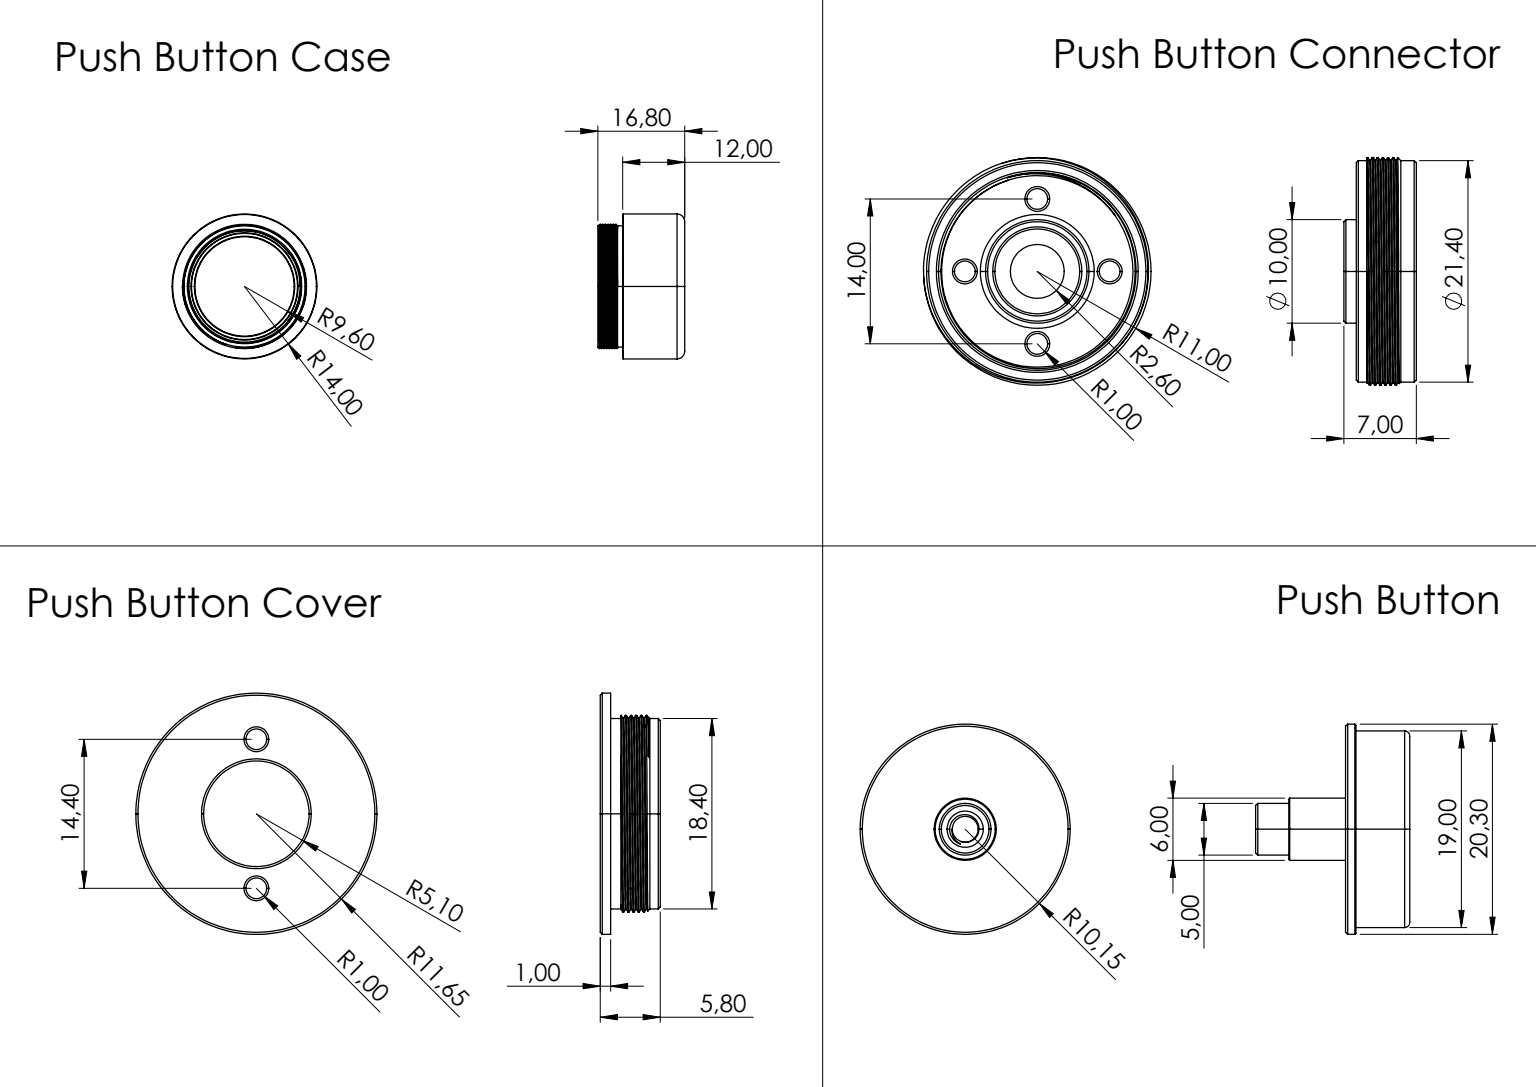
ISO-10303-21;
HEADER;
FILE_DESCRIPTION (('STEP AP214'),
    '1' );
FILE_NAME ('Push Button Case.step',
    '2026-10-07T19:06:49',
    ( '' ),
    ( '' ),
    'SwSTEP 2.0',
    'SolidWorks 2020',
    '' );
FILE_SCHEMA (( 'AUTOMOTIVE_DESIGN' ));
ENDSEC;

DATA;
#16=CARTESIAN_POINT ( 'NONE',  ( 3.109033293168000256, -77.33638120859698972, -11.95479571607999958 ) ) ;
#23=CARTESIAN_POINT ( 'NONE',  ( -2.309466437478999712, -77.64150279751002870, 10.97654204954999990 ) ) ;
#32=AXIS2_PLACEMENT_3D ( 'NONE', #6356, #50954, #38231 ) ;
#33=ADVANCED_FACE ( 'NONE', ( #3684 ), #39982, .F. ) ;
#37=AXIS2_PLACEMENT_3D ( 'NONE', #47276, #15952, #33942 ) ;
#39=CARTESIAN_POINT ( 'NONE',  ( -6.620362748380999918, -76.28137637478999977, -10.34376132320999986 ) ) ;
#46=CARTESIAN_POINT ( 'NONE',  ( 2.813789756862229652, -77.85416666666665719, 10.47020627418440064 ) ) ;
#50=CARTESIAN_POINT ( 'NONE',  ( -10.20076187689604374, -79.12621043184928737, -3.463739626987611064 ) ) ;
#55=CARTESIAN_POINT ( 'NONE',  ( -11.91766194687999914, -78.07234609596400787, 0.6362673702790999641 ) ) ;
#59=CARTESIAN_POINT ( 'NONE',  ( 7.698699457163000304, -79.83930274324279708, 7.739857405570000459 ) ) ;
#68=CARTESIAN_POINT ( 'NONE',  ( 1.570796326794856590, -77.76458333333333428, 12.00000000000000711 ) ) ;
#72=CARTESIAN_POINT ( 'NONE',  ( 6.724228645090999379, -79.38539396382098801, -8.890407735272999545 ) ) ;
#80=ADVANCED_FACE ( 'NONE', ( #13408 ), #31504, .F. ) ;
#87=DIRECTION ( 'NONE',  ( 0.000000000000000000, 1.000000000000000000, 0.000000000000000000 ) ) ;
#96=ORIENTED_EDGE ( 'NONE', *, *, #34117, .T. ) ;
#98=CARTESIAN_POINT ( 'NONE',  ( 6.225574660483999878, -77.96842036916400787, 9.107357164861998200 ) ) ;
#102=CARTESIAN_POINT ( 'NONE',  ( 10.54265532893000135, -78.47604828264000787, 3.830212845596999927 ) ) ;
#103=CARTESIAN_POINT ( 'NONE',  ( 10.87736683009447525, -81.00000000000001421, 1.725104219249947057 ) ) ;
#104=EDGE_LOOP ( 'NONE', ( #8306, #56264, #8122, #44410 ) ) ;
#119=CARTESIAN_POINT ( 'NONE',  ( -10.96659098533000076, -79.41245439073298940, -5.858662427812999951 ) ) ;
#121=CARTESIAN_POINT ( 'NONE',  ( 2.970805461283999804, -76.56305898269899046, 11.10324980701000008 ) ) ;
#122=CARTESIAN_POINT ( 'NONE',  ( -5.476929600924019148, -78.01766025678556105, 9.250714535254271453 ) ) ;
#123=CARTESIAN_POINT ( 'NONE',  ( -4.085659785884999451, -78.53658950733898791, 11.26159174134999930 ) ) ;
#129=CARTESIAN_POINT ( 'NONE',  ( 4.095273378172390899, -80.94411864974023274, 9.939233580224922093 ) ) ;
#132=CARTESIAN_POINT ( 'NONE',  ( 8.145565103785999739, -77.70092985212998826, 7.609492079688000565 ) ) ;
#133=CARTESIAN_POINT ( 'NONE',  ( 11.68767212001977995, -78.07083333333333997, 3.140974612311385972 ) ) ;
#134=CARTESIAN_POINT ( 'NONE',  ( -1.803444444386999912, -80.27907522661350015, 10.99384993464000004 ) ) ;
#140=CARTESIAN_POINT ( 'NONE',  ( 0.2654799511899000319, -78.39298939775198960, -11.21373274707999990 ) ) ;
#150=CARTESIAN_POINT ( 'NONE',  ( 0.1384068119873999858, -77.08287542851299179, 11.14609546546000018 ) ) ;
#159=CARTESIAN_POINT ( 'NONE',  ( 10.58961540942159729, -78.57316667069575544, -3.698874623828772634 ) ) ;
#164=CARTESIAN_POINT ( 'NONE',  ( -0.4120475804594999625, -79.51319421340399174, -11.13933648663000042 ) ) ;
#183=CARTESIAN_POINT ( 'NONE',  ( 4.145485675599949182, -78.25643109645689321, -9.984513293680489454 ) ) ;
#185=VERTEX_POINT ( 'NONE', #55030 ) ;
#196=CARTESIAN_POINT ( 'NONE',  ( -7.859650249856000137, -76.58738468523199572, -7.529696512734999736 ) ) ;
#197=CARTESIAN_POINT ( 'NONE',  ( 12.00000000000000000, -78.14999999999999147, 0.000000000000000000 ) ) ;
#200=CARTESIAN_POINT ( 'NONE',  ( -11.26045488449999965, -80.83153675553073469, 0.3336940576009999604 ) ) ;
#207=CARTESIAN_POINT ( 'NONE',  ( 8.440675369999999234, -80.13928997744719140, 7.053722371789000967 ) ) ;
#219=ORIENTED_EDGE ( 'NONE', *, *, #4233, .T. ) ;
#230=CARTESIAN_POINT ( 'NONE',  ( 0.2080084001491119827, -77.22664242507777033, -10.74806830262927981 ) ) ;
#238=CARTESIAN_POINT ( 'NONE',  ( -0.7898276719169999849, -78.74313915747200099, -11.90847071177000061 ) ) ;
#242=CARTESIAN_POINT ( 'NONE',  ( 9.597438627498371844, -76.59723940367341299, -7.375897342311914073 ) ) ;
#263=CARTESIAN_POINT ( 'NONE',  ( -1.879551087701830880, -76.29218749999812133, 11.88134584529343485 ) ) ;
#275=CARTESIAN_POINT ( 'NONE',  ( 2.269106295766999856E-14, -92.56607767729998670, -10.93038838648999977 ) ) ;
#277=CARTESIAN_POINT ( 'NONE',  ( 5.013494814495999208, -77.86362032395699373, 9.697434492446999954 ) ) ;
#278=CARTESIAN_POINT ( 'NONE',  ( 12.18149635271999820, -78.11332874153899297, -1.551427017228999894 ) ) ;
#286=CARTESIAN_POINT ( 'NONE',  ( -4.648821459404000045, -81.05100055871760389, 9.896537447400001852 ) ) ;
#289=CARTESIAN_POINT ( 'NONE',  ( 7.508079800428999917, -77.01725177193199556, -8.333477563431999968 ) ) ;
#305=ORIENTED_EDGE ( 'NONE', *, *, #4247, .T. ) ;
#307=ORIENTED_EDGE ( 'NONE', *, *, #4039, .F. ) ;
#314=CARTESIAN_POINT ( 'NONE',  ( 1.293235748077000036, -76.48998211639099054, 12.16612483867000094 ) ) ;
#315=CARTESIAN_POINT ( 'NONE',  ( -10.47027344149396377, -78.61824586144523153, -2.436629557234976762 ) ) ;
#321=CARTESIAN_POINT ( 'NONE',  ( -1.570796326794885012, -78.91458333333333997, -12.00000000000000178 ) ) ;
#334=DIRECTION ( 'NONE',  ( 0.000000000000000000, 1.000000000000000000, 1.686839199259000058E-13 ) ) ;
#335=ADVANCED_FACE ( 'NONE', ( #15362 ), #37204, .T. ) ;
#341=ORIENTED_EDGE ( 'NONE', *, *, #14163, .T. ) ;
#351=CARTESIAN_POINT ( 'NONE',  ( -1.612912635236000147, -78.84554001676799828, 10.91330597072999886 ) ) ;
#353=VERTEX_POINT ( 'NONE', #51103 ) ;
#360=CARTESIAN_POINT ( 'NONE',  ( -3.140974612311405512, -77.79583333333334849, 11.68767212001977640 ) ) ;
#364=CARTESIAN_POINT ( 'NONE',  ( -9.018305195942000196, -79.72548445825199792, 6.745675351750000104 ) ) ;
#374=CARTESIAN_POINT ( 'NONE',  ( -5.413904038987206846, -78.41666666666665719, 9.393203674808249914 ) ) ;
#381=CARTESIAN_POINT ( 'NONE',  ( -3.140974612311405512, -79.69583333333332575, 11.68767212001977640 ) ) ;
#382=EDGE_LOOP ( 'NONE', ( #44129, #54601, #18071, #20029, #55022, #27124, #7591, #40469, #14418, #38243, #20068 ) ) ;
#383=CARTESIAN_POINT ( 'NONE',  ( 8.628867348358941314, -76.05332450398152844, 6.837351357443815836 ) ) ;
#386=AXIS2_PLACEMENT_3D ( 'NONE', #45632, #45042, #41184 ) ;
#387=CARTESIAN_POINT ( 'NONE',  ( 11.00720109383000000, -77.39645716612599813, 0.7370606905150999255 ) ) ;
#391=CARTESIAN_POINT ( 'NONE',  ( 1.099819419251000019, -79.63329055598900652, 11.16281809564999961 ) ) ;
#411=CARTESIAN_POINT ( 'NONE',  ( -12.01465389393999850, -78.95880199243299558, -2.711845028153999859 ) ) ;
#412=CARTESIAN_POINT ( 'NONE',  ( -10.26547038271000112, -76.61176894222799660, 3.946724975948999958 ) ) ;
#413=CARTESIAN_POINT ( 'NONE',  ( -6.822290318485905836, -78.02980255133013543, 8.307683877974495701 ) ) ;
#414=CARTESIAN_POINT ( 'NONE',  ( 8.770451247185000909, -78.94352923869598726, 8.160602927202999624 ) ) ;
#419=CARTESIAN_POINT ( 'NONE',  ( 6.307978547608708020, -80.92535043715515997, 8.704505370279399301 ) ) ;
#421=DIRECTION ( 'NONE',  ( -0.7071067811864976127, 0.7071067811865975328, -1.591673720108993631E-09 ) ) ;
#422=CARTESIAN_POINT ( 'NONE',  ( -10.52129323452999898, -77.86434791014099233, 3.681981700656000278 ) ) ;
#424=CARTESIAN_POINT ( 'NONE',  ( -11.00676540241999923, -80.45419303504098707, 0.6467430135644000044 ) ) ;
#431=CARTESIAN_POINT ( 'NONE',  ( 9.070694317316998934, -77.99836472845399271, 6.598531290616000078 ) ) ;
#436=CARTESIAN_POINT ( 'NONE',  ( -10.65295200446612967, -78.51231955895573833, -1.664190318615639042 ) ) ;
#439=CARTESIAN_POINT ( 'NONE',  ( -4.801183948719927486, -76.05000000000001137, 10.79468190462868016 ) ) ;
#441=CARTESIAN_POINT ( 'NONE',  ( -3.610459473067000324, -77.11011177151499396, 10.54605058607999979 ) ) ;
#447=CARTESIAN_POINT ( 'NONE',  ( -7.579570500035162972, -80.16319179611589618, -7.622759937838323729 ) ) ;
#451=DIRECTION ( 'NONE',  ( 0.000000000000000000, 1.000000000000000000, 0.000000000000000000 ) ) ;
#452=CARTESIAN_POINT ( 'NONE',  ( 0.9518616847512999524, -79.02294003937198852, -11.10623968335000100 ) ) ;
#472=CARTESIAN_POINT ( 'NONE',  ( 10.75000000000000000, -78.25000000000000000, 1.005550720961999908E-14 ) ) ;
#483=CARTESIAN_POINT ( 'NONE',  ( 9.755626371838998168, -80.97443200427989041, -5.633583086437000453 ) ) ;
#489=CARTESIAN_POINT ( 'NONE',  ( 7.551392188974999975, -80.21711109272469287, 8.117862728809001283 ) ) ;
#493=CARTESIAN_POINT ( 'NONE',  ( -10.75000000000000000, -80.00000000000000000, 0.000000000000000000 ) ) ;
#502=CARTESIAN_POINT ( 'NONE',  ( -6.340838181001343443, -79.52523374718921900, 8.680779125499762827 ) ) ;
#516=CARTESIAN_POINT ( 'NONE',  ( 0.01050698433460529012, -77.22515890467916222, -10.74994752102681339 ) ) ;
#520=ORIENTED_EDGE ( 'NONE', *, *, #57168, .F. ) ;
#524=CARTESIAN_POINT ( 'NONE',  ( 6.436424241555000592, -80.32391735373440156, 8.610165096135999008 ) ) ;
#526=CARTESIAN_POINT ( 'NONE',  ( 11.27339212957999948, -77.96985744374799765, 4.255161755617000274 ) ) ;
#533=FACE_OUTER_BOUND ( 'NONE', #5641, .T. ) ;
#534=CIRCLE ( 'NONE', #25023, 12.09999999999999964 ) ;
#543=CARTESIAN_POINT ( 'NONE',  ( -11.08400893143999966, -76.20894737471998326, -1.489506537590000068 ) ) ;
#546=CARTESIAN_POINT ( 'NONE',  ( -11.92766985523999956, -77.65742819841213418, -1.116582401450000095 ) ) ;
#548=CARTESIAN_POINT ( 'NONE',  ( -6.660059710594288696, -76.92432036743132073, -9.025807911732075084 ) ) ;
#562=CARTESIAN_POINT ( 'NONE',  ( -0.2428088493965334382, -78.22329368912637904, -10.77973457647781785 ) ) ;
#563=EDGE_CURVE ( 'NONE', #20195, #7399, #29212, .T. ) ;
#569=CARTESIAN_POINT ( 'NONE',  ( 1.764045786578000152, -77.01006991430598703, -11.99279291753999921 ) ) ;
#578=CARTESIAN_POINT ( 'NONE',  ( -7.249076177254000442, -80.50531345225510904, 8.347662706485998285 ) ) ;
#579=CARTESIAN_POINT ( 'NONE',  ( -9.599999999999999645, -90.39999999999999147, 0.000000000000000000 ) ) ;
#581=CYLINDRICAL_SURFACE ( 'NONE', #57781, 12.00000000000000000 ) ;
#610=CARTESIAN_POINT ( 'NONE',  ( -10.75000000000000000, -76.50000000000000000, 0.000000000000000000 ) ) ;
#616=VERTEX_POINT ( 'NONE', #44246 ) ;
#624=CARTESIAN_POINT ( 'NONE',  ( 2.548493721447000038, -77.06004840258400179, 12.01365081398999912 ) ) ;
#635=CARTESIAN_POINT ( 'NONE',  ( 11.20799393363000007, -77.77703814603999888, 4.230477091134000389 ) ) ;
#637=CARTESIAN_POINT ( 'NONE',  ( 4.928445265185000146, -78.16739492409399759, -10.99573548889999941 ) ) ;
#640=CARTESIAN_POINT ( 'NONE',  ( -10.57985553746999940, -78.98172173177698596, -3.125442558719000008 ) ) ;
#642=ORIENTED_EDGE ( 'NONE', *, *, #17291, .F. ) ;
#646=CARTESIAN_POINT ( 'NONE',  ( -14.00000000000000000, -80.89999999999999147, 0.000000000000000000 ) ) ;
#647=CARTESIAN_POINT ( 'NONE',  ( -7.374560639699019760, -77.82708333333329165, 9.596002108778129980 ) ) ;
#652=CARTESIAN_POINT ( 'NONE',  ( 10.16136252780999882, -79.56206640024099386, 4.855993836148999598 ) ) ;
#654=CARTESIAN_POINT ( 'NONE',  ( 9.393203674808260573, -79.79166666666665719, 5.413904038987188194 ) ) ;
#671=CARTESIAN_POINT ( 'NONE',  ( 7.605248831740031967, -78.78754124960966010, -7.597529869121465218 ) ) ;
#672=CARTESIAN_POINT ( 'NONE',  ( -12.00000000000000000, -79.79999999999999716, 6.639246269807000381E-13 ) ) ;
#679=CARTESIAN_POINT ( 'NONE',  ( -6.549634241348975650, -76.96947804690607597, 10.29244451497932467 ) ) ;
#680=CARTESIAN_POINT ( 'NONE',  ( 6.917883603915965907, -78.72389193389439299, -9.780740130690492862 ) ) ;
#681=CARTESIAN_POINT ( 'NONE',  ( 10.93160348586000019, -79.03409100994899461, 2.513594203403000105 ) ) ;
#682=CARTESIAN_POINT ( 'NONE',  ( 10.14177821597014173, -81.00000000000002842, 4.213176577505078235 ) ) ;
#692=CARTESIAN_POINT ( 'NONE',  ( -10.75000000000000000, -81.00000000000000000, 2.851355842494999902E-13 ) ) ;
#694=DIRECTION ( 'NONE',  ( 0.000000000000000000, -1.000000000000000000, 0.000000000000000000 ) ) ;
#700=CARTESIAN_POINT ( 'NONE',  ( -12.29903597714999997, -79.44542282429898705, -0.6631160193374000533 ) ) ;
#701=CARTESIAN_POINT ( 'NONE',  ( -3.222839321634999976, -76.53899580226399735, 10.90918487679000037 ) ) ;
#702=CARTESIAN_POINT ( 'NONE',  ( 1.078297123321654505, -77.96723831660007420, 10.71709050783147710 ) ) ;
#703=CARTESIAN_POINT ( 'NONE',  ( -8.885616033064000163, -78.07539114513500067, 8.035041515002001589 ) ) ;
#706=AXIS2_PLACEMENT_3D ( 'NONE', #56290, #17001, #47739 ) ;
#709=CARTESIAN_POINT ( 'NONE',  ( 8.032001238464035353, -80.90813382219710093, 7.145123807818250405 ) ) ;
#712=CARTESIAN_POINT ( 'NONE',  ( -11.10013370946000144, -76.88383956207499637, 1.020686637641000205 ) ) ;
#713=CARTESIAN_POINT ( 'NONE',  ( -0.6669403506045999963, -76.27067270026404344, -12.26286337364000012 ) ) ;
#718=CARTESIAN_POINT ( 'NONE',  ( 1.633411169670999863, -77.83494667044399762, -11.09730050697999992 ) ) ;
#740=CARTESIAN_POINT ( 'NONE',  ( -0.2300833467695000134, -78.44680123892500490, -11.11357981391999949 ) ) ;
#744=EDGE_CURVE ( 'NONE', #35616, #18221, #56482, .T. ) ;
#754=CARTESIAN_POINT ( 'NONE',  ( 10.75000000000000355, -78.23958333333330017, -1.407171709420407035 ) ) ;
#756=EDGE_CURVE ( 'NONE', #5144, #34885, #31774, .T. ) ;
#758=ORIENTED_EDGE ( 'NONE', *, *, #11996, .T. ) ;
#772=CARTESIAN_POINT ( 'NONE',  ( -9.578166812159000898, -80.15420130091290218, 5.930253639820000089 ) ) ;
#775=CARTESIAN_POINT ( 'NONE',  ( 9.494399870356199145, -76.17369791634894227, -7.297544775540704798 ) ) ;
#786=CARTESIAN_POINT ( 'NONE',  ( -9.038474301085981821, -79.55454762255861567, 5.819977710880431587 ) ) ;
#801=CARTESIAN_POINT ( 'NONE',  ( -6.221842943951165772, -77.17604202210270614, -8.766351684138484757 ) ) ;
#811=CARTESIAN_POINT ( 'NONE',  ( 7.527227981725999939, -78.51244375222299254, 9.409389490551998136 ) ) ;
#816=CARTESIAN_POINT ( 'NONE',  ( -11.68619273497913014, -76.42035715448702149, -3.140303762288782163 ) ) ;
#823=CARTESIAN_POINT ( 'NONE',  ( 0.000000000000000000, -76.00000000000000000, 0.000000000000000000 ) ) ;
#828=CONICAL_SURFACE ( 'NONE', #33783, 10.96250000000000036, 0.7853981633972997312 ) ;
#829=CARTESIAN_POINT ( 'NONE',  ( -4.800187936532999800, -76.10861960676400884, 10.10109298474000106 ) ) ;
#830=CARTESIAN_POINT ( 'NONE',  ( 0.000000000000000000, -92.79999999999999716, 0.000000000000000000 ) ) ;
#846=CARTESIAN_POINT ( 'NONE',  ( 2.264809212410999647E-14, -92.79999999999999716, 0.000000000000000000 ) ) ;
#852=CARTESIAN_POINT ( 'NONE',  ( 11.48873525783000105, -77.65213037933499152, 4.336443399433000501 ) ) ;
#860=CARTESIAN_POINT ( 'NONE',  ( -6.095058532100999571, -81.19811224954469253, 9.210169058603000281 ) ) ;
#865=CARTESIAN_POINT ( 'NONE',  ( 11.75000000000000000, -79.80000000000002558, -1.240340237986687466 ) ) ;
#877=CARTESIAN_POINT ( 'NONE',  ( 11.26957934775000147, -79.10909624325299205, 4.877733875464000057 ) ) ;
#885=ORIENTED_EDGE ( 'NONE', *, *, #57938, .F. ) ;
#886=CARTESIAN_POINT ( 'NONE',  ( 5.438910196678000020, -76.28506842486599737, -10.95925680354000065 ) ) ;
#909=FACE_OUTER_BOUND ( 'NONE', #1382, .T. ) ;
#914=CARTESIAN_POINT ( 'NONE',  ( -2.848564863371000122, -78.85456761274453186, -10.84913769894000168 ) ) ;
#918=DIRECTION ( 'NONE',  ( 1.558073931336000057E-11, -1.000000000000000000, 1.336740861260999965E-10 ) ) ;
#919=CIRCLE ( 'NONE', #14073, 10.25000000000000000 ) ;
#924=CARTESIAN_POINT ( 'NONE',  ( -4.771559678803999560, -78.60146397087400771, -11.06471824780000013 ) ) ;
#927=CARTESIAN_POINT ( 'NONE',  ( 10.41480047653000085, -78.68212195875699422, -3.637813056042999982 ) ) ;
#939=CARTESIAN_POINT ( 'NONE',  ( -3.994755123096000560, -79.11303053380299843, 10.40656197200999955 ) ) ;
#941=CARTESIAN_POINT ( 'NONE',  ( -3.037998163973060883, -79.44541822414515764, 11.43917581953734697 ) ) ;
#957=CARTESIAN_POINT ( 'NONE',  ( 7.478737840490471633, -78.78621029007136656, -7.724116019082565288 ) ) ;
#958=CIRCLE ( 'NONE', #32, 10.25000000000000000 ) ;
#965=CARTESIAN_POINT ( 'NONE',  ( -9.690759288037638086, -78.09991767914834782, -7.043378150385348313 ) ) ;
#966=CARTESIAN_POINT ( 'NONE',  ( 2.407803015296000382, -80.19133328329790800, 10.73324203768999929 ) ) ;
#967=CARTESIAN_POINT ( 'NONE',  ( 4.500641208133613347, -81.00000000000001421, 9.880214559888472081 ) ) ;
#968=ORIENTED_EDGE ( 'NONE', *, *, #8365, .F. ) ;
#973=CARTESIAN_POINT ( 'NONE',  ( 9.576266942756152645, -76.04999999999998295, 5.533717098124343536 ) ) ;
#977=CARTESIAN_POINT ( 'NONE',  ( 1.570796326794910547, -78.53541666666664867, -11.99999999999999822 ) ) ;
#987=CARTESIAN_POINT ( 'NONE',  ( -8.615867236575999399, -76.71811381506900318, 7.785367480540000606 ) ) ;
#989=CARTESIAN_POINT ( 'NONE',  ( -11.86109855473999986, -78.57731821575799813, -1.682380905046999997 ) ) ;
#993=CARTESIAN_POINT ( 'NONE',  ( 1.544981608555010544, -80.96391980284444401, 10.63828215852447023 ) ) ;
#996=CARTESIAN_POINT ( 'NONE',  ( 10.69210609810000001, -78.16394768316000352, 3.151740433137000252 ) ) ;
#998=CARTESIAN_POINT ( 'NONE',  ( 8.209261416751999718, -80.19853216860269640, 7.218337095169999884 ) ) ;
#1003=CARTESIAN_POINT ( 'NONE',  ( -6.984027423104000043, -77.12680175239600544, 8.777327129872999123 ) ) ;
#1014=EDGE_CURVE ( 'NONE', #4724, #21904, #41618, .T. ) ;
#1017=CARTESIAN_POINT ( 'NONE',  ( 8.229676506584999274, -77.58638398095499156, 7.688067972860000765 ) ) ;
#1020=CARTESIAN_POINT ( 'NONE',  ( -9.596002108778161954, -79.35208333333332575, -7.374560639698982456 ) ) ;
#1023=CARTESIAN_POINT ( 'NONE',  ( -5.970525758963701080, -80.17821961223123139, -8.939477884329102508 ) ) ;
#1028=CARTESIAN_POINT ( 'NONE',  ( -10.27879708628000088, -78.85952198136099867, 4.312879667924000238 ) ) ;
#1042=VERTEX_POINT ( 'NONE', #55012 ) ;
#1056=CARTESIAN_POINT ( 'NONE',  ( 11.02326530841000007, -81.02459481428599020, 1.187788371667000131 ) ) ;
#1058=CYLINDRICAL_SURFACE ( 'NONE', #386, 12.00000000000000000 ) ;
#1059=CARTESIAN_POINT ( 'NONE',  ( 3.098607378237295595, -76.14114583267888747, -11.53327867144136043 ) ) ;
#1070=FACE_BOUND ( 'NONE', #30736, .T. ) ;
#1074=CARTESIAN_POINT ( 'NONE',  ( 7.189755216797094839, -79.41669502080303289, 7.992951545765084376 ) ) ;
#1086=CARTESIAN_POINT ( 'NONE',  ( 12.00000000000000000, -76.64999999999999147, 0.000000000000000000 ) ) ;
#1089=CARTESIAN_POINT ( 'NONE',  ( -10.75033332359620708, -77.11068282368783855, -1.411355356088692670 ) ) ;
#1095=CARTESIAN_POINT ( 'NONE',  ( 6.536979956083999177, -79.30461158636299501, -10.09826910480999906 ) ) ;
#1097=DIRECTION ( 'NONE',  ( 0.000000000000000000, -1.000000000000000000, 0.000000000000000000 ) ) ;
#1099=CARTESIAN_POINT ( 'NONE',  ( 11.66178877871000097, -78.39045805696299851, 2.537357863477000208 ) ) ;
#1110=CARTESIAN_POINT ( 'NONE',  ( -10.75000000000000000, -80.50000000000000000, -1.711887504597999906E-14 ) ) ;
#1114=CARTESIAN_POINT ( 'NONE',  ( 9.776276929627000456, -75.90796407085099418, -5.431214116490000521 ) ) ;
#1145=CARTESIAN_POINT ( 'NONE',  ( -10.20620196243999978, -80.81341270350478112, -5.091275341613999750 ) ) ;
#1150=CARTESIAN_POINT ( 'NONE',  ( 10.79417609527999922, -77.62976718524500086, -3.050225076229999832 ) ) ;
#1155=CARTESIAN_POINT ( 'NONE',  ( 1.147008568205678536, -76.09166666666237688, 10.95833333328629067 ) ) ;
#1156=ORIENTED_EDGE ( 'NONE', *, *, #53762, .F. ) ;
#1159=CARTESIAN_POINT ( 'NONE',  ( 0.000000000000000000, -87.64999999984398471, 0.000000000000000000 ) ) ;
#1164=CARTESIAN_POINT ( 'NONE',  ( 2.263099670254000273, -78.11897245443199722, 11.95244370277000101 ) ) ;
#1173=VERTEX_POINT ( 'NONE', #7578 ) ;
#1175=CARTESIAN_POINT ( 'NONE',  ( 8.586577278446998918, -79.87637572403669139, 6.741381070085999738 ) ) ;
#1182=CARTESIAN_POINT ( 'NONE',  ( -10.31421052434999908, -76.72175206120299151, 3.823226550887000030 ) ) ;
#1188=CARTESIAN_POINT ( 'NONE',  ( -10.75000000000000000, -77.51041666666665719, -1.407171709420429018 ) ) ;
#1193=CARTESIAN_POINT ( 'NONE',  ( 10.16964605767000052, -76.26874748315199781, -6.884832982024000181 ) ) ;
#1197=CARTESIAN_POINT ( 'NONE',  ( -6.324515969367999979, -78.82733126974268600, -9.263833350438000380 ) ) ;
#1206=CARTESIAN_POINT ( 'NONE',  ( 10.75624577990000041, -78.22165355494099970, -5.431293436759999871 ) ) ;
#1219=CARTESIAN_POINT ( 'NONE',  ( 6.758989304250999197, -77.04505930305400341, -10.14916591256000089 ) ) ;
#1226=CARTESIAN_POINT ( 'NONE',  ( -11.77076513002849012, -79.55082450634814961, -0.1443961957164959509 ) ) ;
#1235=CARTESIAN_POINT ( 'NONE',  ( 9.393203674808260573, -79.29166666666665719, 5.413904038987188194 ) ) ;
#1241=CARTESIAN_POINT ( 'NONE',  ( 6.122270975308672369, -78.77338805014832701, -8.836258741097333669 ) ) ;
#1247=EDGE_CURVE ( 'NONE', #50686, #10829, #57163, .T. ) ;
#1250=CARTESIAN_POINT ( 'NONE',  ( 8.049776716670494991, -77.23386658315779130, -8.806146062382781636 ) ) ;
#1252=CARTESIAN_POINT ( 'NONE',  ( -7.301194973305000779, -79.19750906795999867, 8.515319286630999684 ) ) ;
#1269=ORIENTED_EDGE ( 'NONE', *, *, #11855, .T. ) ;
#1270=CARTESIAN_POINT ( 'NONE',  ( -3.140974612311352221, -79.50416666666664867, -11.68767212001979061 ) ) ;
#1272=CARTESIAN_POINT ( 'NONE',  ( 3.165837231865861856, -77.95154321140272202, 10.30965284180923724 ) ) ;
#1276=CARTESIAN_POINT ( 'NONE',  ( 10.45256899451774757, -80.86916725350319268, 2.510129016786621925 ) ) ;
#1279=CARTESIAN_POINT ( 'NONE',  ( -3.573177736666999671, -77.36011177151499396, 10.43715168250999881 ) ) ;
#1280=CARTESIAN_POINT ( 'NONE',  ( 2.548493721447000038, -77.00836198975264324, 12.01365081398999912 ) ) ;
#1281=CARTESIAN_POINT ( 'NONE',  ( -6.382578252665999763, -80.53473609305189029, -8.990542599477999275 ) ) ;
#1282=ORIENTED_EDGE ( 'NONE', *, *, #26492, .F. ) ;
#1285=CARTESIAN_POINT ( 'NONE',  ( -7.712695008784000272, -77.26298346740499312, -8.144473358846001432 ) ) ;
#1300=CARTESIAN_POINT ( 'NONE',  ( -7.374560639698971798, -79.37291666666664014, -9.596002108778163731 ) ) ;
#1303=CARTESIAN_POINT ( 'NONE',  ( -7.600460745173878152, -80.16297109611984695, -7.601925197388003319 ) ) ;
#1307=ORIENTED_EDGE ( 'NONE', *, *, #22440, .T. ) ;
#1311=CARTESIAN_POINT ( 'NONE',  ( -5.305451056584999492, -80.04393910884809316, -9.672327717035999584 ) ) ;
#1334=CARTESIAN_POINT ( 'NONE',  ( -12.00000000000000000, -76.89999999999999147, 0.000000000000000000 ) ) ;
#1342=CARTESIAN_POINT ( 'NONE',  ( 8.440675369999999234, -80.07150142417098948, 7.053722371789000967 ) ) ;
#1343=LINE ( 'NONE', #46804, #52543 ) ;
#1344=CARTESIAN_POINT ( 'NONE',  ( 5.413936244485441307, -76.76681587759365755, -9.393431973814015734 ) ) ;
#1356=CARTESIAN_POINT ( 'NONE',  ( 10.07201971379686967, -79.37863564844947462, 3.781752685250035828 ) ) ;
#1369=CARTESIAN_POINT ( 'NONE',  ( -6.271765859646529329, -77.17558322877896160, -8.730771744879000096 ) ) ;
#1371=ADVANCED_FACE ( 'NONE', ( #22609 ), #37635, .F. ) ;
#1374=CARTESIAN_POINT ( 'NONE',  ( 2.377756013412999803, -79.34251650879200213, -11.79209151100000064 ) ) ;
#1379=B_SPLINE_CURVE_WITH_KNOTS ( 'NONE', 3,
 ( #54929, #32472, #36631, #36336, #46687, #49939, #54361, #10071, #37209, #28052, #41359, #5340, #36918, #27471, #654, #51107, #41940, #10659 ),
 .UNSPECIFIED., .F., .F.,
 ( 4, 2, 2, 2, 2, 2, 2, 2, 4 ),
 ( 0.000000000000000000, 0.1250000000000000000, 0.2500000000000000000, 0.3750000000000000000, 0.5000000000000000000, 0.6250000000000000000, 0.7500000000000000000, 0.8750000000000000000, 1.000000000000000000 ),
 .UNSPECIFIED. ) ;
#1380=CARTESIAN_POINT ( 'NONE',  ( 10.65351345285000129, -78.33619942611500164, -5.379419444189999844 ) ) ;
#1382=EDGE_LOOP ( 'NONE', ( #1591, #17664, #4339, #1641 ) ) ;
#1393=CARTESIAN_POINT ( 'NONE',  ( -10.75000000000000000, -80.51041666666664298, -1.407171709420429018 ) ) ;
#1395=CARTESIAN_POINT ( 'NONE',  ( -2.170944906844886724, -79.79999999999999716, -11.61767828058813024 ) ) ;
#1396=DIRECTION ( 'NONE',  ( 0.000000000000000000, 1.000000000000000000, 0.000000000000000000 ) ) ;
#1399=CARTESIAN_POINT ( 'NONE',  ( 11.09875712452000052, -76.02591650810499857, 1.375294608629999971 ) ) ;
#1429=CARTESIAN_POINT ( 'NONE',  ( 10.68616709762000028, -77.08241475543599108, -6.049920594266999352 ) ) ;
#1435=CARTESIAN_POINT ( 'NONE',  ( -9.360432184603999062, -80.25606803504099673, -6.310659218800999781 ) ) ;
#1438=CARTESIAN_POINT ( 'NONE',  ( 5.151324428776999476, -77.73871255725200058, 9.964033682248000900 ) ) ;
#1444=ORIENTED_EDGE ( 'NONE', *, *, #36214, .F. ) ;
#1452=CARTESIAN_POINT ( 'NONE',  ( -0.08650930969203998733, -78.63442944748399555, 12.16449944406000050 ) ) ;
#1457=ORIENTED_EDGE ( 'NONE', *, *, #20680, .F. ) ;
#1467=CARTESIAN_POINT ( 'NONE',  ( 4.763443004301499251, -80.76150222777162924, -9.661361922714023720 ) ) ;
#1481=CARTESIAN_POINT ( 'NONE',  ( -3.699256142337000064, -76.96545403433599120, 11.71059914860999918 ) ) ;
#1485=FACE_OUTER_BOUND ( 'NONE', #53120, .T. ) ;
#1488=DIRECTION ( 'NONE',  ( 0.000000000000000000, 0.000000000000000000, -1.000000000000000000 ) ) ;
#1493=CARTESIAN_POINT ( 'NONE',  ( -10.32936100969000037, -78.46581739375498898, 6.204842689816000068 ) ) ;
#1497=CARTESIAN_POINT ( 'NONE',  ( -10.76888293467999880, -79.53970297022300429, -1.790677617362999907 ) ) ;
#1508=EDGE_LOOP ( 'NONE', ( #37769, #21742, #3756, #37883, #53212, #55093 ) ) ;
#1510=CARTESIAN_POINT ( 'NONE',  ( -6.349996674360999904, -78.85392148219399644, -9.301156207373001195 ) ) ;
#1512=CARTESIAN_POINT ( 'NONE',  ( 11.75000000000000000, -79.79999999999999716, -4.009019365174000020E-13 ) ) ;
#1516=CARTESIAN_POINT ( 'NONE',  ( -9.735746418238305111, -79.30854793174478345, 5.571072665431956672 ) ) ;
#1522=CARTESIAN_POINT ( 'NONE',  ( -1.570796326794938524, -77.18541666666666856, 11.99999999999999645 ) ) ;
#1523=VERTEX_POINT ( 'NONE', #42081 ) ;
#1525=FACE_OUTER_BOUND ( 'NONE', #27120, .T. ) ;
#1526=CARTESIAN_POINT ( 'NONE',  ( 7.078252940824787842, -78.78224352234950345, -8.090973445952867493 ) ) ;
#1529=CARTESIAN_POINT ( 'NONE',  ( 5.177752511601999785, -76.58669514303510084, 9.912858493839999952 ) ) ;
#1535=CARTESIAN_POINT ( 'NONE',  ( 3.925131995945446928, -78.39834014880939606, 11.31871592374366031 ) ) ;
#1536=CARTESIAN_POINT ( 'NONE',  ( -9.735611069857000643, -79.22474541096200085, 5.570995215215999607 ) ) ;
#1543=FACE_OUTER_BOUND ( 'NONE', #16314, .T. ) ;
#1546=CARTESIAN_POINT ( 'NONE',  ( -6.043427764450784778, -78.48333333333333428, -10.48543666025109822 ) ) ;
#1553=ORIENTED_EDGE ( 'NONE', *, *, #47173, .F. ) ;
#1556=CARTESIAN_POINT ( 'NONE',  ( 10.44750279757892208, -77.86896311195575038, 2.532177459664171515 ) ) ;
#1557=CARTESIAN_POINT ( 'NONE',  ( -4.743879332790999825, -78.65870616202899157, -11.00053059214000051 ) ) ;
#1561=CARTESIAN_POINT ( 'NONE',  ( 10.56032766684168145, -80.86570825649420158, 2.052053817749484033 ) ) ;
#1564=CARTESIAN_POINT ( 'NONE',  ( 5.176319218327999572, -78.12272937556599572, -9.742045664616000522 ) ) ;
#1566=CARTESIAN_POINT ( 'NONE',  ( 7.215203368301000175, -80.84409233149752083, 8.184401438574999688 ) ) ;
#1570=CARTESIAN_POINT ( 'NONE',  ( 9.329667775425885878, -80.39183487745914647, 5.387493164505086085 ) ) ;
#1571=CARTESIAN_POINT ( 'NONE',  ( -7.712695008784000272, -77.33077202068200506, -8.144473358846001432 ) ) ;
#1580=DIRECTION ( 'NONE',  ( -1.000000000000000000, 0.000000000000000000, 0.000000000000000000 ) ) ;
#1591=ORIENTED_EDGE ( 'NONE', *, *, #32952, .F. ) ;
#1596=CARTESIAN_POINT ( 'NONE',  ( -1.751509483276000090, -80.07117545184989638, -10.89192126806999994 ) ) ;
#1602=ORIENTED_EDGE ( 'NONE', *, *, #43595, .T. ) ;
#1606=SHAPE_DEFINITION_REPRESENTATION ( #29966, #7879 ) ;
#1610=CARTESIAN_POINT ( 'NONE',  ( 10.34999999999999964, -82.00000000000000000, 0.000000000000000000 ) ) ;
#1612=ORIENTED_EDGE ( 'NONE', *, *, #744, .T. ) ;
#1624=CARTESIAN_POINT ( 'NONE',  ( -12.00000000000000000, -77.29999999999999716, 0.000000000000000000 ) ) ;
#1632=CARTESIAN_POINT ( 'NONE',  ( -10.75000000000000000, -76.59999999999999432, 0.000000000000000000 ) ) ;
#1641=ORIENTED_EDGE ( 'NONE', *, *, #1869, .F. ) ;
#1643=B_SPLINE_CURVE_WITH_KNOTS ( 'NONE', 3,
 ( #34375, #34084, #11680, #11964, #12528, #39107, #29655, #47707, #7236, #25241, #29940, #52690, #3108, #7529, #25527, #30236, #48279, #7815, #43844, #3391, #39399, #57408, #16965, #31391, #10665, #22555, #58278, #40566, #33064, #37502, #5921, #51111, #13982, #1516, #26967, #40265, #50817, #28345, #49431, #4257, #28642, #26670, #31093, #39968, #46395, #22254, #19508, #46692, #15069, #9273, #17841, #4553, #44702, #55521, #10360, #49130, #23926, #54446, #35829, #41945, #159, #57982, #13687, #18135, #21956 ),
 .UNSPECIFIED., .F., .F.,
 ( 4, 1, 1, 1, 1, 1, 1, 1, 1, 1, 1, 1, 1, 1, 1, 1, 1, 1, 1, 1, 1, 1, 1, 1, 1, 1, 1, 1, 1, 1, 1, 1, 1, 1, 1, 1, 1, 1, 1, 1, 1, 1, 1, 1, 1, 1, 1, 1, 1, 1, 1, 1, 1, 1, 1, 1, 1, 1, 1, 1, 1, 1, 4 ),
 ( 0.000000000000000000, 0.01249977918653635833, 0.02874978664248438107, 0.04499979409843239686, 0.06124980155438042306, 0.07749980901032844927, 0.09374981646627647547, 0.1099998239222245017, 0.1262498313781725279, 0.1424998388341205402, 0.1587498462900685803, 0.1749998537460165648, 0.1912498612019646049, 0.2074998686579126173, 0.2237498761138606573, 0.2399998835698086697, 0.2562498910257566265, 0.2724998984817046943, 0.2887499059376527066, 0.3049999133936007190, 0.3212499208495487313, 0.3374999283054967991, 0.3537499357614448114, 0.3699999432173928238, 0.3862499506733408361, 0.4024999581292889039, 0.4187499655852369163, 0.4349999730411849286, 0.4512499804971329409, 0.4674999879530810087, 0.4837499954090290211, 0.5000000028649770334, 0.5162500103209249902, 0.5325000177768730580, 0.5487500252328210149, 0.5650000326887690827, 0.5812500401447171505, 0.5975000476006652184, 0.6137500550566131752, 0.6300000625125612430, 0.6462500699685091998, 0.6625000774244572677, 0.6787500848804052245, 0.6950000923363532923, 0.7112500997923013601, 0.7275001072482493170, 0.7437501147041973848, 0.7600001221601453416, 0.7762501296160934094, 0.7925001370720413663, 0.8087501445279894341, 0.8250001519839373909, 0.8412501594398855698, 0.8575001668958335266, 0.8737501743517815944, 0.8900001818077295512, 0.9062501892636776191, 0.9225001967196255759, 0.9387502041755736437, 0.9550002116315216005, 0.9712502190874696684, 0.9875002265434177362, 1.000000000000000000 ),
 .UNSPECIFIED. ) ;
#1649=CARTESIAN_POINT ( 'NONE',  ( 10.75346375278748745, -79.35200905115739545, 0.2566943562741798579 ) ) ;
#1661=CARTESIAN_POINT ( 'NONE',  ( 10.75000000000000000, -80.34999999999999432, 0.000000000000000000 ) ) ;
#1667=CARTESIAN_POINT ( 'NONE',  ( 7.520016693046000178, -79.81263331077090584, -9.389162645085001202 ) ) ;
#1672=CARTESIAN_POINT ( 'NONE',  ( 2.687462146607000335, -77.76648380221600121, -11.62811462177000088 ) ) ;
#1674=ORIENTED_EDGE ( 'NONE', *, *, #38865, .T. ) ;
#1687=CARTESIAN_POINT ( 'NONE',  ( -10.61294613146216115, -80.08761099959438923, 1.709916667674025392 ) ) ;
#1690=CARTESIAN_POINT ( 'NONE',  ( 9.886069181790999139, -76.40960291063299792, -5.228720670581999741 ) ) ;
#1691=CARTESIAN_POINT ( 'NONE',  ( 9.470019493006097022, -76.39166030756085490, 5.309339906474421333 ) ) ;
#1701=CARTESIAN_POINT ( 'NONE',  ( -9.947467367995102450, -78.06912791544839081, 4.075482521126458479 ) ) ;
#1702=ADVANCED_FACE ( 'NONE', ( #52967 ), #24938, .F. ) ;
#1721=EDGE_LOOP ( 'NONE', ( #52266, #3590, #38822, #18146 ) ) ;
#1724=CARTESIAN_POINT ( 'NONE',  ( -3.103714625783000169, -80.67352195949028726, 10.97518102889000069 ) ) ;
#1727=CARTESIAN_POINT ( 'NONE',  ( -4.531904799951000484, -77.49358547023599897, -10.26060180864999971 ) ) ;
#1732=CARTESIAN_POINT ( 'NONE',  ( 11.00000000000000178, -81.00000000000002842, -0.5732958683357214369 ) ) ;
#1735=CARTESIAN_POINT ( 'NONE',  ( 9.755626371838998168, -80.90664345100368848, -5.633583086437000453 ) ) ;
#1737=ADVANCED_FACE ( 'NONE', ( #2804 ), #31377, .F. ) ;
#1743=CARTESIAN_POINT ( 'NONE',  ( 8.400721904471998513, -78.44452423951798892, -8.798318138657000631 ) ) ;
#1768=CARTESIAN_POINT ( 'NONE',  ( -6.606377239730330864, -77.57291666666665719, -8.596418555780440229 ) ) ;
#1772=CARTESIAN_POINT ( 'NONE',  ( -7.650089724727000551, -76.70538068117299701, -9.607224057717001386 ) ) ;
#1776=CARTESIAN_POINT ( 'NONE',  ( 4.653115705712000505, -78.90904029874850778, -10.20620521156999949 ) ) ;
#1784=CARTESIAN_POINT ( 'NONE',  ( 3.268459929338999981, -78.65572260172200458, -11.59797143510999895 ) ) ;
#1786=AXIS2_PLACEMENT_3D ( 'NONE', #26851, #36596, #14156 ) ;
#1799=CARTESIAN_POINT ( 'NONE',  ( 0.000000000000000000, -75.15999999999999659, 0.000000000000000000 ) ) ;
#1801=CARTESIAN_POINT ( 'NONE',  ( -5.290207344092000774, -78.69050342418300659, 9.942216594703999988 ) ) ;
#1802=CARTESIAN_POINT ( 'NONE',  ( 8.155100784587984819, -76.15986216400646924, 7.653265680561434969 ) ) ;
#1819=CARTESIAN_POINT ( 'NONE',  ( 6.894123566350000232, -77.49915716295998891, -10.09017945751000056 ) ) ;
#1820=CARTESIAN_POINT ( 'NONE',  ( 9.939632792372378844, -78.81897174444549137, -4.094538100961752747 ) ) ;
#1830=CARTESIAN_POINT ( 'NONE',  ( -3.085217259120516697, -78.15417630999539256, -11.57589848832679280 ) ) ;
#1831=CARTESIAN_POINT ( 'NONE',  ( -11.06493808903000087, -79.34700665024199395, -1.839906431680000010 ) ) ;
#1832=ORIENTED_EDGE ( 'NONE', *, *, #17700, .T. ) ;
#1838=CARTESIAN_POINT ( 'NONE',  ( -10.93323770240847814, -78.36784654652733195, -2.507174414007888430 ) ) ;
#1839=EDGE_CURVE ( 'NONE', #54390, #24385, #25400, .T. ) ;
#1853=CARTESIAN_POINT ( 'NONE',  ( -2.102085772900874616, -77.99079252367346271, 10.54238248243097686 ) ) ;
#1854=CARTESIAN_POINT ( 'NONE',  ( 10.99419336675999936, -78.84861136999599296, 4.758540471090999979 ) ) ;
#1856=CARTESIAN_POINT ( 'NONE',  ( -2.814036715996205196, -78.99599336343645462, 10.47066865085466958 ) ) ;
#1861=CARTESIAN_POINT ( 'NONE',  ( -6.868829560331000117, -77.38734811451699613, 8.632549730677999023 ) ) ;
#1862=CARTESIAN_POINT ( 'NONE',  ( 12.24159337356999977, -76.39362091517861586, -0.9828625608234000666 ) ) ;
#1863=CARTESIAN_POINT ( 'NONE',  ( -9.596002108778161954, -78.35208333333332575, -7.374560639698982456 ) ) ;
#1868=CARTESIAN_POINT ( 'NONE',  ( 10.75087127669428000, -80.36060727671831216, 1.407091297144698938 ) ) ;
#1869=EDGE_CURVE ( 'NONE', #14050, #10331, #7738, .T. ) ;
#1870=CARTESIAN_POINT ( 'NONE',  ( 10.75916580684000046, -78.03891693872900248, 3.171507801093999657 ) ) ;
#1882=CARTESIAN_POINT ( 'NONE',  ( 6.459716167540999976, -77.45020226594600388, -9.225293035625000471 ) ) ;
#1892=ORIENTED_EDGE ( 'NONE', *, *, #36548, .T. ) ;
#1894=CARTESIAN_POINT ( 'NONE',  ( 10.46019799182000121, -80.23459350986080096, 3.505129431450999977 ) ) ;
#1912=FACE_OUTER_BOUND ( 'NONE', #13839, .T. ) ;
#1915=CARTESIAN_POINT ( 'NONE',  ( 11.05000000000000071, -81.00000000000000000, 0.000000000000000000 ) ) ;
#1928=CARTESIAN_POINT ( 'NONE',  ( 6.043427764450763462, -77.23333333333330586, 10.48543666025111065 ) ) ;
#1941=EDGE_CURVE ( 'NONE', #51047, #53789, #919, .T. ) ;
#1945=CARTESIAN_POINT ( 'NONE',  ( -1.399903487910991728, -79.48551242492223423, 10.65869450429586962 ) ) ;
#1949=EDGE_CURVE ( 'NONE', #5424, #31838, #47110, .T. ) ;
#1954=EDGE_CURVE ( 'NONE', #4693, #53569, #56526, .T. ) ;
#1959=CARTESIAN_POINT ( 'NONE',  ( 10.70855674592274909, -80.34275261640850374, -1.007396462679471805 ) ) ;
#1960=CARTESIAN_POINT ( 'NONE',  ( -6.227654752595058518, -77.17598872457767811, -8.762225621070838244 ) ) ;
#1962=ORIENTED_EDGE ( 'NONE', *, *, #31274, .F. ) ;
#1964=CARTESIAN_POINT ( 'NONE',  ( 7.313768098873999257, -78.95596922647499127, 9.313141831727000053 ) ) ;
#1965=CARTESIAN_POINT ( 'NONE',  ( -5.051502324002999760E-14, -80.79999999999999716, 0.000000000000000000 ) ) ;
#1969=CARTESIAN_POINT ( 'NONE',  ( -0.08487245167305000615, -78.49897531865799749, 11.93433278878999992 ) ) ;
#1972=VECTOR ( 'NONE', #18173, 1000.000000000000000 ) ;
#1984=CARTESIAN_POINT ( 'NONE',  ( 11.34981816413709055, -79.79999999999996874, 3.212464588891036588 ) ) ;
#1985=ADVANCED_FACE ( 'NONE', ( #13379 ), #26655, .T. ) ;
#1989=CARTESIAN_POINT ( 'NONE',  ( 1.546553306619000256, -76.53772274449399049, -11.07619323537999989 ) ) ;
#1990=CARTESIAN_POINT ( 'NONE',  ( 10.83694732149156081, -76.34642857556234219, -0.6522557621669171635 ) ) ;
#2000=CARTESIAN_POINT ( 'NONE',  ( 4.607226558409000639, -78.92046296702099539, 11.17099812874999998 ) ) ;
#2001=CARTESIAN_POINT ( 'NONE',  ( -8.509317581196993885, -78.04784009799371347, 6.570080670988565075 ) ) ;
#2018=CARTESIAN_POINT ( 'NONE',  ( -8.360726197242001945, -80.08342291261719481, 7.410943183935000178 ) ) ;
#2021=CARTESIAN_POINT ( 'NONE',  ( 3.895497176768000003, -77.24845838321999736, 10.51870773133999926 ) ) ;
#2035=CARTESIAN_POINT ( 'NONE',  ( 6.129172116842999785, -78.09184313900898644, 10.50789130831999962 ) ) ;
#2037=CARTESIAN_POINT ( 'NONE',  ( 3.042547531669000271, -78.64783470746900207, -10.31045122763999977 ) ) ;
#2038=ORIENTED_EDGE ( 'NONE', *, *, #42332, .T. ) ;
#2043=CARTESIAN_POINT ( 'NONE',  ( -6.043427764450832740, -79.71666666666668277, 10.48543666025107512 ) ) ;
#2047=CARTESIAN_POINT ( 'NONE',  ( -7.210617325615999995, -79.14099446298800444, -8.196484842528999337 ) ) ;
#2064=CARTESIAN_POINT ( 'NONE',  ( -12.17466003208999936, -76.62341520456298838, 1.612538369963999907 ) ) ;
#2067=CARTESIAN_POINT ( 'NONE',  ( 3.507155896972999898, -79.09969469976067558, 10.65448112794999957 ) ) ;
#2070=ORIENTED_EDGE ( 'NONE', *, *, #1949, .T. ) ;
#2075=DIRECTION ( 'NONE',  ( 0.000000000000000000, 1.000000000000000000, 0.000000000000000000 ) ) ;
#2077=CARTESIAN_POINT ( 'NONE',  ( 7.966054476048999078, -77.32638614595698812, 9.040893068079999040 ) ) ;
#2081=CARTESIAN_POINT ( 'NONE',  ( -1.596083865962000026, -78.91326708118100441, 10.79943897993000057 ) ) ;
#2094=CARTESIAN_POINT ( 'NONE',  ( 9.414214675708999280, -79.48035737123599631, -6.181142822975999707 ) ) ;
#2095=CARTESIAN_POINT ( 'NONE',  ( -9.831872778489293196, -76.31035381594146827, 5.330330710487904078 ) ) ;
#2096=CARTESIAN_POINT ( 'NONE',  ( 5.000677505783216681, -78.88963964525443373, 10.65720018581769502 ) ) ;
#2104=CARTESIAN_POINT ( 'NONE',  ( 0.000000000000000000, -91.29999999999999716, 0.000000000000000000 ) ) ;
#2105=DIRECTION ( 'NONE',  ( 1.000000000000000000, 0.000000000000000000, 0.000000000000000000 ) ) ;
#2111=CARTESIAN_POINT ( 'NONE',  ( -4.169758043522275415, -78.69350354638132217, -9.910626147760272175 ) ) ;
#2120=CARTESIAN_POINT ( 'NONE',  ( -10.75729140709000120, -78.85675247620899597, -3.177859684493999914 ) ) ;
#2126=CARTESIAN_POINT ( 'NONE',  ( -6.984124517864168880, -77.27839282645433627, 8.777449155807051540 ) ) ;
#2129=CARTESIAN_POINT ( 'NONE',  ( -6.606377239730371720, -80.92708333333332860, 8.596418555780411808 ) ) ;
#2133=CARTESIAN_POINT ( 'NONE',  ( 10.52307592342000042, -79.44025170634557753, 5.828552047478999576 ) ) ;
#2141=CARTESIAN_POINT ( 'NONE',  ( -9.964549960864999889, -77.58706346750800265, 6.650098383618000319 ) ) ;
#2149=CARTESIAN_POINT ( 'NONE',  ( 2.807878695492000087, -78.31338377657900196, 10.66853090226000056 ) ) ;
#2156=CARTESIAN_POINT ( 'NONE',  ( -9.393714757630084122, -80.55838208141010170, 5.413950316515291128 ) ) ;
#2157=CARTESIAN_POINT ( 'NONE',  ( 9.144378690012999300, -77.46695373569099274, -6.496033325431000094 ) ) ;
#2162=CARTESIAN_POINT ( 'NONE',  ( -11.95099068536000075, -76.09110318827499952, -2.203773976563000225 ) ) ;
#2199=DIRECTION ( 'NONE',  ( 0.000000000000000000, -1.000000000000000000, 0.000000000000000000 ) ) ;
#2213=CARTESIAN_POINT ( 'NONE',  ( -10.48543666025111776, -77.35833333333330586, 6.043427764450754580 ) ) ;
#2217=CARTESIAN_POINT ( 'NONE',  ( -3.140974612311405512, -78.29583333333334849, 11.68767212001977640 ) ) ;
#2221=CARTESIAN_POINT ( 'NONE',  ( 10.65295200446612967, -80.26231955895572412, 1.664190318615631270 ) ) ;
#2230=CARTESIAN_POINT ( 'NONE',  ( -0.8350018197176957147, -79.48137498126830280, 10.71907040161639735 ) ) ;
#2236=CARTESIAN_POINT ( 'NONE',  ( 9.706674989537999565, -76.85173030608999056, -5.242346328414999590 ) ) ;
#2243=CARTESIAN_POINT ( 'NONE',  ( 7.892561263457914755, -80.29061954989504102, -7.298914836821083441 ) ) ;
#2244=EDGE_CURVE ( 'NONE', #1173, #5899, #7451, .T. ) ;
#2247=CARTESIAN_POINT ( 'NONE',  ( -11.22206352833000054, -79.59542660325699615, -4.332716936452000844 ) ) ;
#2250=CARTESIAN_POINT ( 'NONE',  ( 10.42985624311000059, -77.41380270170699873, 5.801172517007000096 ) ) ;
#2253=CARTESIAN_POINT ( 'NONE',  ( 9.393203674808260573, -78.79166666666665719, 5.413904038987188194 ) ) ;
#2263=ORIENTED_EDGE ( 'NONE', *, *, #43832, .T. ) ;
#2266=CARTESIAN_POINT ( 'NONE',  ( -3.627345285118236173, -79.79999999999999716, -11.28297148844626641 ) ) ;
#2272=CARTESIAN_POINT ( 'NONE',  ( -10.99972769911000015, -76.38723109256000043, 2.019869862886000345 ) ) ;
#2273=CARTESIAN_POINT ( 'NONE',  ( 9.145904359845623333, -76.30685081006325277, -5.699187237481845969 ) ) ;
#2275=CARTESIAN_POINT ( 'NONE',  ( -1.950974211964999983, -76.50209444038399909, -10.94135830880000171 ) ) ;
#2283=CARTESIAN_POINT ( 'NONE',  ( 2.757516338679999901, -79.71991147651499432, -11.76501219937000009 ) ) ;
#2284=CARTESIAN_POINT ( 'NONE',  ( -8.197392310145165339, -78.04411871163161152, 6.956661028266359459 ) ) ;
#2294=LINE ( 'NONE', #15566, #45221 ) ;
#2301=CARTESIAN_POINT ( 'NONE',  ( 10.71017182930000011, -80.49865852947209532, -3.921716777206999627 ) ) ;
#2304=CARTESIAN_POINT ( 'NONE',  ( -10.93308570624999909, -78.41962113229800480, -2.507139558745000052 ) ) ;
#2321=CARTESIAN_POINT ( 'NONE',  ( 12.16237383090999913, -78.01045519273699824, 0.2432969017631999853 ) ) ;
#2326=CARTESIAN_POINT ( 'NONE',  ( -1.570796326794938524, -79.68541666666668277, 11.99999999999999645 ) ) ;
#2331=CARTESIAN_POINT ( 'NONE',  ( 10.30613478042999986, -78.29666782993099616, -3.599856929194000354 ) ) ;
#2333=CARTESIAN_POINT ( 'NONE',  ( 9.393794433358884532, -80.80838448933172913, -5.414110195013384974 ) ) ;
#2339=VECTOR ( 'NONE', #17547, 1000.000000000000000 ) ;
#2349=CARTESIAN_POINT ( 'NONE',  ( 7.144724566336000393, -76.39169569806699656, 9.988770583665001368 ) ) ;
#2352=CARTESIAN_POINT ( 'NONE',  ( 11.68767212001979594, -78.02916666666668277, -3.140974612311341563 ) ) ;
#2359=CARTESIAN_POINT ( 'NONE',  ( -9.022824479474000015, -77.88263333629100771, 8.159115699504999597 ) ) ;
#2364=CARTESIAN_POINT ( 'NONE',  ( -0.2230286467304000153, -78.64998243216399487, -10.77282081049999896 ) ) ;
#2365=CARTESIAN_POINT ( 'NONE',  ( -10.07999562765293255, -79.57180944839785752, 3.736692566665637205 ) ) ;
#2366=ORIENTED_EDGE ( 'NONE', *, *, #17037, .F. ) ;
#2378=CARTESIAN_POINT ( 'NONE',  ( 8.680500415593000341, -78.58155805217599266, 7.175156920760000112 ) ) ;
#2389=CARTESIAN_POINT ( 'NONE',  ( 6.605943070247981552, -78.42293208188651477, 8.595924706473319077 ) ) ;
#2393=CARTESIAN_POINT ( 'NONE',  ( -12.36265669798000033, -76.74838446013099258, 1.637438600144999867 ) ) ;
#2394=CARTESIAN_POINT ( 'NONE',  ( 0.5871605803710688853, -78.72939686299562823, -10.73511180301259671 ) ) ;
#2399=CARTESIAN_POINT ( 'NONE',  ( -3.463687794021950150, -79.69898096214407701, -10.20052495849528995 ) ) ;
#2401=CARTESIAN_POINT ( 'NONE',  ( 6.060638544127889382, -77.21786737044560311, -10.11814076704347443 ) ) ;
#2402=CARTESIAN_POINT ( 'NONE',  ( 9.453938376997999882, -79.12911590622699975, 6.036651369377000087 ) ) ;
#2410=CARTESIAN_POINT ( 'NONE',  ( 10.34084413924634305, -78.06824677350734021, -4.346096116244792640 ) ) ;
#2424=CARTESIAN_POINT ( 'NONE',  ( -5.413876276891260275, -79.18349062226657509, -9.393307288579276104 ) ) ;
#2425=CARTESIAN_POINT ( 'NONE',  ( 0.9627474882855999727, -78.12971924654898714, -11.94107121277999894 ) ) ;
#2427=CARTESIAN_POINT ( 'NONE',  ( 9.329450859912574501, -78.89181274521322962, 5.387597712135250738 ) ) ;
#2429=CARTESIAN_POINT ( 'NONE',  ( 9.526733066210548273, -80.88851237995341137, 4.980266374315006850 ) ) ;
#2433=CARTESIAN_POINT ( 'NONE',  ( -10.41264997627000000, -77.93207497455300370, 3.643961423121000021 ) ) ;
#2434=CARTESIAN_POINT ( 'NONE',  ( 10.75000000000000000, -79.25000000000000000, 0.000000000000000000 ) ) ;
#2435=CARTESIAN_POINT ( 'NONE',  ( 0.5212087151649998917, -80.89778770350477544, 10.89825343941999947 ) ) ;
#2442=CARTESIAN_POINT ( 'NONE',  ( 9.869466656387999137, -76.97669956165799476, -5.330266269891000164 ) ) ;
#2446=FACE_OUTER_BOUND ( 'NONE', #20407, .T. ) ;
#2452=EDGE_CURVE ( 'NONE', #31055, #49519, #17758, .T. ) ;
#2459=CARTESIAN_POINT ( 'NONE',  ( 0.000000000000000000, -87.20000000000000284, 0.000000000000000000 ) ) ;
#2472=CARTESIAN_POINT ( 'NONE',  ( -8.973625165401864834, -81.00000000000001421, -6.089121955489211757 ) ) ;
#2473=CARTESIAN_POINT ( 'NONE',  ( -5.597547907814000467, -77.65556621773498591, -9.372450235129999641 ) ) ;
#2480=LINE ( 'NONE', #38190, #24417 ) ;
#2481=EDGE_CURVE ( 'NONE', #44663, #23438, #1379, .T. ) ;
#2486=CARTESIAN_POINT ( 'NONE',  ( 1.407171709420440342, -76.63541666666665719, -10.74999999999999822 ) ) ;
#2487=CARTESIAN_POINT ( 'NONE',  ( -12.00000000000000888, -76.88958333333333428, 1.570796326794847264 ) ) ;
#2492=CARTESIAN_POINT ( 'NONE',  ( -1.570796326794937636, -77.28541666666664867, 11.99999999999999467 ) ) ;
#2498=( NAMED_UNIT ( * ) SI_UNIT ( $, .STERADIAN. ) SOLID_ANGLE_UNIT ( ) );
#2501=AXIS2_PLACEMENT_3D ( 'NONE', #15199, #10199, #28179 ) ;
#2510=CARTESIAN_POINT ( 'NONE',  ( -9.329492144256546382, -77.05848916406876015, 5.387603188400559517 ) ) ;
#2518=EDGE_CURVE ( 'NONE', #9803, #34745, #14001, .T. ) ;
#2520=CARTESIAN_POINT ( 'NONE',  ( -2.172168385828000314, -77.81825668956298614, -10.93326506925000174 ) ) ;
#2526=CARTESIAN_POINT ( 'NONE',  ( 9.446529892197220946, -80.31034450011661363, -5.155174753762183926 ) ) ;
#2529=CARTESIAN_POINT ( 'NONE',  ( -3.970056213021999625, -78.96787035545898448, 11.35542513096999961 ) ) ;
#2540=VECTOR ( 'NONE', #37179, 1000.000000000000114 ) ;
#2543=VERTEX_POINT ( 'NONE', #6502 ) ;
#2551=CARTESIAN_POINT ( 'NONE',  ( -11.00477662459603501, -79.80000000000001137, -4.649775713267806587 ) ) ;
#2553=CARTESIAN_POINT ( 'NONE',  ( -10.13847005927290468, -80.07308699731846957, 3.575929410332394642 ) ) ;
#2556=CARTESIAN_POINT ( 'NONE',  ( 11.06808393496999976, -76.66313245443998881, 1.603559079323000125 ) ) ;
#2559=CARTESIAN_POINT ( 'NONE',  ( -7.811514047910000258, -76.82815968624299785, 7.905692513472000194 ) ) ;
#2565=CARTESIAN_POINT ( 'NONE',  ( 9.045277090019000710, -79.20032221108399995, -8.187312926306001160 ) ) ;
#2567=CARTESIAN_POINT ( 'NONE',  ( -10.56344111567097954, -78.08522265697479270, 1.994203520344934644 ) ) ;
#2575=B_SPLINE_CURVE_WITH_KNOTS ( 'NONE', 3,
 ( #11940, #20789, #52668, #39377, #12504, #34924, #47969, #2221, #7213, #25504 ),
 .UNSPECIFIED., .F., .F.,
 ( 4, 2, 2, 2, 4 ),
 ( 0.000000000000000000, 0.2500000000000000000, 0.5000000000000000000, 0.7500000000000000000, 1.000000000000000000 ),
 .UNSPECIFIED. ) ;
#2584=CONICAL_SURFACE ( 'NONE', #12912, 9.649999999909001147, 0.7853981633972997312 ) ;
#2586=DIRECTION ( 'NONE',  ( 0.000000000000000000, 1.000000000000000000, 0.000000000000000000 ) ) ;
#2596=CARTESIAN_POINT ( 'NONE',  ( 4.230954068466677320, -79.94294377347027591, 9.882283910680856209 ) ) ;
#2608=CARTESIAN_POINT ( 'NONE',  ( 4.442094508599000235, -77.41361025341399227, -11.32474889210000057 ) ) ;
#2616=CARTESIAN_POINT ( 'NONE',  ( -6.040190233171999878, -79.49506692201099156, 9.093484917090998820 ) ) ;
#2625=CARTESIAN_POINT ( 'NONE',  ( 9.831723082683108572, -80.55996316945166313, -5.387191927894570576 ) ) ;
#2627=CARTESIAN_POINT ( 'NONE',  ( 11.88382656225999945, -78.38991971485397414, -1.513515996960000276 ) ) ;
#2637=CARTESIAN_POINT ( 'NONE',  ( 11.61133755414000035, -76.77471726614500369, 3.999933378912999604 ) ) ;
#2639=EDGE_CURVE ( 'NONE', #51790, #14050, #28489, .T. ) ;
#2640=CARTESIAN_POINT ( 'NONE',  ( -11.68767212001979061, -77.82083333333333997, -3.140974612311365988 ) ) ;
#2641=ORIENTED_EDGE ( 'NONE', *, *, #31744, .F. ) ;
#2648=CARTESIAN_POINT ( 'NONE',  ( -11.23155942826000064, -77.90976265171399007, 4.672751159098000429 ) ) ;
#2653=CARTESIAN_POINT ( 'NONE',  ( -9.823574345946489927, -79.56680724124903747, 4.374665960120871944 ) ) ;
#2656=CARTESIAN_POINT ( 'NONE',  ( -11.40016033654000083, -79.16505199243299273, 3.876673637571999897 ) ) ;
#2663=CARTESIAN_POINT ( 'NONE',  ( -11.68767212001978706, -77.92083333333333428, -3.140974612311364655 ) ) ;
#2667=CARTESIAN_POINT ( 'NONE',  ( 3.970614904013836988, -79.39750627768901836, 11.12517343397338898 ) ) ;
#2669=B_SPLINE_SURFACE_WITH_KNOTS ( 'NONE', 3, 3, ( 
 ( #15754, #38763, #7476, #24326, #42342, #19902, #25473, #3053, #15469, #21048, #33749, #39050, #57065, #51498, #16625, #34610, #11055, #29037, #47076, #6604, #24616, #42629, #4498, #54093, #44067, #35772, #48787, #8332, #53800, #31628, #17482, #34894, #16914, #21902, #8046, #8921, #4200, #22496, #3337, #57351, #57925, #7763, #31038, #40507, #26911, #43786, #40209, #3616, #30753, #31330, #44646, #49374, #48501, #17782, #13334, #53497, #35469, #49074, #3898, #102, #52923, #26331, #39344, #12757, #25766, #39911, #39625 ),
 ( #44942, #13631, #21331, #18077, #13040, #26043, #36072, #12474, #30475, #8624, #21621, #57633, #22198, #17189, #26610, #35178, #53209, #44345, #58219, #391, #55248, #37522, #28076, #45535, #45829, #37231, #55540, #15091, #19529, #54953, #41671, #49670, #9215, #27493, #1536, #1252, #28367, #54671, #9506, #19239, #14794, #681, #50251, #4786, #27201, #22788, #45239, #46125, #14505, #40797, #32789, #5649, #5080, #10382, #18664, #46413, #9801, #18368, #5943, #36361, #54388, #27784, #23658, #13925, #14212, #31920, #41383 ),
 ( #966, #5365, #23947, #41963, #49965, #23075, #41090, #36652, #32209, #23372, #18949, #36942, #32496, #50543, #10096, #38399, #16264, #2972, #28664, #7394, #33960, #42265, #34243, #51712, #24828, #33385, #56419, #11262, #29243, #7111, #24249, #20119, #1831, #19827, #47290, #52278, #6818, #2695, #43414, #42843, #2402, #51421, #56987, #20971, #46713, #33086, #20403, #51997, #15968, #38109, #2120, #33675, #38976, #6233, #20689, #15678, #11552, #29530, #47586, #43137, #25112, #6527, #38687, #51130, #37819, #11833, #56707 ),
 ( #29813, #24539, #47865, #28957, #10978, #10684, #25397, #55840, #15391, #46999, #42552, #56129, #48430, #4123, #3266, #39837, #12403, #22123, #21257, #49298, #3832, #26262, #21831, #8550, #12966, #8850, #35104, #57852, #4422, #40133, #39263, #58146, #44568, #17409, #34822, #35391, #22422, #44275, #53422, #30965, #53138, #26541, #53727, #44868, #26840, #49002, #34531, #39553, #17713, #52850, #16549, #35698, #13266, #31257, #17119, #43995, #40434, #52564, #12116, #7972, #25969, #30101, #48152, #57558, #7683, #30394, #25684 ) ),
 .UNSPECIFIED., .F., .F., .F.,
 ( 4, 4 ),
 ( 4, 1, 1, 1, 1, 1, 1, 1, 1, 1, 1, 1, 1, 1, 1, 1, 1, 1, 1, 1, 1, 1, 1, 1, 1, 1, 1, 1, 1, 1, 1, 1, 1, 1, 1, 1, 1, 1, 1, 1, 1, 1, 1, 1, 1, 1, 1, 1, 1, 1, 1, 1, 1, 1, 1, 1, 1, 1, 1, 1, 1, 1, 1, 1, 4 ),
 ( -0.5168282991434000051, 1.516828299142999992 ),
 ( -0.02000000000000000042, -0.003749999999999999861, 0.01250000000000000069, 0.02875000000000000125, 0.04499999999999999833, 0.06124999999999999889, 0.07749999999999999944, 0.09375000000000000000, 0.1100000000000000006, 0.1262500000000000011, 0.1424999999999999878, 0.1587500000000000022, 0.1749999999999999889, 0.1912500000000000033, 0.2074999999999999900, 0.2237500000000000044, 0.2399999999999999911, 0.2562499999999999778, 0.2725000000000000200, 0.2887500000000000067, 0.3049999999999999933, 0.3212499999999999800, 0.3375000000000000222, 0.3537500000000000089, 0.3699999999999999956, 0.3862499999999999822, 0.4025000000000000244, 0.4187500000000000111, 0.4349999999999999978, 0.4512499999999999845, 0.4675000000000000266, 0.4837500000000000133, 0.5000000000000000000, 0.5162499999999999867, 0.5324999999999999734, 0.5487499999999999600, 0.5649999999999999467, 0.5812500000000000444, 0.5975000000000000311, 0.6137500000000000178, 0.6300000000000000044, 0.6462499999999999911, 0.6624999999999999778, 0.6787499999999999645, 0.6949999999999999512, 0.7112500000000000488, 0.7275000000000000355, 0.7437500000000000222, 0.7600000000000000089, 0.7762499999999999956, 0.7924999999999999822, 0.8087499999999999689, 0.8249999999999999556, 0.8412500000000000533, 0.8575000000000000400, 0.8737500000000000266, 0.8900000000000000133, 0.9062500000000000000, 0.9224999999999999867, 0.9387499999999999734, 0.9549999999999999600, 0.9712499999999999467, 0.9875000000000000444, 1.003749999999999920, 1.020000000000000018 ),
 .UNSPECIFIED. ) ;
#2674=DIRECTION ( 'NONE',  ( 0.000000000000000000, -1.000000000000000000, 0.000000000000000000 ) ) ;
#2677=CARTESIAN_POINT ( 'NONE',  ( 9.375326036246072192, -76.27905215015013596, 5.420036776477389573 ) ) ;
#2678=CARTESIAN_POINT ( 'NONE',  ( -6.606163316386915341, -78.52711955731416538, 8.596028648480132262 ) ) ;
#2682=CARTESIAN_POINT ( 'NONE',  ( -6.722591978632999066, -76.33855707708200100, -10.50348591810000087 ) ) ;
#2683=CARTESIAN_POINT ( 'NONE',  ( -4.872804940501344717, -78.68772107945071070, -9.582789324058202496 ) ) ;
#2695=CARTESIAN_POINT ( 'NONE',  ( -0.2721098858049000313, -79.21082493523199730, 11.21356619464000026 ) ) ;
#2697=ORIENTED_EDGE ( 'NONE', *, *, #42819, .F. ) ;
#2702=CARTESIAN_POINT ( 'NONE',  ( 10.79432616025544611, -77.57799259947435644, -3.050267481686816939 ) ) ;
#2708=EDGE_CURVE ( 'NONE', #53789, #24195, #958, .T. ) ;
#2716=CARTESIAN_POINT ( 'NONE',  ( 11.97742283006000186, -77.81769738389299107, 0.2395971301470000148 ) ) ;
#2719=CIRCLE ( 'NONE', #8341, 10.25000000000000000 ) ;
#2724=CARTESIAN_POINT ( 'NONE',  ( 10.06402303786000196, -78.24492912598299199, -4.229752508564000202 ) ) ;
#2725=CARTESIAN_POINT ( 'NONE',  ( 8.596418555780450887, -79.19791666666667140, -6.606377239730321982 ) ) ;
#2726=CARTESIAN_POINT ( 'NONE',  ( -10.51811773240999948, -81.00517844751929886, 2.900480251473000148 ) ) ;
#2728=ORIENTED_EDGE ( 'NONE', *, *, #37415, .F. ) ;
#2731=CARTESIAN_POINT ( 'NONE',  ( -5.751434148371999733, -77.84826253771599625, -9.630115047516998317 ) ) ;
#2735=CARTESIAN_POINT ( 'NONE',  ( -11.14126686682999967, -76.54389604793398405, 4.853629488117999990 ) ) ;
#2756=CARTESIAN_POINT ( 'NONE',  ( -2.812084287824942574, -81.00000000000000000, -10.57161323837342159 ) ) ;
#2757=CARTESIAN_POINT ( 'NONE',  ( -7.506332976489000330, -77.13807570069999997, -7.926558599818001483 ) ) ;
#2761=B_SPLINE_CURVE_WITH_KNOTS ( 'NONE', 3,
 ( #32593, #11357, #47092, #6623, #46219, #24634, #10477, #15773, #1344, #33765, #5745, #51803, #23753, #55345, #24045, #46512, #14888, #32886, #50930, #28463, #6036, #1632 ),
 .UNSPECIFIED., .F., .F.,
 ( 4, 2, 2, 2, 2, 2, 2, 2, 2, 2, 4 ),
 ( 0.000000000000000000, 0.06249999999999995837, 0.1249999999999999167, 0.2500000000000000000, 0.3750000000000000000, 0.5000000000000001110, 0.6250000000000001110, 0.7500000000000001110, 0.8125000000000001110, 0.8750000000000001110, 1.000000000000000000 ),
 .UNSPECIFIED. ) ;
#2765=CARTESIAN_POINT ( 'NONE',  ( 5.643184558664585460, -76.28046875019616380, -9.211581335339863230 ) ) ;
#2804=FACE_OUTER_BOUND ( 'NONE', #5564, .T. ) ;
#2808=CARTESIAN_POINT ( 'NONE',  ( -6.550114462690999950, -76.71554859108100288, -8.876808543633000426 ) ) ;
#2814=CARTESIAN_POINT ( 'NONE',  ( 7.627621379903384735, -80.28777230127180076, -7.575081149988561080 ) ) ;
#2817=CARTESIAN_POINT ( 'NONE',  ( 6.536979956083999177, -79.16903447980999431, -10.09826910480999906 ) ) ;
#2819=CARTESIAN_POINT ( 'NONE',  ( 10.97564558566000059, -79.09139468996799849, 2.523721168482999655 ) ) ;
#2822=VERTEX_POINT ( 'NONE', #57977 ) ;
#2836=CARTESIAN_POINT ( 'NONE',  ( 6.200214177871735899, -79.80000000000001137, 10.15137242043624966 ) ) ;
#2837=CARTESIAN_POINT ( 'NONE',  ( -5.074860051582180454, -80.01429829952145667, 9.477187767418271847 ) ) ;
#2840=CARTESIAN_POINT ( 'NONE',  ( -1.432420283025999996, -76.28690332460300283, 11.09153081809999897 ) ) ;
#2841=CARTESIAN_POINT ( 'NONE',  ( -8.707837037439713157, -76.54997136955654469, 6.490898182015857110 ) ) ;
#2844=CARTESIAN_POINT ( 'NONE',  ( 10.16646861257000012, -76.10830213011298895, 4.767248372777999954 ) ) ;
#2851=CARTESIAN_POINT ( 'NONE',  ( -5.997359202501453268, -78.02227085838593723, 8.921436172744598991 ) ) ;
#2859=CARTESIAN_POINT ( 'NONE',  ( 6.365665562422999635, -79.13050366622999832, 10.17242851768000023 ) ) ;
#2869=CARTESIAN_POINT ( 'NONE',  ( -6.711381441964999972, -80.17578567971679604, 9.048015653393999713 ) ) ;
#2873=DIRECTION ( 'NONE',  ( 0.000000000000000000, -1.000000000000000000, 0.000000000000000000 ) ) ;
#2878=EDGE_CURVE ( 'NONE', #28730, #12876, #9840, .T. ) ;
#2879=VERTEX_POINT ( 'NONE', #42317 ) ;
#2880=DIRECTION ( 'NONE',  ( 4.860620543616000107E-11, -1.000000000000000000, 3.762834028070999803E-10 ) ) ;
#2889=ORIENTED_EDGE ( 'NONE', *, *, #50634, .F. ) ;
#2895=VECTOR ( 'NONE', #57044, 1000.000000000000000 ) ;
#2904=CARTESIAN_POINT ( 'NONE',  ( -11.19161167724979222, -80.34518168142261629, 0.6576043368013242407 ) ) ;
#2905=CARTESIAN_POINT ( 'NONE',  ( -6.777984382448001277, -78.22714382231113461, -9.878005474088999094 ) ) ;
#2906=FACE_OUTER_BOUND ( 'NONE', #17702, .T. ) ;
#2915=CARTESIAN_POINT ( 'NONE',  ( 4.297951556683999641, -76.65176905123000495, -11.50435740523999861 ) ) ;
#2922=CARTESIAN_POINT ( 'NONE',  ( 8.012523733906446566, -78.71708638852500428, 8.990154430766319038 ) ) ;
#2924=CARTESIAN_POINT ( 'NONE',  ( 6.129172116842999785, -77.77411607459599452, 10.50789130831999962 ) ) ;
#2932=CARTESIAN_POINT ( 'NONE',  ( -6.394435847298999498, -79.27158651582300308, -10.20310948103000115 ) ) ;
#2943=CARTESIAN_POINT ( 'NONE',  ( -5.279640230871068596, -76.43576352588647183, -9.859185912017370157 ) ) ;
#2944=CARTESIAN_POINT ( 'NONE',  ( 8.047230821198958495, -79.23460565973853420, -8.591241732543773324 ) ) ;
#2957=CARTESIAN_POINT ( 'NONE',  ( 0.000000000000000000, -79.79999999999999716, 0.000000000000000000 ) ) ;
#2961=CARTESIAN_POINT ( 'NONE',  ( 5.596253190686999446, -76.48824961810498735, -11.27629867687000065 ) ) ;
#2962=CARTESIAN_POINT ( 'NONE',  ( 4.129401235074444010, -78.75639348479435853, -9.925231067652177330 ) ) ;
#2972=CARTESIAN_POINT ( 'NONE',  ( -6.206245474241999460, -79.75555179526899963, 9.343480492029000217 ) ) ;
#2994=EDGE_CURVE ( 'NONE', #3745, #31953, #5640, .T. ) ;
#2995=DIRECTION ( 'NONE',  ( 0.000000000000000000, -1.000000000000000000, 0.000000000000000000 ) ) ;
#3000=CARTESIAN_POINT ( 'NONE',  ( -11.70000000000000107, -80.79999999999999716, 0.000000000000000000 ) ) ;
#3002=CARTESIAN_POINT ( 'NONE',  ( -5.687706977064000746, -77.98047327643499216, 10.54353137130999940 ) ) ;
#3009=CARTESIAN_POINT ( 'NONE',  ( -6.481772035086000194, -77.10100271990599197, -8.784189910979000260 ) ) ;
#3015=CARTESIAN_POINT ( 'NONE',  ( -7.421735313277000756, -79.75327784566698597, 9.772525563196001741 ) ) ;
#3016=CARTESIAN_POINT ( 'NONE',  ( 12.00000000000000000, -77.04999999999999716, 0.000000000000000000 ) ) ;
#3020=CARTESIAN_POINT ( 'NONE',  ( 11.82336703301000114, -76.80802521606899802, -2.809544199102999684 ) ) ;
#3023=ORIENTED_EDGE ( 'NONE', *, *, #17197, .T. ) ;
#3024=CARTESIAN_POINT ( 'NONE',  ( 7.679819846117000637, -78.82741272537499810, -7.919728626202000576 ) ) ;
#3026=EDGE_CURVE ( 'NONE', #8229, #8361, #4019, .T. ) ;
#3031=CARTESIAN_POINT ( 'NONE',  ( 12.00000000000000888, -79.53958333333332575, -1.570796326794872577 ) ) ;
#3037=CYLINDRICAL_SURFACE ( 'NONE', #46262, 10.75000000000000000 ) ;
#3042=ORIENTED_EDGE ( 'NONE', *, *, #46991, .F. ) ;
#3048=CARTESIAN_POINT ( 'NONE',  ( 3.399186938124000079, -81.00000000000000000, -10.46162167925000119 ) ) ;
#3049=CARTESIAN_POINT ( 'NONE',  ( -3.535896000267000350, -76.97465764268899591, 10.32825277893000226 ) ) ;
#3052=AXIS2_PLACEMENT_3D ( 'NONE', #44830, #36259, #26502 ) ;
#3053=CARTESIAN_POINT ( 'NONE',  ( 8.554126827399000987, -79.89233811873450009, -7.255689219360999864 ) ) ;
#3056=B_SPLINE_CURVE_WITH_KNOTS ( 'NONE', 3,
 ( #4437, #26856, #4142, #26556, #35410, #8864, #36816, #27948, #50417, #40149, #16857, #21847, #58161, #35122, #57294, #17727, #54834, #35715 ),
 .UNSPECIFIED., .F., .F.,
 ( 4, 2, 2, 2, 2, 2, 2, 2, 4 ),
 ( 0.000000000000000000, 0.1250000000000000000, 0.2499999999999999722, 0.3750000000000000000, 0.5000000000000000000, 0.6250000000000000000, 0.7500000000000000000, 0.8750000000000000000, 1.000000000000000000 ),
 .UNSPECIFIED. ) ;
#3072=CARTESIAN_POINT ( 'NONE',  ( 8.770451247185000909, -79.01131779197200444, 8.160602927202999624 ) ) ;
#3078=CARTESIAN_POINT ( 'NONE',  ( 0.000000000000000000, -76.00000000000000000, -11.04999999999995275 ) ) ;
#3079=CARTESIAN_POINT ( 'NONE',  ( -0.8287201338969000242, -77.44254838670400432, -11.23152649900999833 ) ) ;
#3083=CARTESIAN_POINT ( 'NONE',  ( 0.000000000000000000, -87.29999999999999716, 0.000000000000000000 ) ) ;
#3095=ADVANCED_FACE ( 'NONE', ( #16321 ), #45280, .F. ) ;
#3096=AXIS2_PLACEMENT_3D ( 'NONE', #8865, #40453, #9164 ) ;
#3099=CARTESIAN_POINT ( 'NONE',  ( 6.290530912463999869, -78.03614743357699979, 9.202381290206000486 ) ) ;
#3105=CARTESIAN_POINT ( 'NONE',  ( -2.054101735612868129, -80.20991162323984724, -10.55179437476100013 ) ) ;
#3108=CARTESIAN_POINT ( 'NONE',  ( -10.39774148753954641, -79.88051113478326215, -4.208156475417354159 ) ) ;
#3112=CARTESIAN_POINT ( 'NONE',  ( 7.652056849482000267, -79.31845263404798629, 9.281873293285000770 ) ) ;
#3114=CARTESIAN_POINT ( 'NONE',  ( 0.9616906432773000279, -78.95521297495899660, -11.22092312000000014 ) ) ;
#3115=CARTESIAN_POINT ( 'NONE',  ( 9.393509054760620813, -77.39172388621676646, 5.413909507467279170 ) ) ;
#3119=ORIENTED_EDGE ( 'NONE', *, *, #17784, .F. ) ;
#3133=CARTESIAN_POINT ( 'NONE',  ( -8.667213820335565089, -80.04983638533551016, 6.359185785815872016 ) ) ;
#3135=CARTESIAN_POINT ( 'NONE',  ( -9.939389728518001732, -76.79599943707599152, 5.126617716248000001 ) ) ;
#3140=CARTESIAN_POINT ( 'NONE',  ( -4.770269334038999887, -76.30143890447099864, 10.03813491106999933 ) ) ;
#3143=FACE_OUTER_BOUND ( 'NONE', #47788, .T. ) ;
#3147=CARTESIAN_POINT ( 'NONE',  ( -2.206042088423531222, -77.99158609026490296, 10.52113899700466781 ) ) ;
#3152=VECTOR ( 'NONE', #49791, 1000.000000000000000 ) ;
#3163=CARTESIAN_POINT ( 'NONE',  ( -11.09105850093000001, -80.23598105172408168, 1.974238845993000258 ) ) ;
#3170=CARTESIAN_POINT ( 'NONE',  ( -0.4597697825790413861, -79.97871958790278768, 10.74439705486481067 ) ) ;
#3179=AXIS2_PLACEMENT_3D ( 'NONE', #19689, #45696, #37390 ) ;
#3183=CARTESIAN_POINT ( 'NONE',  ( -0.7974440169908999509, -78.81086622188499291, -12.02330465019000094 ) ) ;
#3185=ORIENTED_EDGE ( 'NONE', *, *, #8365, .T. ) ;
#3199=FACE_BOUND ( 'NONE', #5719, .T. ) ;
#3200=CARTESIAN_POINT ( 'NONE',  ( 4.212091869424105184, -80.69420159946982096, 10.38955714771617522 ) ) ;
#3201=CARTESIAN_POINT ( 'NONE',  ( -11.86109855474000163, -78.66121286909155685, -1.682380905047000219 ) ) ;
#3209=CARTESIAN_POINT ( 'NONE',  ( -3.699256142337000064, -76.89766548106000243, 11.71059914860999918 ) ) ;
#3212=DIRECTION ( 'NONE',  ( -1.000000000000000000, 0.000000000000000000, 0.000000000000000000 ) ) ;
#3220=CARTESIAN_POINT ( 'NONE',  ( 9.940990682305997694, -78.64225416815600056, -7.011364793726000855 ) ) ;
#3225=CARTESIAN_POINT ( 'NONE',  ( -6.312747718300130373, -79.52497251010836976, 8.701216629874789277 ) ) ;
#3228=CARTESIAN_POINT ( 'NONE',  ( -11.00710520982000062, -79.72435824023099826, -4.882200574570999763 ) ) ;
#3232=DIRECTION ( 'NONE',  ( 1.000000000000000000, 0.000000000000000000, 0.000000000000000000 ) ) ;
#3241=EDGE_CURVE ( 'NONE', #12329, #353, #49848, .T. ) ;
#3256=CARTESIAN_POINT ( 'NONE',  ( 9.642431301336001681, -77.02102521606900609, -8.092989473023999736 ) ) ;
#3257=CARTESIAN_POINT ( 'NONE',  ( 2.342876876834760758, -78.74262638912878742, -10.49166047009287261 ) ) ;
#3258=ORIENTED_EDGE ( 'NONE', *, *, #2878, .T. ) ;
#3266=CARTESIAN_POINT ( 'NONE',  ( -11.20683111097000051, -79.90504937755049752, -0.4743912329535999728 ) ) ;
#3283=CARTESIAN_POINT ( 'NONE',  ( -8.734850699938000673, -79.58966986058341320, 8.271005326623001253 ) ) ;
#3290=CARTESIAN_POINT ( 'NONE',  ( 11.53501176087999980, -78.72656418587199312, -3.234124663588000104 ) ) ;
#3294=CARTESIAN_POINT ( 'NONE',  ( -8.968518105033201238, -76.34128233971088662, 8.069401009964305871 ) ) ;
#3303=CARTESIAN_POINT ( 'NONE',  ( -3.799897982867999957, -79.72664421481898955, 11.66812693903999865 ) ) ;
#3304=DIRECTION ( 'NONE',  ( -1.000000000000000000, 0.000000000000000000, 0.000000000000000000 ) ) ;
#3307=DIRECTION ( 'NONE',  ( 1.000000000000000000, 0.000000000000000000, 0.000000000000000000 ) ) ;
#3308=CARTESIAN_POINT ( 'NONE',  ( -10.53979166895999953, -76.55163446013099815, -6.281747244366999716 ) ) ;
#3312=CARTESIAN_POINT ( 'NONE',  ( 5.587778422887999419, -79.87564813785350282, -9.645275144704999803 ) ) ;
#3321=CARTESIAN_POINT ( 'NONE',  ( 8.696932689530999738, -76.29999999999999716, -6.318691462144000681 ) ) ;
#3334=CARTESIAN_POINT ( 'NONE',  ( -4.522750724863999316, -77.98240233375699404, 9.935798501838000618 ) ) ;
#3335=VECTOR ( 'NONE', #54267, 1000.000000000000114 ) ;
#3337=CARTESIAN_POINT ( 'NONE',  ( 3.507155896972999898, -79.04801148567800340, 10.65448112794999957 ) ) ;
#3353=CARTESIAN_POINT ( 'NONE',  ( 11.88382656225999945, -78.44160216807300401, -1.513515996960000054 ) ) ;
#3355=EDGE_CURVE ( 'NONE', #37074, #8174, #57905, .T. ) ;
#3361=CARTESIAN_POINT ( 'NONE',  ( 6.459716167540999976, -77.49702107270799445, -9.225293035625000471 ) ) ;
#3363=CARTESIAN_POINT ( 'NONE',  ( 0.5376952571279000059, -80.69460651026599862, 11.24298004781999971 ) ) ;
#3365=ORIENTED_EDGE ( 'NONE', *, *, #5634, .T. ) ;
#3383=CARTESIAN_POINT ( 'NONE',  ( -3.190971086128000067, -76.74278493408199608, -10.56027646911999973 ) ) ;
#3389=CARTESIAN_POINT ( 'NONE',  ( -5.498018440344079494, -80.18236152930400351, -9.239502841344624073 ) ) ;
#3390=CARTESIAN_POINT ( 'NONE',  ( -5.930212039233577315, -76.09166666665643675, 10.26675032132114040 ) ) ;
#3391=CARTESIAN_POINT ( 'NONE',  ( 4.782544914675210812, -79.68985673377078172, 10.14637241100733434 ) ) ;
#3392=CARTESIAN_POINT ( 'NONE',  ( -8.734850699938000673, -79.43798715743798766, 8.271005326623001253 ) ) ;
#3395=CARTESIAN_POINT ( 'NONE',  ( 5.414072109562871660, -77.43337924860836097, 9.393465288415251635 ) ) ;
#3402=CARTESIAN_POINT ( 'NONE',  ( -10.75000000000000000, -78.50000000000000000, 0.000000000000000000 ) ) ;
#3411=CARTESIAN_POINT ( 'NONE',  ( 0.000000000000000000, -75.15999999999999659, 0.000000000000000000 ) ) ;
#3414=CARTESIAN_POINT ( 'NONE',  ( -4.824611332692330556, -80.01213778624108386, 9.606459940033937883 ) ) ;
#3419=VECTOR ( 'NONE', #39889, 1000.000000000000000 ) ;
#3422=CARTESIAN_POINT ( 'NONE',  ( 9.860379324123998757, -76.74539509872099075, 4.873887145968000212 ) ) ;
#3442=CARTESIAN_POINT ( 'NONE',  ( 8.735587516832000077, -80.07898629742850005, 6.757696599697999851 ) ) ;
#3447=CARTESIAN_POINT ( 'NONE',  ( -2.935164356122387908, -79.99732793198559477, 10.34225144355774617 ) ) ;
#3453=ORIENTED_EDGE ( 'NONE', *, *, #38507, .F. ) ;
#3458=AXIS2_PLACEMENT_3D ( 'NONE', #15490, #47098, #28759 ) ;
#3475=CARTESIAN_POINT ( 'NONE',  ( 0.000000000000000000, -82.00000000000000000, 0.000000000000000000 ) ) ;
#3477=CARTESIAN_POINT ( 'NONE',  ( -9.690626710582000314, -78.20001450688755540, -7.043281791253000357 ) ) ;
#3485=CARTESIAN_POINT ( 'NONE',  ( 6.725657209017000149, -77.17088373642599208, -9.843613558058999402 ) ) ;
#3487=AXIS2_PLACEMENT_3D ( 'NONE', #5752, #19053, #37042 ) ;
#3497=CARTESIAN_POINT ( 'NONE',  ( 0.4919088493939999807, -77.31291771239200727, 12.15485731165999894 ) ) ;
#3503=CARTESIAN_POINT ( 'NONE',  ( -7.608827018420656785, -79.53773796140059460, 7.593810091919143801 ) ) ;
#3506=CARTESIAN_POINT ( 'NONE',  ( -5.548968227290999700, -79.70989843751300441, -10.55673919551000139 ) ) ;
#3516=ORIENTED_EDGE ( 'NONE', *, *, #38191, .F. ) ;
#3517=B_SPLINE_CURVE_WITH_KNOTS ( 'NONE', 3,
 ( #51296, #47461, #43295, #32958, #38565, #6698, #19695, #43009, #2567, #19404, #11146, #42135, #20567, #33835, #56580, #20280, #55413, #52160, #56006, #6109, #24117, #16140, #1701, #42719, #33254, #33549, #51588, #37695, #14961, #34116, #10852, #51873, #28825, #55714, #10552, #11716, #29120, #11427, #29693, #29408, #24416, #46874, #6401, #42432, #2001, #47166, #19996, #24707, #2284, #38274, #8944, #54112, #49986, #9530, #39930, #13946, #13653, #40821, #8646, #21134, #31648, #44962, #57946, #49395, #27515, #31354, #26931, #13356, #40228, #49691, #413, #31942, #54408, #4517, #20848, #26631, #22518, #17500, #2851, #40528, #18391, #4220, #35789, #35488, #22217, #122, #53820, #58240, #9237, #36382, #18099, #36095, #38852, #27223, #43584, #16429, #56871, #45262, #34412, #4810, #52441, #12001, #53518, #22810, #44666, #17803, #29979, #48033, #7564, #25564, #3147, #13059, #31058, #49095, #41987, #1853, #41111, #36676, #37255, #45556, #10404, #23681, #15111, #55861, #5671, #41694, #45853, #10996, #15413, #702, #5102, #1272, #46436, #19263, #50563, #14526, #46146, #33406, #18684, #33108, #28097, #23101, #55267, #18973, #14815, #19547, #54692, #32812, #51151, #10706, #5386, #14234, #51444, #32232, #50274, #50859, #5965, #28389, #10117, #32519, #23968, #9822, #1556, #27806, #37545, #23393, #55562, #36964, #28683, #46735, #41405, #6254, #24269, #42285 ),
 .UNSPECIFIED., .F., .F.,
 ( 4, 2, 2, 2, 1, 1, 1, 2, 2, 2, 2, 1, 1, 1, 1, 1, 2, 2, 2, 2, 2, 1, 1, 1, 1, 2, 2, 2, 1, 2, 2, 1, 1, 1, 1, 1, 1, 2, 2, 2, 2, 2, 1, 1, 1, 2, 2, 2, 2, 1, 1, 1, 2, 2, 2, 2, 1, 1, 1, 2, 2, 2, 1, 1, 1, 1, 1, 2, 2, 2, 2, 2, 1, 1, 1, 1, 2, 2, 2, 2, 2, 2, 2, 2, 2, 2, 2, 2, 1, 1, 1, 2, 2, 2, 1, 1, 2, 2, 1, 1, 2, 2, 2, 2, 1, 2, 2, 1, 2, 4 ),
 ( 0.000000000000000000, 0.03125000000004676121, 0.04687500000007015916, 0.05468750000008183038, 0.05859375000008768680, 0.06054687500009063583, 0.06152343750009210688, 0.06201171875009282852, 0.06250000000009355017, 0.09375000000013758439, 0.1093750000001596362, 0.1171875000001706552, 0.1210937500001761785, 0.1230468750001789263, 0.1240234375001803419, 0.1245117187501810357, 0.1247558593751813966, 0.1250000000001817435, 0.1562500000002016165, 0.1718750000002115252, 0.1796875000002164657, 0.1835937500002188805, 0.1855468750002200740, 0.1865234375002206846, 0.1870117187502209621, 0.1872558593752211009, 0.1875000000002212397, 0.2031250000002264577, 0.2109375000002290113, 0.2148437500002303435, 0.2187500000002316480, 0.2343750000002371714, 0.2421875000002399470, 0.2460937500002412792, 0.2480468750002420286, 0.2490234375002424450, 0.2495117187502426670, 0.2497558593752427503, 0.2500000000002428058, 0.2656250000002447487, 0.2734375000002456924, 0.2773437500002461920, 0.2792968750002464140, 0.2802734375002465250, 0.2807617187502465805, 0.2810058593752466360, 0.2812500000002466360, 0.2968750000002501888, 0.3046875000002519096, 0.3085937500002527978, 0.3105468750002532419, 0.3115234375002534639, 0.3120117187502535749, 0.3125000000002536304, 0.3281250000002541301, 0.3359375000002544076, 0.3398437500002545186, 0.3417968750002544631, 0.3427734375002545186, 0.3432617187502545741, 0.3437500000002546297, 0.3593750000002553513, 0.3671875000002556844, 0.3710937500002557954, 0.3730468750002559064, 0.3740234375002558509, 0.3745117187502558509, 0.3747558593752558509, 0.3750000000002557954, 0.4062500000002492451, 0.4218750000002459699, 0.4296875000002443601, 0.4335937500002434719, 0.4355468750002430278, 0.4365234375002428058, 0.4370117187502426948, 0.4372558593752426392, 0.4375000000002425282, 0.4687500000002331468, 0.4843750000002284284, 0.4921875000002260414, 0.4960937500002248757, 0.5000000000002235989, 0.5625000000002046141, 0.6250000000001857403, 0.6406250000001809664, 0.6425781250001804112, 0.6435546875001800782, 0.6445312500001797451, 0.6484375000001786349, 0.6562500000001763034, 0.6875000000001670886, 0.7500000000001487699, 0.8125000000001304512, 0.8437500000001213474, 0.8476562500001202372, 0.8496093750001195710, 0.8500976562501194600, 0.8505859375001192380, 0.8515625000001189049, 0.8593750000001161293, 0.8750000000001104672, 0.9062500000000992539, 0.9218750000000937028, 0.9238281250000927036, 0.9248046875000915934, 0.9257812500000903722, 0.9296875000000855982, 0.9375000000000761613, 1.000000000000000000 ),
 .UNSPECIFIED. ) ;
#3534=CARTESIAN_POINT ( 'NONE',  ( 12.43062359974000053, -76.50248803030198985, -0.9980395665033999775 ) ) ;
#3537=ORIENTED_EDGE ( 'NONE', *, *, #6365, .T. ) ;
#3543=CARTESIAN_POINT ( 'NONE',  ( 3.895497176767999559, -77.09677593747389324, 10.51870773133999926 ) ) ;
#3559=LINE ( 'NONE', #26552, #51524 ) ;
#3570=CARTESIAN_POINT ( 'NONE',  ( 7.483561698776000526, -78.31962445451600274, 9.354804580292000793 ) ) ;
#3573=CARTESIAN_POINT ( 'NONE',  ( 2.687462146607000335, -77.71966499545499119, -11.62811462177000088 ) ) ;
#3579=ORIENTED_EDGE ( 'NONE', *, *, #2518, .T. ) ;
#3582=CARTESIAN_POINT ( 'NONE',  ( -9.570476163416000048, -79.38040701380199948, -7.680520617063000266 ) ) ;
#3583=EDGE_CURVE ( 'NONE', #49218, #13366, #20951, .T. ) ;
#3587=CARTESIAN_POINT ( 'NONE',  ( -11.96958589357000058, -75.93049390057900894, 1.626211782151000040 ) ) ;
#3590=ORIENTED_EDGE ( 'NONE', *, *, #46709, .T. ) ;
#3591=CARTESIAN_POINT ( 'NONE',  ( -0.2676215762113999808, -79.01806712638799013, 11.02860431212999970 ) ) ;
#3600=CARTESIAN_POINT ( 'NONE',  ( -1.881092013513000039, -78.21382883426899468, 12.13496073407999987 ) ) ;
#3612=CARTESIAN_POINT ( 'NONE',  ( 3.791268666074999683, -76.92018495668600053, 10.23726759892000082 ) ) ;
#3616=CARTESIAN_POINT ( 'NONE',  ( -2.848564863371000122, -78.80288439866200179, -10.84913769893999991 ) ) ;
#3617=ORIENTED_EDGE ( 'NONE', *, *, #38962, .F. ) ;
#3633=ORIENTED_EDGE ( 'NONE', *, *, #2452, .T. ) ;
#3635=CARTESIAN_POINT ( 'NONE',  ( -6.506018757879999725, -79.93025345888189293, 9.866615368227002136 ) ) ;
#3637=CARTESIAN_POINT ( 'NONE',  ( 0.9627474882855999727, -78.33308490637799082, -11.94107121277999894 ) ) ;
#3644=CARTESIAN_POINT ( 'NONE',  ( -10.91036644271999911, -76.84334884066400662, -2.792455208340000272 ) ) ;
#3660=CIRCLE ( 'NONE', #29108, 11.05000000000000071 ) ;
#3665=CARTESIAN_POINT ( 'NONE',  ( -10.09586848912000079, -78.24005621299899360, 4.990731814912999553 ) ) ;
#3671=CARTESIAN_POINT ( 'NONE',  ( -1.794921875279598122, -80.21179327765182165, -10.59966322526386229 ) ) ;
#3672=CARTESIAN_POINT ( 'NONE',  ( 2.813789756862274505, -77.14583333333334281, -10.47020627418438821 ) ) ;
#3674=CARTESIAN_POINT ( 'NONE',  ( -7.858171174022000827, -78.92996543302999157, 9.108036400545000077 ) ) ;
#3676=CARTESIAN_POINT ( 'NONE',  ( 1.104250457816000175, -79.69059423600799619, 11.20779173096999948 ) ) ;
#3684=FACE_OUTER_BOUND ( 'NONE', #58058, .T. ) ;
#3685=CARTESIAN_POINT ( 'NONE',  ( -10.76888293467999880, -79.08652177698400010, -1.790677617362999907 ) ) ;
#3688=VERTEX_POINT ( 'NONE', #35977 ) ;
#3703=CARTESIAN_POINT ( 'NONE',  ( -10.78744351475000052, -76.53722080125399430, -1.449653075750000131 ) ) ;
#3715=VERTEX_POINT ( 'NONE', #3810 ) ;
#3727=CARTESIAN_POINT ( 'NONE',  ( -10.34138800174999950, -80.71754402778218207, 4.468208825537999473 ) ) ;
#3733=CARTESIAN_POINT ( 'NONE',  ( -3.202240918582688334, -79.99931087886648129, 10.26207580309217349 ) ) ;
#3735=ORIENTED_EDGE ( 'NONE', *, *, #12317, .F. ) ;
#3745=VERTEX_POINT ( 'NONE', #48982 ) ;
#3756=ORIENTED_EDGE ( 'NONE', *, *, #55347, .T. ) ;
#3762=CARTESIAN_POINT ( 'NONE',  ( 1.283537837596413045, -80.98401907456398874, -11.03296757967288677 ) ) ;
#3771=CARTESIAN_POINT ( 'NONE',  ( -8.987350104473000201, -76.93864821936499254, 8.369597699504998545 ) ) ;
#3773=CARTESIAN_POINT ( 'NONE',  ( 3.042547531669000271, -78.24783470746899638, -10.31045122763999977 ) ) ;
#3779=AXIS2_PLACEMENT_3D ( 'NONE', #2104, #29513, #47568 ) ;
#3781=CARTESIAN_POINT ( 'NONE',  ( -0.8126767071385999630, -78.49313915747200099, -12.25297252704000073 ) ) ;
#3784=CARTESIAN_POINT ( 'NONE',  ( -1.407171709420418138, -79.11458333333331439, -10.75000000000000000 ) ) ;
#3788=CARTESIAN_POINT ( 'NONE',  ( -5.583693648563480494, -79.51845993124416623, 9.199230099472547550 ) ) ;
#3790=CARTESIAN_POINT ( 'NONE',  ( -6.745911349169845472, -78.82231418035541992, 9.981325353439961745 ) ) ;
#3791=CARTESIAN_POINT ( 'NONE',  ( -11.34557120194999946, -79.21831925412799080, -4.033641907284000183 ) ) ;
#3792=CARTESIAN_POINT ( 'NONE',  ( -3.008550086500999754, -80.47034076625139676, 10.63866553953000071 ) ) ;
#3794=CARTESIAN_POINT ( 'NONE',  ( -2.047671225339077468E-06, -76.25353340279926329, -10.79679441329301959 ) ) ;
#3799=ORIENTED_EDGE ( 'NONE', *, *, #26920, .T. ) ;
#3808=CONICAL_SURFACE ( 'NONE', #12328, 9.649999999909001147, 0.7853981633972997312 ) ;
#3810=CARTESIAN_POINT ( 'NONE',  ( 3.042547531669000271, -78.24783470746899638, -10.31045122763999977 ) ) ;
#3820=CARTESIAN_POINT ( 'NONE',  ( -9.039790932574998550, -77.13146751707299131, 8.418433967051999645 ) ) ;
#3821=CARTESIAN_POINT ( 'NONE',  ( -10.53015523610255144, -78.61621378903457469, -2.164481121597691349 ) ) ;
#3829=CARTESIAN_POINT ( 'NONE',  ( -6.884807209879997281, -78.32241137255587660, -8.855368954042999619 ) ) ;
#3832=CARTESIAN_POINT ( 'NONE',  ( 4.782478426736999744, -79.74163131954000505, 10.14623135401999932 ) ) ;
#3845=LINE ( 'NONE', #27142, #31714 ) ;
#3859=CARTESIAN_POINT ( 'NONE',  ( -11.01904509677000021, -78.04521678053998812, 4.584337204197000304 ) ) ;
#3869=CARTESIAN_POINT ( 'NONE',  ( 11.59999999999999964, -87.70000000000000284, 0.000000000000000000 ) ) ;
#3873=CARTESIAN_POINT ( 'NONE',  ( 12.30622754380999950, -76.18204548927899111, -1.412018855228999836 ) ) ;
#3877=VECTOR ( 'NONE', #5772, 1000.000000000000000 ) ;
#3878=CARTESIAN_POINT ( 'NONE',  ( 4.576365007000999796, -78.80017638237299593, -10.03785921918999868 ) ) ;
#3882=CARTESIAN_POINT ( 'NONE',  ( -10.75000000000000533, -76.49166666666666003, 1.125737367536309597 ) ) ;
#3883=CARTESIAN_POINT ( 'NONE',  ( 9.377644441546999943, -78.13244088799798703, 7.928150093746000771 ) ) ;
#3885=CARTESIAN_POINT ( 'NONE',  ( -10.75000000000000355, -78.48958333333331439, 1.407171709420384609 ) ) ;
#3886=EDGE_CURVE ( 'NONE', #616, #8229, #9683, .T. ) ;
#3890=CARTESIAN_POINT ( 'NONE',  ( 10.60216386470985839, -78.83683079414333861, -1.778172759129439395 ) ) ;
#3895=CARTESIAN_POINT ( 'NONE',  ( -6.481772035086000194, -76.64782152666799675, -8.784189910979000260 ) ) ;
#3898=CARTESIAN_POINT ( 'NONE',  ( 8.645668071321999548, -78.50328462564201004, 7.146365085715999044 ) ) ;
#3917=CARTESIAN_POINT ( 'NONE',  ( 8.190016797772999624, -79.75825050192599974, 9.199421104438000540 ) ) ;
#3919=CARTESIAN_POINT ( 'NONE',  ( 7.483561698776000526, -78.52299011434399745, 9.354804580292000793 ) ) ;
#3927=CARTESIAN_POINT ( 'NONE',  ( 0.5495723139228999576, -76.95229421267099212, -11.24864145460999865 ) ) ;
#3928=DIRECTION ( 'NONE',  ( 1.000000000000000000, 0.000000000000000000, 0.000000000000000000 ) ) ;
#3929=CARTESIAN_POINT ( 'NONE',  ( 4.329053196835999984, -80.47982502223689494, -10.39004403086999950 ) ) ;
#3937=CARTESIAN_POINT ( 'NONE',  ( 10.74983318585575631, -76.85537858145019641, 0.7036223827703862455 ) ) ;
#3942=DIRECTION ( 'NONE',  ( 0.000000000000000000, 1.000000000000000000, 0.000000000000000000 ) ) ;
#3945=CARTESIAN_POINT ( 'NONE',  ( -11.10013370946000144, -76.70156662648800250, 1.020686637641000205 ) ) ;
#3952=CARTESIAN_POINT ( 'NONE',  ( 4.121696569562778301, -80.25639609395949492, -9.928389259389652111 ) ) ;
#3953=CARTESIAN_POINT ( 'NONE',  ( -6.606377239730330864, -77.07291666666667140, -8.596418555780440229 ) ) ;
#3959=CARTESIAN_POINT ( 'NONE',  ( 4.752670204043000446, -79.73108495741900015, 10.08299194199999960 ) ) ;
#3970=CARTESIAN_POINT ( 'NONE',  ( -5.305451056584999492, -79.72621204443500176, -9.672327717035999584 ) ) ;
#3971=CARTESIAN_POINT ( 'NONE',  ( -3.140974612311351777, -76.40416666663691103, -11.68767212001978884 ) ) ;
#3977=ADVANCED_FACE ( 'NONE', ( #13735 ), #58327, .T. ) ;
#3981=CYLINDRICAL_SURFACE ( 'NONE', #54615, 10.75000000000000000 ) ;
#3989=CARTESIAN_POINT ( 'NONE',  ( 5.236819022057999540, -76.36164720732999456, 9.541811095419998168 ) ) ;
#3997=CARTESIAN_POINT ( 'NONE',  ( 11.02326530841000007, -81.16017192083839404, 1.187788371667000131 ) ) ;
#4002=DIRECTION ( 'NONE',  ( -1.776356839400000238E-14, -1.000000000000000000, 8.585724723767000453E-14 ) ) ;
#4013=CARTESIAN_POINT ( 'NONE',  ( -3.140974612311352221, -79.00416666666664867, -11.68767212001979061 ) ) ;
#4018=ORIENTED_EDGE ( 'NONE', *, *, #5557, .F. ) ;
#4019=B_SPLINE_CURVE_WITH_KNOTS ( 'NONE', 3,
 ( #45882, #23712, #5414, #41434, #1020, #1300, #41722, #19001, #55009, #14847, #32841, #51763, #38160, #11314, #56183, #34591, #3031, #29295 ),
 .UNSPECIFIED., .F., .F.,
 ( 4, 2, 2, 2, 2, 2, 2, 2, 4 ),
 ( 0.000000000000000000, 0.1250000000000000000, 0.2500000000000000000, 0.3750000000000000000, 0.5000000000000000000, 0.6250000000000000000, 0.7500000000000000000, 0.8750000000000000000, 1.000000000000000000 ),
 .UNSPECIFIED. ) ;
#4020=CARTESIAN_POINT ( 'NONE',  ( 7.615030601986474856, -77.28781258845663160, -7.587605221805258537 ) ) ;
#4028=ORIENTED_EDGE ( 'NONE', *, *, #48091, .F. ) ;
#4030=CARTESIAN_POINT ( 'NONE',  ( -7.209427067528999977, -77.61717634323900938, 9.655047023863000177 ) ) ;
#4034=CARTESIAN_POINT ( 'NONE',  ( 11.61765826232213250, -76.62845391823577756, -3.111680234998253525 ) ) ;
#4039=EDGE_CURVE ( 'NONE', #40109, #10164, #49176, .T. ) ;
#4041=DIRECTION ( 'NONE',  ( 0.000000000000000000, -1.000000000000000000, 0.000000000000000000 ) ) ;
#4049=CARTESIAN_POINT ( 'NONE',  ( 11.20799393363000185, -77.92872135264997269, 4.230477091134000389 ) ) ;
#4059=DIRECTION ( 'NONE',  ( 0.000000000000000000, 0.000000000000000000, -1.000000000000000000 ) ) ;
#4067=CARTESIAN_POINT ( 'NONE',  ( -8.418448289622000758, -78.08151106797200214, -6.950186643912999784 ) ) ;
#4069=CARTESIAN_POINT ( 'NONE',  ( -1.881092013513000039, -77.76064764102999050, 12.13496073407999987 ) ) ;
#4079=CARTESIAN_POINT ( 'NONE',  ( -11.88541927438999934, -79.62999754497099048, -0.9862366044713999358 ) ) ;
#4080=CARTESIAN_POINT ( 'NONE',  ( -9.997577002847000571, -80.67795857467889675, -4.987204589701000224 ) ) ;
#4083=CARTESIAN_POINT ( 'NONE',  ( 0.5473670387515998659, -76.96277908592900019, -11.20350390113000039 ) ) ;
#4097=DIRECTION ( 'NONE',  ( 0.000000000000000000, -1.000000000000000000, 0.000000000000000000 ) ) ;
#4107=ORIENTED_EDGE ( 'NONE', *, *, #58364, .T. ) ;
#4109=CARTESIAN_POINT ( 'NONE',  ( 8.222285421689999652, -77.37736394690199404, -8.489546592527000612 ) ) ;
#4111=CARTESIAN_POINT ( 'NONE',  ( -10.50169165321555553, -78.61722614632127204, -2.300187871545900098 ) ) ;
#4119=CARTESIAN_POINT ( 'NONE',  ( 9.668944085725000193, -77.04230325147001679, 5.685915129398998680 ) ) ;
#4120=CARTESIAN_POINT ( 'NONE',  ( 0.000000000000000000, -76.29999999999999716, 0.000000000000000000 ) ) ;
#4123=CARTESIAN_POINT ( 'NONE',  ( -10.39759693597000023, -79.93228572055228653, -4.208097972746998927 ) ) ;
#4137=CARTESIAN_POINT ( 'NONE',  ( -11.38972971424999869, -76.73218649614399567, -4.593112662244999811 ) ) ;
#4138=CYLINDRICAL_SURFACE ( 'NONE', #33583, 10.75000000000000000 ) ;
#4142=CARTESIAN_POINT ( 'NONE',  ( 10.47020627418439531, -79.72916666666665719, -2.813789756862242974 ) ) ;
#4143=CARTESIAN_POINT ( 'NONE',  ( -1.780884232981000181, -79.86231230381177681, -11.07459082487999957 ) ) ;
#4152=CARTESIAN_POINT ( 'NONE',  ( -9.654076420390000024, -78.12660472681200474, -7.016716533807999312 ) ) ;
#4166=CARTESIAN_POINT ( 'NONE',  ( -5.751434148371999733, -77.91605109099198501, -9.630115047516998317 ) ) ;
#4169=CARTESIAN_POINT ( 'NONE',  ( -11.24870262279999977, -76.47616898352099213, 4.900433263621000179 ) ) ;
#4174=CARTESIAN_POINT ( 'NONE',  ( 2.026540639977999714, -79.84841179485169960, -10.96119216345999803 ) ) ;
#4182=CARTESIAN_POINT ( 'NONE',  ( -5.393290222407999934, -77.91540636460800329, -11.03214393298000040 ) ) ;
#4196=CARTESIAN_POINT ( 'NONE',  ( 8.145694891731999121, -77.83223865415499176, -7.439717004853999782 ) ) ;
#4200=CARTESIAN_POINT ( 'NONE',  ( -4.019809786096000259, -79.10248417168200774, 10.47183077952999852 ) ) ;
#4217=EDGE_LOOP ( 'NONE', ( #23361, #54592, #1307, #38166, #34155, #25462, #27092, #36877, #27817, #27219, #29425 ) ) ;
#4218=CARTESIAN_POINT ( 'NONE',  ( 1.519276649035000037, -79.23866123649499116, 12.34025290414999887 ) ) ;
#4220=CARTESIAN_POINT ( 'NONE',  ( -5.974663857816401524, -78.02206841552093408, 8.936645035771457302 ) ) ;
#4225=CARTESIAN_POINT ( 'NONE',  ( 6.244078553291731559, -80.92595668623671656, 8.750503958027614715 ) ) ;
#4228=CARTESIAN_POINT ( 'NONE',  ( -6.686799317902000439, -76.89782152666799675, -9.062045808939998892 ) ) ;
#4230=CARTESIAN_POINT ( 'NONE',  ( 2.042758677500000175, -81.03081043471520672, -10.95189639700000050 ) ) ;
#4233=EDGE_CURVE ( 'NONE', #46084, #55147, #40190, .T. ) ;
#4247=EDGE_CURVE ( 'NONE', #49218, #15698, #10038, .T. ) ;
#4249=CARTESIAN_POINT ( 'NONE',  ( -0.8202502003661000796, -77.32800251553000237, -11.11673469052999863 ) ) ;
#4255=CARTESIAN_POINT ( 'NONE',  ( 0.04941934297688648642, -80.22561524380986953, -10.74974344490763656 ) ) ;
#4257=CARTESIAN_POINT ( 'NONE',  ( 9.454069809452303019, -79.14512987373443309, 6.036735293332626817 ) ) ;
#4259=AXIS2_PLACEMENT_3D ( 'NONE', #57813, #39517, #26225 ) ;
#4261=CARTESIAN_POINT ( 'NONE',  ( -1.478754609759999950, -78.43772245792399644, -10.94487265352999827 ) ) ;
#4263=ORIENTED_EDGE ( 'NONE', *, *, #16967, .F. ) ;
#4272=CARTESIAN_POINT ( 'NONE',  ( 4.703593957913000168, -79.48108495741900015, 9.978874598900000947 ) ) ;
#4279=ORIENTED_EDGE ( 'NONE', *, *, #2481, .F. ) ;
#4288=MECHANICAL_DESIGN_GEOMETRIC_PRESENTATION_REPRESENTATION('',(#23168),#56180);
#4289=CARTESIAN_POINT ( 'NONE',  ( 2.042225293701000144, -76.31900208490598914, 10.80792172197000056 ) ) ;
#4296=CARTESIAN_POINT ( 'NONE',  ( -8.418594644163000851, -80.95952068081420805, -7.485750452785000064 ) ) ;
#4304=ADVANCED_FACE ( 'NONE', ( #1070, #19058 ), #37046, .T. ) ;
#4321=CARTESIAN_POINT ( 'NONE',  ( -0.8545357605647209143, -77.21876371591302757, -10.72076371046810017 ) ) ;
#4324=VERTEX_POINT ( 'NONE', #7793 ) ;
#4325=EDGE_LOOP ( 'NONE', ( #27413, #52065, #13250, #55978 ) ) ;
#4330=CARTESIAN_POINT ( 'NONE',  ( 0.4872551020249000220, -77.56291771239200727, 12.03986520427999984 ) ) ;
#4331=EDGE_CURVE ( 'NONE', #38464, #40725, #54158, .T. ) ;
#4333=CIRCLE ( 'NONE', #43117, 12.50000000000000000 ) ;
#4339=ORIENTED_EDGE ( 'NONE', *, *, #16382, .T. ) ;
#4343=CARTESIAN_POINT ( 'NONE',  ( -11.05835115351384879, -79.80000000000001137, -4.525376038907399590 ) ) ;
#4353=CARTESIAN_POINT ( 'NONE',  ( -10.07979664880000037, -76.97175206120299151, 3.736335038366999761 ) ) ;
#4362=CARTESIAN_POINT ( 'NONE',  ( 0.000000000000000000, -92.79999999999999716, 0.000000000000000000 ) ) ;
#4371=CARTESIAN_POINT ( 'NONE',  ( 10.47129194184999967, -78.29940181198600158, 3.086650459461000473 ) ) ;
#4373=CARTESIAN_POINT ( 'NONE',  ( 11.54375705602000046, -77.66559881290099554, -3.837213001227999687 ) ) ;
#4382=CARTESIAN_POINT ( 'NONE',  ( -1.100349016362999865, -80.25828634263528727, -11.11813777798999858 ) ) ;
#4387=CARTESIAN_POINT ( 'NONE',  ( 4.013660496580000903, -78.55580284730699248, -10.47417304634999979 ) ) ;
#4405=FILL_AREA_STYLE ('',( #22407 ) ) ;
#4407=ORIENTED_EDGE ( 'NONE', *, *, #46423, .F. ) ;
#4409=CARTESIAN_POINT ( 'NONE',  ( -1.996166675347000208, -76.07957723391299965, 11.82412830296999928 ) ) ;
#4414=VECTOR ( 'NONE', #23046, 1000.000000000000000 ) ;
#4419=CARTESIAN_POINT ( 'NONE',  ( 0.5473670387515998659, -76.87888519345946747, -11.20350390113000039 ) ) ;
#4422=CARTESIAN_POINT ( 'NONE',  ( -0.4146318973825999787, -79.52374057552499664, -11.20920117498000046 ) ) ;
#4437=CARTESIAN_POINT ( 'NONE',  ( 10.75000000000000000, -79.75000000000000000, 0.000000000000000000 ) ) ;
#4438=CARTESIAN_POINT ( 'NONE',  ( 4.782478426736999744, -79.58994887379353145, 10.14623135401999932 ) ) ;
#4447=CARTESIAN_POINT ( 'NONE',  ( 6.891697027498000061, -78.75057898155800729, -9.743716654505998775 ) ) ;
#4452=CARTESIAN_POINT ( 'NONE',  ( 10.91479203715999979, -80.27508423127190440, -0.2066369003937000015 ) ) ;
#4463=CARTESIAN_POINT ( 'NONE',  ( 8.082813797676999812, -77.12536394690199870, -8.776523399436001682 ) ) ;
#4465=FACE_OUTER_BOUND ( 'NONE', #31696, .T. ) ;
#4468=CARTESIAN_POINT ( 'NONE',  ( 11.07171638148000170, -78.94961247579199437, -1.292941197001999942 ) ) ;
#4472=B_SPLINE_CURVE_WITH_KNOTS ( 'NONE', 3,
 ( #58362, #31174, #816, #45086, #27636, #22641, #45678, #23223, #41227, #54809, #40353, #22930, #14351, #49215, #48923, #8764, #242, #17625, #44483, #4034, #22338, #31471, #22040 ),
 .UNSPECIFIED., .F., .F.,
 ( 4, 2, 2, 1, 2, 2, 2, 2, 2, 2, 2, 4 ),
 ( 0.2857074366539503751, 0.3749940070722066476, 0.4196372922813347284, 0.4642805774904628646, 0.5089238626995910009, 0.5535671479087190816, 0.6428537183269752431, 0.7321402887452314046, 0.8214268591634875660, 0.9107134295817437275, 0.9553567147908719193, 1.000000000000000000 ),
 .UNSPECIFIED. ) ;
#4477=CARTESIAN_POINT ( 'NONE',  ( 8.990136242696999958, -79.13622555867699759, 8.365012251980999736 ) ) ;
#4483=CARTESIAN_POINT ( 'NONE',  ( 10.47020627418438643, -78.27083333333332860, 2.813789756862283387 ) ) ;
#4491=ORIENTED_EDGE ( 'NONE', *, *, #56196, .T. ) ;
#4498=CARTESIAN_POINT ( 'NONE',  ( 10.12058791103999944, -79.48379297370699703, 4.836508133599999759 ) ) ;
#4515=CARTESIAN_POINT ( 'NONE',  ( -1.810985506639999798, -79.76004069920800532, 12.30075622849999917 ) ) ;
#4516=CARTESIAN_POINT ( 'NONE',  ( 7.350255374610999759, -76.45613051119899239, -8.990260894034001637 ) ) ;
#4517=CARTESIAN_POINT ( 'NONE',  ( -6.285277716731378028, -78.02485450714230808, 8.721419318336506521 ) ) ;
#4518=CARTESIAN_POINT ( 'NONE',  ( 2.956870837876000468, -78.98874476440199999, 11.44999256673999888 ) ) ;
#4521=DIRECTION ( 'NONE',  ( -3.552713678800000476E-14, -1.000000000000000000, 1.317464655887999919E-13 ) ) ;
#4524=CARTESIAN_POINT ( 'NONE',  ( 1.648069335750886433, -80.96312284482743848, 10.62269281186031655 ) ) ;
#4527=CARTESIAN_POINT ( 'NONE',  ( 10.94776161156000072, -77.15620299209300015, 2.097883759165000139 ) ) ;
#4529=CARTESIAN_POINT ( 'NONE',  ( 10.87801983317999976, -80.69582220907369674, -1.798845711797000035 ) ) ;
#4531=CARTESIAN_POINT ( 'NONE',  ( 3.089702623610774967, -78.34792614711045644, -10.47025075772299374 ) ) ;
#4535=CARTESIAN_POINT ( 'NONE',  ( 1.508420534579999917, -77.56258324042499908, 11.11497989572000122 ) ) ;
#4541=CARTESIAN_POINT ( 'NONE',  ( -10.79468190574739594, -76.05000000000001137, 4.801183946204664821 ) ) ;
#4545=CARTESIAN_POINT ( 'NONE',  ( -7.835303970625000503, -78.21281986999699143, 8.089621514298000804 ) ) ;
#4553=CARTESIAN_POINT ( 'NONE',  ( -10.34340836277019449, -78.81829375771278023, 4.339989908386851170 ) ) ;
#4559=CARTESIAN_POINT ( 'NONE',  ( -11.13698119474000059, -79.89450301542969157, -0.4714344481541999921 ) ) ;
#4583=CARTESIAN_POINT ( 'NONE',  ( 10.12567350656000009, -76.18657555664699998, 4.748118780173999909 ) ) ;
#4588=B_SPLINE_CURVE_WITH_KNOTS ( 'NONE', 3,
 ( #52525, #12367, #20653, #48396, #17372, #47830, #53102, #12082, #25077, #7933, #25934, #21795, #12651, #30644, #30064, #25646, #39799, #7361 ),
 .UNSPECIFIED., .F., .F.,
 ( 4, 2, 2, 2, 2, 2, 2, 2, 4 ),
 ( 0.000000000000000000, 0.1250000000000000000, 0.2500000000000000000, 0.3749999999999999445, 0.4999999999999998890, 0.6249999999999998890, 0.7499999999999998890, 0.8749999999999998890, 1.000000000000000000 ),
 .UNSPECIFIED. ) ;
#4589=CARTESIAN_POINT ( 'NONE',  ( -10.38689113780999840, -77.00541705171700357, 2.826523783570000337 ) ) ;
#4591=LINE ( 'NONE', #197, #1972 ) ;
#4594=CARTESIAN_POINT ( 'NONE',  ( -0.9849936891751999157, -80.95192749954530598, -11.22225356808999841 ) ) ;
#4624=CARTESIAN_POINT ( 'NONE',  ( 0.03815395216748320578, -77.22536730000003047, -10.74989112016262993 ) ) ;
#4630=CARTESIAN_POINT ( 'NONE',  ( -1.548298113504216866, -76.12161458261024904, -11.82161455805163719 ) ) ;
#4631=CARTESIAN_POINT ( 'NONE',  ( -2.981173517641313886, -80.39728512301172714, 10.37580895950596904 ) ) ;
#4633=CARTESIAN_POINT ( 'NONE',  ( 3.237243043699999934, -78.77026847289599232, -11.48719983142999901 ) ) ;
#4647=CARTESIAN_POINT ( 'NONE',  ( -11.02098641988770034, -79.79999999999999716, -4.612498697062771491 ) ) ;
#4654=CARTESIAN_POINT ( 'NONE',  ( -1.835125225091999823, -78.03723861434511377, 11.83842809849000410 ) ) ;
#4656=CARTESIAN_POINT ( 'NONE',  ( 5.246383657897999875, -77.06100733245999379, -10.79237965019999912 ) ) ;
#4675=CARTESIAN_POINT ( 'NONE',  ( -3.419437234775999812, -78.62623792800799549, -10.36738907398999920 ) ) ;
#4676=CARTESIAN_POINT ( 'NONE',  ( -0.08732773870155000062, -78.24897531865799749, 12.27958277169999945 ) ) ;
#4679=CARTESIAN_POINT ( 'NONE',  ( -12.00000000000000000, -78.89999999999999147, -1.868256502752000067E-14 ) ) ;
#4683=CARTESIAN_POINT ( 'NONE',  ( 0.3693169358421000137, -79.94575047619699149, 11.04974602993000055 ) ) ;
#4693=VERTEX_POINT ( 'NONE', #34780 ) ;
#4697=DIRECTION ( 'NONE',  ( 0.000000000000000000, -1.000000000000000000, 0.000000000000000000 ) ) ;
#4710=CARTESIAN_POINT ( 'NONE',  ( 9.371326875074000640, -76.81784402283000190, -7.865448804155000140 ) ) ;
#4711=CARTESIAN_POINT ( 'NONE',  ( -9.133843623092825936, -78.64447737370456082, -5.680053951677152213 ) ) ;
#4714=ORIENTED_EDGE ( 'NONE', *, *, #32564, .F. ) ;
#4718=CARTESIAN_POINT ( 'NONE',  ( -10.48543666025109111, -78.84166666666665435, -6.043427764450793660 ) ) ;
#4724=VERTEX_POINT ( 'NONE', #16506 ) ;
#4746=CARTESIAN_POINT ( 'NONE',  ( 3.281228840419999848, -79.67588468523199197, -10.41195962760999905 ) ) ;
#4754=CARTESIAN_POINT ( 'NONE',  ( -12.29672256689999976, -75.88792199503599534, -2.267527262250000231 ) ) ;
#4756=CARTESIAN_POINT ( 'NONE',  ( -6.417398495783289469, -76.92555371511903672, 8.714208636181064449 ) ) ;
#4759=CARTESIAN_POINT ( 'NONE',  ( 10.67847671903000162, -80.05232057427369341, 3.578272902691999491 ) ) ;
#4767=CARTESIAN_POINT ( 'NONE',  ( -2.251292830498186071, -76.39166666666665151, 10.57172952794456933 ) ) ;
#4771=CARTESIAN_POINT ( 'NONE',  ( 10.74999999999999645, -79.26041666666667140, 1.407171709420451666 ) ) ;
#4772=CARTESIAN_POINT ( 'NONE',  ( 8.596418555780418913, -78.30208333333331439, 6.606377239730356621 ) ) ;
#4782=CARTESIAN_POINT ( 'NONE',  ( 1.483539930421000186, -77.50540253813299785, 10.93164414240999882 ) ) ;
#4786=CARTESIAN_POINT ( 'NONE',  ( 10.05828973332000054, -78.97961832394499027, -4.964767691657000270 ) ) ;
#4807=CARTESIAN_POINT ( 'NONE',  ( -11.92000176286999924, -78.99177042599900744, 2.600513710866999784 ) ) ;
#4809=CARTESIAN_POINT ( 'NONE',  ( -9.323141007194999830, -76.18968473043899792, -6.517165561429999698 ) ) ;
#4810=CARTESIAN_POINT ( 'NONE',  ( -4.144776331383936530, -78.00651457564580937, 9.918828337007836282 ) ) ;
#4811=CARTESIAN_POINT ( 'NONE',  ( 1.720939166139000109, -77.33834334083999806, -11.69973432676000158 ) ) ;
#4814=CARTESIAN_POINT ( 'NONE',  ( -9.393376654192294950, -79.05850173436991213, 5.414072594118386483 ) ) ;
#4817=CARTESIAN_POINT ( 'NONE',  ( 5.710891535341052538, -80.93086402315771011, 9.111465207288862445 ) ) ;
#4820=CARTESIAN_POINT ( 'NONE',  ( 0.1384068119873000102, -77.26514836410099463, 11.14609546546000018 ) ) ;
#4821=CARTESIAN_POINT ( 'NONE',  ( 9.596002108778145967, -78.10208333333332575, 7.374560639699001996 ) ) ;
#4822=CARTESIAN_POINT ( 'NONE',  ( -6.536208127187000727, -80.81602894668615988, 9.021928177040001273 ) ) ;
#4827=CARTESIAN_POINT ( 'NONE',  ( -11.21668965365999959, -77.69876495543400097, -0.06311738993059998193 ) ) ;
#4829=CARTESIAN_POINT ( 'NONE',  ( 9.393285425842218928, -76.89183432704838594, 5.414042684532392791 ) ) ;
#4831=CARTESIAN_POINT ( 'NONE',  ( -8.779106447692180737, -78.54927823582298174, -6.259569139016079475 ) ) ;
#4835=CARTESIAN_POINT ( 'NONE',  ( 5.137083998358000336, -77.31100733245999379, -10.56753840748999984 ) ) ;
#4840=CARTESIAN_POINT ( 'NONE',  ( -10.97713377773999888, -78.29452889900299795, -2.517240518847000175 ) ) ;
#4847=CARTESIAN_POINT ( 'NONE',  ( -10.02265812545943469, -80.13001055447919896, -3.947397417359383986 ) ) ;
#4850=ORIENTED_EDGE ( 'NONE', *, *, #54858, .F. ) ;
#4853=CARTESIAN_POINT ( 'NONE',  ( 0.000000000000000000, -79.79999999999999716, 0.000000000000000000 ) ) ;
#4854=CARTESIAN_POINT ( 'NONE',  ( 7.759949366729999909, -79.07741272537499810, -8.002361301306001096 ) ) ;
#4881=CARTESIAN_POINT ( 'NONE',  ( 9.854749457207999441, -76.31148332335199314, 4.621077397111999829 ) ) ;
#4884=CARTESIAN_POINT ( 'NONE',  ( 6.985849709488999970, -81.01212287155250635, -8.837815942395002011 ) ) ;
#4890=FACE_OUTER_BOUND ( 'NONE', #42330, .T. ) ;
#4891=CARTESIAN_POINT ( 'NONE',  ( -6.711381441964999972, -80.32746927473799303, 9.048015653393999713 ) ) ;
#4897=DIRECTION ( 'NONE',  ( -1.000000000000000000, 0.000000000000000000, 0.000000000000000000 ) ) ;
#4901=CARTESIAN_POINT ( 'NONE',  ( -2.714236658744829445, -79.49531908340782138, 10.40320972029338442 ) ) ;
#4906=CARTESIAN_POINT ( 'NONE',  ( 6.158633396698134810, -80.07777475630253150, 9.129463103461906925 ) ) ;
#4916=CARTESIAN_POINT ( 'NONE',  ( -2.546404564821087124, -77.20613843984394009, -10.44401662958821220 ) ) ;
#4917=CARTESIAN_POINT ( 'NONE',  ( 11.99999999999999822, -79.05670863885251265, 1.011638905658235110 ) ) ;
#4919=ORIENTED_EDGE ( 'NONE', *, *, #2639, .F. ) ;
#4920=CARTESIAN_POINT ( 'NONE',  ( -11.22206352833000054, -79.73100370980900209, -4.332716936452000844 ) ) ;
#4921=CARTESIAN_POINT ( 'NONE',  ( -8.625997596412716462, -80.44864256150583515, 6.491299759919599843 ) ) ;
#4924=CARTESIAN_POINT ( 'NONE',  ( 0.9683650813416999625, -78.32253854425700013, -12.01074688531000056 ) ) ;
#4925=VERTEX_POINT ( 'NONE', #9391 ) ;
#4935=LINE ( 'NONE', #30897, #51015 ) ;
#4936=B_SPLINE_CURVE_WITH_KNOTS ( 'NONE', 3,
 ( #14359, #9070, #17930, #32358, #31777, #27056, #50402, #45093, #8771, #49818, #44792, #45393, #9951, #5507, #4343, #4647, #2551, #6091, #41820, #33533, #15538, #47440, #5799, #10834, #33818, #37677, #11412, #55396, #51857, #32942, #24400, #23805, #10239, #20553, #10535, #29392, #29106, #33236, #2266, #42702, #15830, #1395, #24100, #38549, #15243, #50984, #51280, #24973, #6969, #56281, #42994, #6681, #14650, #19676, #28518, #20266, #38257, #42120, #14942 ),
 .UNSPECIFIED., .F., .F.,
 ( 4, 1, 1, 1, 1, 1, 2, 2, 1, 1, 1, 1, 1, 2, 2, 1, 2, 2, 1, 1, 1, 2, 2, 1, 1, 2, 2, 1, 2, 2, 1, 1, 2, 2, 1, 1, 1, 1, 2, 2, 4 ),
 ( 0.000000000000000000, 0.06250000000000048572, 0.09375000000000070777, 0.1093750000000008049, 0.1171875000000008465, 0.1210937500000008604, 0.1230468750000009021, 0.1250000000000009437, 0.1875000000000023037, 0.2187500000000028866, 0.2343750000000032196, 0.2421875000000033862, 0.2460937500000035250, 0.2480468750000035805, 0.2500000000000036637, 0.3125000000000029421, 0.3437500000000026090, 0.3750000000000022760, 0.4375000000000016098, 0.4687500000000012212, 0.4843750000000010547, 0.4921875000000009437, 0.5000000000000007772, 0.5625000000000007772, 0.5937500000000008882, 0.6093750000000008882, 0.6250000000000008882, 0.6875000000000006661, 0.7187500000000006661, 0.7500000000000006661, 0.7812500000000006661, 0.7968750000000006661, 0.8046875000000005551, 0.8125000000000005551, 0.8437500000000004441, 0.8593750000000003331, 0.8671875000000003331, 0.8710937500000003331, 0.8730468750000003331, 0.8750000000000003331, 1.000000000000000000 ),
 .UNSPECIFIED. ) ;
#4956=CARTESIAN_POINT ( 'NONE',  ( -7.769589423449606791, -78.16171743685177375, -7.614127194111606656 ) ) ;
#4965=EDGE_CURVE ( 'NONE', #12394, #36999, #36246, .T. ) ;
#4967=CARTESIAN_POINT ( 'NONE',  ( 7.859834628577000437, -80.32823171464259815, -7.940198685096999220 ) ) ;
#4970=CARTESIAN_POINT ( 'NONE',  ( -10.86658628928999981, -76.85383371392200047, -2.781249891074999869 ) ) ;
#4974=CARTESIAN_POINT ( 'NONE',  ( -12.00000000000000000, -76.79999999999999716, 1.164316068523999942E-14 ) ) ;
#4977=CARTESIAN_POINT ( 'NONE',  ( 8.899186938125001944, -76.04999999999999716, 6.465637775217000005 ) ) ;
#4979=CARTESIAN_POINT ( 'NONE',  ( 0.000000000000000000, -90.29999999999999716, 0.000000000000000000 ) ) ;
#4997=CARTESIAN_POINT ( 'NONE',  ( 11.67908924396999915, -76.96753656385298825, 4.023272830065000250 ) ) ;
#5006=CARTESIAN_POINT ( 'NONE',  ( 3.140974612311377090, -78.94583333333332575, -11.68767212001978528 ) ) ;
#5029=CARTESIAN_POINT ( 'NONE',  ( 7.851705946354000432, -77.18019320671699290, -9.048036745432998629 ) ) ;
#5031=CARTESIAN_POINT ( 'NONE',  ( -11.55487901120999972, -78.03174834697500728, -3.417680896482000019 ) ) ;
#5035=CARTESIAN_POINT ( 'NONE',  ( 8.589798209762999903, -78.65488561575499205, -6.922213596449000583 ) ) ;
#5039=EDGE_CURVE ( 'NONE', #36154, #41200, #46005, .T. ) ;
#5044=CARTESIAN_POINT ( 'NONE',  ( -2.813789756862300262, -77.39583333333334281, 10.47020627418438465 ) ) ;
#5048=CARTESIAN_POINT ( 'NONE',  ( -12.47910600135000081, -76.37844759300099895, -0.7911314731844000248 ) ) ;
#5051=ORIENTED_EDGE ( 'NONE', *, *, #4039, .T. ) ;
#5052=CARTESIAN_POINT ( 'NONE',  ( 7.942219812765999087, -79.58930274324299603, 7.984679643171000762 ) ) ;
#5070=CARTESIAN_POINT ( 'NONE',  ( 7.655285058836605039, -78.78807752846175561, -7.547175273370277715 ) ) ;
#5075=CIRCLE ( 'NONE', #55992, 11.70000000000000107 ) ;
#5076=CARTESIAN_POINT ( 'NONE',  ( 6.099615176083999835, -78.31341404718699550, -9.019941877331000057 ) ) ;
#5079=CARTESIAN_POINT ( 'NONE',  ( -10.86803167256632463, -77.58446068609639212, -5.040424477369018774 ) ) ;
#5080=CARTESIAN_POINT ( 'NONE',  ( -10.34326456654000026, -78.73449123692898866, 4.339929572939999147 ) ) ;
#5081=CARTESIAN_POINT ( 'NONE',  ( 8.562542432403372317, -81.00000000000002842, 6.777005483380555084 ) ) ;
#5097=CARTESIAN_POINT ( 'NONE',  ( 12.50000000000000000, -91.29999999999999716, 2.555046452191000376E-12 ) ) ;
#5100=CARTESIAN_POINT ( 'NONE',  ( -9.739450257827000357, -78.99356062328099881, -7.539835367685000733 ) ) ;
#5101=CARTESIAN_POINT ( 'NONE',  ( 0.1598674175986999901, -76.08275625893899985, 11.49285586031999884 ) ) ;
#5102=CARTESIAN_POINT ( 'NONE',  ( 2.414752746249941406, -77.95724855646152207, 10.49752381153813907 ) ) ;
#5103=CARTESIAN_POINT ( 'NONE',  ( 10.69384760718000038, -78.34668429937299550, -5.399785902169999652 ) ) ;
#5107=CARTESIAN_POINT ( 'NONE',  ( 0.000000000000000000, -91.29999999999999716, 0.000000000000000000 ) ) ;
#5108=CARTESIAN_POINT ( 'NONE',  ( 3.268028314528707678, -80.95051983432966836, 10.24357525341220132 ) ) ;
#5111=CARTESIAN_POINT ( 'NONE',  ( 2.958310398169000432, -77.53751179411899841, -10.74723220921999989 ) ) ;
#5112=CARTESIAN_POINT ( 'NONE',  ( -12.17466003208999936, -76.63951734500820123, 1.612538369963999907 ) ) ;
#5113=CARTESIAN_POINT ( 'NONE',  ( 1.937333205045999929, -80.25222754060989416, 10.97105737937000036 ) ) ;
#5121=CARTESIAN_POINT ( 'NONE',  ( 7.155101792066000499, -78.44746208375599394, -8.354909834651998324 ) ) ;
#5122=CARTESIAN_POINT ( 'NONE',  ( 0.000000000000000000, -76.00000000000000000, 0.000000000000000000 ) ) ;
#5125=CARTESIAN_POINT ( 'NONE',  ( 3.042547531669000271, -78.64783470746900207, -10.31045122763999977 ) ) ;
#5130=EDGE_CURVE ( 'NONE', #33417, #3715, #16755, .T. ) ;
#5142=CARTESIAN_POINT ( 'NONE',  ( 10.63213186872000016, -78.54666782993099616, -3.713725309742000213 ) ) ;
#5144=VERTEX_POINT ( 'NONE', #30545 ) ;
#5152=CARTESIAN_POINT ( 'NONE',  ( -10.48543666025109111, -76.34166666662416389, -6.043427764450793660 ) ) ;
#5156=ORIENTED_EDGE ( 'NONE', *, *, #30225, .F. ) ;
#5157=EDGE_LOOP ( 'NONE', ( #11690, #54004, #49135, #2070 ) ) ;
#5171=CARTESIAN_POINT ( 'NONE',  ( -8.418594644163000851, -80.82394357426177578, -7.485750452785000064 ) ) ;
#5176=CARTESIAN_POINT ( 'NONE',  ( 7.189039685305539606, -77.47583944371665154, -9.673072753243907584 ) ) ;
#5188=CARTESIAN_POINT ( 'NONE',  ( -6.313152452412044369, -79.52497619356374514, 8.700938145767349141 ) ) ;
#5205=CARTESIAN_POINT ( 'NONE',  ( -3.395352835590720098, -77.19953567266439620, -10.19974753772885201 ) ) ;
#5211=ORIENTED_EDGE ( 'NONE', *, *, #27920, .T. ) ;
#5212=CARTESIAN_POINT ( 'NONE',  ( 1.730980777285999972, -77.32779697871899316, -11.76800180821999930 ) ) ;
#5217=B_SPLINE_CURVE_WITH_KNOTS ( 'NONE', 3,
 ( #46347, #55475, #14722, #4718, #41311, #40730, #9437, #13856, #321, #18298, #5006, #36293, #54315, #31851, #50474, #27716, #5294, #49893 ),
 .UNSPECIFIED., .F., .F.,
 ( 4, 2, 2, 2, 2, 2, 2, 2, 4 ),
 ( 0.000000000000000000, 0.1250000000000000000, 0.2500000000000000000, 0.3750000000000000000, 0.5000000000000000000, 0.6250000000000000000, 0.7500000000000000000, 0.8750000000000000000, 1.000000000000000000 ),
 .UNSPECIFIED. ) ;
#5218=CARTESIAN_POINT ( 'NONE',  ( -9.596002108778193929, -78.74791666666664014, 7.374560639698935383 ) ) ;
#5228=CARTESIAN_POINT ( 'NONE',  ( -8.075725583014000009, -76.32689981197398765, -7.736700848913999451 ) ) ;
#5230=EDGE_CURVE ( 'NONE', #32124, #47573, #32202, .T. ) ;
#5232=CARTESIAN_POINT ( 'NONE',  ( -9.871315929017001167, -76.28387572403700290, 5.351714737855999715 ) ) ;
#5240=CARTESIAN_POINT ( 'NONE',  ( 0.000000000000000000, -75.15999999999999659, 0.000000000000000000 ) ) ;
#5247=DIRECTION ( 'NONE',  ( 0.000000000000000000, 1.000000000000000000, 0.000000000000000000 ) ) ;
#5259=CARTESIAN_POINT ( 'NONE',  ( 5.125497890974998860, -79.28376034395300564, -10.76871041769000037 ) ) ;
#5261=CARTESIAN_POINT ( 'NONE',  ( -10.83119716622999995, -80.18612266303370006, 3.182336190940000087 ) ) ;
#5270=AXIS2_PLACEMENT_3D ( 'NONE', #30124, #2995, #49837 ) ;
#5277=ORIENTED_EDGE ( 'NONE', *, *, #7186, .T. ) ;
#5286=CARTESIAN_POINT ( 'NONE',  ( -1.977101394398999679, -76.01185016949999351, 11.71119668716000106 ) ) ;
#5294=CARTESIAN_POINT ( 'NONE',  ( 12.00000000000000888, -79.03958333333332575, -1.570796326794872577 ) ) ;
#5298=EDGE_LOOP ( 'NONE', ( #6954, #18723, #25174, #2641, #39990, #4018 ) ) ;
#5314=CARTESIAN_POINT ( 'NONE',  ( -10.34326456654000026, -78.71838589773552997, 4.339929572939999147 ) ) ;
#5323=CARTESIAN_POINT ( 'NONE',  ( -11.93030759001999996, -78.52007602460300006, -1.692197530282999907 ) ) ;
#5326=CARTESIAN_POINT ( 'NONE',  ( 11.03163745116999905, -78.70935830175899639, 0.06858965353743999571 ) ) ;
#5333=CARTESIAN_POINT ( 'NONE',  ( 12.16540687204999927, -76.60484402282999383, -2.890821896307000038 ) ) ;
#5337=EDGE_LOOP ( 'NONE', ( #38765, #37194, #29093, #6430 ) ) ;
#5338=CARTESIAN_POINT ( 'NONE',  ( -10.97184146967999929, -79.19473956280799598, 1.968068935562000243 ) ) ;
#5340=CARTESIAN_POINT ( 'NONE',  ( 5.413904038987143785, -79.83333333333334281, 9.393203674808290771 ) ) ;
#5356=CARTESIAN_POINT ( 'NONE',  ( 9.234857099017842685, -78.80734080730690039, -5.504304055585024003 ) ) ;
#5364=CARTESIAN_POINT ( 'NONE',  ( 11.95265301635149946, -78.80527988016636698, 0.8087635557727725910 ) ) ;
#5365=CARTESIAN_POINT ( 'NONE',  ( 3.632329907060999563, -80.18225450229719797, 10.45854222826000068 ) ) ;
#5366=CARTESIAN_POINT ( 'NONE',  ( 10.44969936162916646, -81.00000000000000000, 3.411603317218904863 ) ) ;
#5375=CARTESIAN_POINT ( 'NONE',  ( -8.596418555780466875, -80.94791666666665719, 6.606377239730298001 ) ) ;
#5386=CARTESIAN_POINT ( 'NONE',  ( 9.562223978213696185, -77.88793088717281421, 4.911682316942298065 ) ) ;
#5394=CARTESIAN_POINT ( 'NONE',  ( 10.22699339414000086, -77.67369350912798609, 4.434321446068000050 ) ) ;
#5396=CARTESIAN_POINT ( 'NONE',  ( -10.73991933103999941, -80.86972431869342870, 2.961644346888999912 ) ) ;
#5401=CARTESIAN_POINT ( 'NONE',  ( -7.803863155890000236, -78.20233499673999233, 8.057160196619001624 ) ) ;
#5404=CARTESIAN_POINT ( 'NONE',  ( -10.31421052434999908, -76.72175206120299151, 3.823226550887000030 ) ) ;
#5414=CARTESIAN_POINT ( 'NONE',  ( -11.68767212001979061, -79.32083333333332575, -3.140974612311365988 ) ) ;
#5417=CARTESIAN_POINT ( 'NONE',  ( -10.75000000000000000, -80.09999999999999432, -1.711887504597999906E-14 ) ) ;
#5422=CARTESIAN_POINT ( 'NONE',  ( 11.14673908614000020, -78.64163123734599026, 0.06930530262389000828 ) ) ;
#5424=VERTEX_POINT ( 'NONE', #1610 ) ;
#5457=CARTESIAN_POINT ( 'NONE',  ( -11.03620408507000050, -80.28218522619640396, -2.260839449595000161 ) ) ;
#5462=CARTESIAN_POINT ( 'NONE',  ( -6.043427764450833628, -78.31666666666667709, 10.48543666025107335 ) ) ;
#5472=CARTESIAN_POINT ( 'NONE',  ( -1.200332545804832840, -79.48406602089589512, 10.68275685977173950 ) ) ;
#5483=CARTESIAN_POINT ( 'NONE',  ( 5.246383657897999875, -77.06100733245999379, -10.79237965019999912 ) ) ;
#5486=CARTESIAN_POINT ( 'NONE',  ( -7.264472637402048960, -77.16596736302702197, -7.925599033090998446 ) ) ;
#5487=CARTESIAN_POINT ( 'NONE',  ( 10.98749645531832542, -79.08354319426250356, 4.929334125397528688 ) ) ;
#5490=CARTESIAN_POINT ( 'NONE',  ( -8.850953919802000414, -79.69309878738100394, -8.146641040006999290 ) ) ;
#5491=CARTESIAN_POINT ( 'NONE',  ( -6.525519130240628130, -80.42663223072267442, 8.600139951612055356 ) ) ;
#5499=CARTESIAN_POINT ( 'NONE',  ( 14.00000000000000000, -80.90000000000000568, 0.000000000000000000 ) ) ;
#5505=CARTESIAN_POINT ( 'NONE',  ( 10.75000000000000000, -80.75000000000000000, 3.489821576044999869E-14 ) ) ;
#5507=CARTESIAN_POINT ( 'NONE',  ( -11.13124813254851198, -79.79999999999998295, -4.350558907888798288 ) ) ;
#5510=CARTESIAN_POINT ( 'NONE',  ( -10.99972769911000015, -76.25165398600699973, 2.019869862886000345 ) ) ;
#5512=CARTESIAN_POINT ( 'NONE',  ( -4.819527309429000539, -76.23371184005799250, 10.14178905882999970 ) ) ;
#5540=CARTESIAN_POINT ( 'NONE',  ( -4.697326221550000014, -81.11872762313059582, 9.999795703097998256 ) ) ;
#5543=CARTESIAN_POINT ( 'NONE',  ( -8.649885944100999424, -77.95660330126699478, -7.141259254888000285 ) ) ;
#5544=FACE_OUTER_BOUND ( 'NONE', #24892, .T. ) ;
#5557=EDGE_CURVE ( 'NONE', #37074, #54955, #30731, .T. ) ;
#5561=CARTESIAN_POINT ( 'NONE',  ( -10.52667135666000142, -78.78354445816799512, 6.323366929881999887 ) ) ;
#5564=EDGE_LOOP ( 'NONE', ( #42174, #13484, #45606, #15517, #9399 ) ) ;
#5567=B_SPLINE_CURVE_WITH_KNOTS ( 'NONE', 3,
 ( #15630, #30340, #39211, #57226 ),
 .UNSPECIFIED., .F., .F.,
 ( 4, 4 ),
 ( 0.000000000000000000, 1.000000000000000000 ),
 .UNSPECIFIED. ) ;
#5587=CARTESIAN_POINT ( 'NONE',  ( 4.297951556683999641, -76.71955760450698847, -11.50435740523999861 ) ) ;
#5592=CARTESIAN_POINT ( 'NONE',  ( 6.085790774524467928, -78.42088135606610422, -9.367230124943132452 ) ) ;
#5602=CARTESIAN_POINT ( 'NONE',  ( 9.201871282504999527, -77.81471382358499511, 7.779546039068999441 ) ) ;
#5604=ADVANCED_FACE ( 'NONE', ( #33460 ), #2669, .F. ) ;
#5607=CARTESIAN_POINT ( 'NONE',  ( 2.253937565478000060, -78.66813999416500280, -10.68151722998999986 ) ) ;
#5616=CARTESIAN_POINT ( 'NONE',  ( -11.46357413472999909, -76.34071485469600304, 4.994040814626000468 ) ) ;
#5621=CARTESIAN_POINT ( 'NONE',  ( -1.463640999337999959, -78.32317658674999450, -10.83301059047000159 ) ) ;
#5623=CARTESIAN_POINT ( 'NONE',  ( 10.49303003107499421, -79.76163707075535569, -5.474388617415005598 ) ) ;
#5634=EDGE_CURVE ( 'NONE', #8440, #38434, #38491, .T. ) ;
#5639=CARTESIAN_POINT ( 'NONE',  ( 8.425244479088499716, -78.79682508674252972, -6.676653465681916977 ) ) ;
#5640=CIRCLE ( 'NONE', #13173, 9.599999999999999645 ) ;
#5641=EDGE_LOOP ( 'NONE', ( #19344, #6143, #56917, #53309 ) ) ;
#5647=CARTESIAN_POINT ( 'NONE',  ( -2.472186688656227371, -77.15814173843004653, -11.94662027503587076 ) ) ;
#5648=CARTESIAN_POINT ( 'NONE',  ( -1.360231837983352676, -77.66584863236742819, -11.90251068871223339 ) ) ;
#5649=CARTESIAN_POINT ( 'NONE',  ( -11.19989528650999944, -78.76172757993099083, 0.6168112860373000661 ) ) ;
#5658=CARTESIAN_POINT ( 'NONE',  ( -1.570796326794884790, -77.51458333333334849, -12.00000000000000355 ) ) ;
#5670=CARTESIAN_POINT ( 'NONE',  ( 8.411888842866000360, -76.58712216313399779, 8.005707060120000662 ) ) ;
#5671=CARTESIAN_POINT ( 'NONE',  ( -0.1701304685956719354, -77.97633532982500526, 10.74867621670826878 ) ) ;
#5672=CARTESIAN_POINT ( 'NONE',  ( 10.46934363224000109, -77.42428757496500680, 5.823135730235999397 ) ) ;
#5676=CARTESIAN_POINT ( 'NONE',  ( 9.574567190152320606, -80.88771002875691352, 4.887542694105030172 ) ) ;
#5680=CARTESIAN_POINT ( 'NONE',  ( -9.244881144060999034, -76.93831224807900071, -6.227904302768000555 ) ) ;
#5682=CARTESIAN_POINT ( 'NONE',  ( 7.291278940103000039, -80.77636526708458575, 8.270696028970998981 ) ) ;
#5686=CARTESIAN_POINT ( 'NONE',  ( 2.787169241930258057, -80.45429007894077245, 10.40602097193850817 ) ) ;
#5687=CARTESIAN_POINT ( 'NONE',  ( 11.01642476345000077, -76.96338369438498717, 2.111041454437999842 ) ) ;
#5691=CARTESIAN_POINT ( 'NONE',  ( -0.2428027759546764197, -78.62319558955745435, -10.77942311248712315 ) ) ;
#5695=CARTESIAN_POINT ( 'NONE',  ( 0.000000000000000000, -75.15999999999999659, 0.000000000000000000 ) ) ;
#5704=CARTESIAN_POINT ( 'NONE',  ( -7.598611126932110160, -80.16299070835863461, -7.603773876929224684 ) ) ;
#5712=CARTESIAN_POINT ( 'NONE',  ( 9.221778727104000595, -79.66263030682299018, -6.054794091447999627 ) ) ;
#5719=EDGE_LOOP ( 'NONE', ( #47994, #31456, #30315 ) ) ;
#5725=CARTESIAN_POINT ( 'NONE',  ( 5.413904038987179312, -78.16666666666662877, -9.393203674808262349 ) ) ;
#5730=CARTESIAN_POINT ( 'NONE',  ( 0.3704480450335023711, -77.02746413819750160, -12.03686759590603650 ) ) ;
#5738=CARTESIAN_POINT ( 'NONE',  ( -10.00716890277074356, -77.34696047196747770, -6.699252482692385158 ) ) ;
#5743=CARTESIAN_POINT ( 'NONE',  ( 7.551392188974999975, -80.08153398617218954, 8.117862728809001283 ) ) ;
#5744=CARTESIAN_POINT ( 'NONE',  ( 1.570796326794857478, -76.66458333333332575, 12.00000000000000533 ) ) ;
#5745=CARTESIAN_POINT ( 'NONE',  ( 1.407187316041068392, -76.73555785001855156, -10.75055512959062121 ) ) ;
#5752=CARTESIAN_POINT ( 'NONE',  ( 2.854661674668000058E-14, -82.00000000000000000, 0.000000000000000000 ) ) ;
#5760=CARTESIAN_POINT ( 'NONE',  ( -2.508531238560355092, -79.49373965571280110, 10.45321017623470716 ) ) ;
#5772=DIRECTION ( 'NONE',  ( 0.000000000000000000, 1.000000000000000000, 4.440892098500000122E-14 ) ) ;
#5781=CARTESIAN_POINT ( 'NONE',  ( -5.092641036025000290, -79.54368063314299775, 10.89826376711000044 ) ) ;
#5782=DIRECTION ( 'NONE',  ( 1.000000000000000000, 0.000000000000000000, 0.000000000000000000 ) ) ;
#5786=CARTESIAN_POINT ( 'NONE',  ( -8.852102014390000662, -78.06490627187800158, 8.004735621704000437 ) ) ;
#5790=B_SPLINE_CURVE_WITH_KNOTS ( 'NONE', 3,
 ( #18494, #4917, #54515, #45368, #5487, #40637, #31160, #53931, #18785, #37065 ),
 .UNSPECIFIED., .F., .F.,
 ( 4, 2, 2, 2, 4 ),
 ( 0.000000000000000000, 0.2500000000000000000, 0.5000000000000000000, 0.7500000000000000000, 1.000000000000000000 ),
 .UNSPECIFIED. ) ;
#5799=CARTESIAN_POINT ( 'NONE',  ( -9.760280716455657313, -79.79999999999999716, -6.845562419370476270 ) ) ;
#5803=CARTESIAN_POINT ( 'NONE',  ( 5.380788203752000065, -76.10116233407198649, 9.804131929786001010 ) ) ;
#5826=CARTESIAN_POINT ( 'NONE',  ( -1.394284273676999808, -77.48935448679299043, -12.20048157021999913 ) ) ;
#5833=CARTESIAN_POINT ( 'NONE',  ( 0.3732109351705000244, -80.01347754060989814, 11.16625220509000016 ) ) ;
#5834=STYLED_ITEM ( 'NONE', ( #54305 ), #11003 ) ;
#5838=CARTESIAN_POINT ( 'NONE',  ( -10.17713110909000029, -76.86714958119398489, 4.716330562529999604 ) ) ;
#5839=CARTESIAN_POINT ( 'NONE',  ( 0.000000000000000000, -75.15999999999999659, 0.000000000000000000 ) ) ;
#5846=CARTESIAN_POINT ( 'NONE',  ( 11.22355342542000045, -80.45517816094930197, 0.9700744431168999427 ) ) ;
#5853=CARTESIAN_POINT ( 'NONE',  ( 12.13705548371000020, -79.01423986341698935, 0.8212409526314999875 ) ) ;
#5868=VECTOR ( 'NONE', #12097, 1000.000000000000000 ) ;
#5871=CARTESIAN_POINT ( 'NONE',  ( -10.23602088258210152, -76.67184350084455957, 3.794244288828453993 ) ) ;
#5881=CARTESIAN_POINT ( 'NONE',  ( -3.164411967817999827, -77.17036772586099858, -11.86639179494000018 ) ) ;
#5890=DIRECTION ( 'NONE',  ( 0.000000000000000000, -1.000000000000000000, 0.000000000000000000 ) ) ;
#5894=CARTESIAN_POINT ( 'NONE',  ( 0.9683650813416999625, -78.14026560866999205, -12.01074688531000056 ) ) ;
#5897=CARTESIAN_POINT ( 'NONE',  ( 10.26057445098000187, -78.80432170917399048, 3.727731092327000173 ) ) ;
#5899=VERTEX_POINT ( 'NONE', #19911 ) ;
#5907=CARTESIAN_POINT ( 'NONE',  ( 9.596002108778145967, -77.70208333333330586, 7.374560639699002884 ) ) ;
#5912=CARTESIAN_POINT ( 'NONE',  ( 6.907293935673000540, -79.09904856920998384, 8.895125352942999442 ) ) ;
#5921=CARTESIAN_POINT ( 'NONE',  ( -9.805777851055321293, -79.39025696075076155, -5.446864207918929779 ) ) ;
#5925=CARTESIAN_POINT ( 'NONE',  ( -10.75000000000000000, -81.00000000000000000, 2.851355842494999902E-13 ) ) ;
#5933=CARTESIAN_POINT ( 'NONE',  ( 9.931997526924730479, -78.81882101904967897, -4.113022196682803333 ) ) ;
#5938=B_SPLINE_CURVE_WITH_KNOTS ( 'NONE', 3,
 ( #48859, #13112, #18154, #5152, #39984, #23153, #17258, #3971, #17554, #49147, #8697, #26688, #19600, #27856, #42340, #51205, #6310, #28443 ),
 .UNSPECIFIED., .F., .F.,
 ( 4, 2, 2, 2, 2, 2, 2, 2, 4 ),
 ( 0.000000000000000000, 0.1250000000000000000, 0.2500000000000000000, 0.3750000000000000000, 0.5000000000000000000, 0.6250000000000000000, 0.7500000000000000000, 0.8750000000000000000, 1.000000000000000000 ),
 .UNSPECIFIED. ) ;
#5940=CARTESIAN_POINT ( 'NONE',  ( 8.196408543750321130, -76.36575423402705098, 9.036094815919039291 ) ) ;
#5941=CARTESIAN_POINT ( 'NONE',  ( 7.103502425096676731, -78.87345073205365509, 9.415326140932604559 ) ) ;
#5943=CARTESIAN_POINT ( 'NONE',  ( 8.645668071321999548, -78.57107317891799880, 7.146365085715999044 ) ) ;
#5963=CARTESIAN_POINT ( 'NONE',  ( 12.00000000000000000, -79.65000000000000568, 0.000000000000000000 ) ) ;
#5965=CARTESIAN_POINT ( 'NONE',  ( 9.769349281881931191, -77.88441593596398604, 4.488065258493001863 ) ) ;
#5966=CARTESIAN_POINT ( 'NONE',  ( 7.919842512016999514, -77.45141689038899813, 8.988445846368000147 ) ) ;
#5967=DIRECTION ( 'NONE',  ( -1.000000000000000000, 0.000000000000000000, 0.000000000000000000 ) ) ;
#5970=CARTESIAN_POINT ( 'NONE',  ( 9.648882615658788353, -80.88645074276622893, 4.741768800263339578 ) ) ;
#5973=CARTESIAN_POINT ( 'NONE',  ( 10.12138908678999982, -77.74142057354099222, 4.388532480841000449 ) ) ;
#5975=CARTESIAN_POINT ( 'NONE',  ( -12.00000000000000178, -78.31041666666665435, -1.570796326794897890 ) ) ;
#5979=CARTESIAN_POINT ( 'NONE',  ( 8.098288960089517374, -80.40744867782952099, 7.103106135035865520 ) ) ;
#5980=CARTESIAN_POINT ( 'NONE',  ( -6.984027423104000043, -77.19459030567298896, 8.777327129872999123 ) ) ;
#5991=CARTESIAN_POINT ( 'NONE',  ( 7.538328940028000247, -76.95994809191398645, -8.367052130149000178 ) ) ;
#6004=CARTESIAN_POINT ( 'NONE',  ( -10.85854583389000005, -79.44473956280799598, 1.947746583844000012 ) ) ;
#6028=CARTESIAN_POINT ( 'NONE',  ( 9.596002108778145967, -76.70208333333333428, 7.374560639699002884 ) ) ;
#6036=CARTESIAN_POINT ( 'NONE',  ( -10.74950085534044852, -76.61052573971902291, -1.407179153412859929 ) ) ;
#6040=CARTESIAN_POINT ( 'NONE',  ( -1.570796326794937636, -78.28541666666666288, 11.99999999999999467 ) ) ;
#6049=DIRECTION ( 'NONE',  ( 1.000000000000000000, 0.000000000000000000, 0.000000000000000000 ) ) ;
#6053=CARTESIAN_POINT ( 'NONE',  ( -0.007641576831010176221, -79.47517447817466518, 10.74992670947085571 ) ) ;
#6055=FACE_OUTER_BOUND ( 'NONE', #12407, .T. ) ;
#6068=CARTESIAN_POINT ( 'NONE',  ( -9.390656772802731922, -77.14192976238929589, -5.419584780083640752 ) ) ;
#6073=CARTESIAN_POINT ( 'NONE',  ( -2.112861425255000203, -79.31263287794399730, -11.84242215301999934 ) ) ;
#6078=CARTESIAN_POINT ( 'NONE',  ( 7.455335830631999450, -78.44471668781000062, 9.319520915745998835 ) ) ;
#6081=CARTESIAN_POINT ( 'NONE',  ( 10.74999999999999645, -78.76041666666667140, 1.407171709420451666 ) ) ;
#6082=ORIENTED_EDGE ( 'NONE', *, *, #54858, .T. ) ;
#6084=CARTESIAN_POINT ( 'NONE',  ( 12.00000000000000000, -79.65000000000000568, 0.000000000000000000 ) ) ;
#6091=CARTESIAN_POINT ( 'NONE',  ( -10.99392646372974092, -79.79999999999999716, -4.674613442768594140 ) ) ;
#6095=CARTESIAN_POINT ( 'NONE',  ( -1.660522255173999984, -76.58517650455699766, 11.05968181062000077 ) ) ;
#6096=CARTESIAN_POINT ( 'NONE',  ( -0.8307515566936579665, -76.48212377155830666, 10.82435606304636799 ) ) ;
#6109=CARTESIAN_POINT ( 'NONE',  ( -10.05357165398491759, -78.07129154303414964, 3.808089728372485272 ) ) ;
#6123=CARTESIAN_POINT ( 'NONE',  ( -8.771511755855000203, -77.43509585594499356, -8.593972346821999508 ) ) ;
#6129=CARTESIAN_POINT ( 'NONE',  ( 11.39554093367000043, -81.02324881952658586, -0.4788264379577999996 ) ) ;
#6143=ORIENTED_EDGE ( 'NONE', *, *, #25630, .F. ) ;
#6149=CARTESIAN_POINT ( 'NONE',  ( -4.817132589604000259, -78.85146397087400771, -11.17039677886999982 ) ) ;
#6157=CARTESIAN_POINT ( 'NONE',  ( 3.140974612311327796, -79.65416666666664014, 11.68767212001979594 ) ) ;
#6162=ORIENTED_EDGE ( 'NONE', *, *, #36908, .F. ) ;
#6167=CARTESIAN_POINT ( 'NONE',  ( 2.853743189566999534E-14, -82.00000000000000000, -10.34999999999597797 ) ) ;
#6171=DIRECTION ( 'NONE',  ( 0.000000000000000000, -1.000000000000000000, 0.000000000000000000 ) ) ;
#6177=CARTESIAN_POINT ( 'NONE',  ( 5.459501886381000091, -76.22776474484699349, -11.00074850082999767 ) ) ;
#6181=CARTESIAN_POINT ( 'NONE',  ( -7.408849624938999234, -79.31758544377551345, -8.421820339245000397 ) ) ;
#6189=CARTESIAN_POINT ( 'NONE',  ( 11.60231809276000092, -78.73711054799299802, -3.252995651540999678 ) ) ;
#6205=CARTESIAN_POINT ( 'NONE',  ( 4.671862542492999815, -78.93563051119899399, -10.24732477002999964 ) ) ;
#6206=CARTESIAN_POINT ( 'NONE',  ( 2.076511064785050653, -76.21002604798447067, 10.98936983701634418 ) ) ;
#6207=CARTESIAN_POINT ( 'NONE',  ( 2.885036932590493652, -79.69456034571689429, -11.47827798692048873 ) ) ;
#6217=B_SPLINE_SURFACE_WITH_KNOTS ( 'NONE', 3, 3, ( 
 ( #43224, #44087, #35196, #3072, #57372, #16931, #7782, #30492, #11646, #8065, #38781, #30772, #53228, #34912, #52944, #44367, #12494, #52375, #48521, #56799, #34629, #3919, #26060, #21922, #3353, #7493, #29905, #47677, #3637, #16358, #34339, #21350, #30197, #56511, #11928, #25490, #47960, #52655, #39645, #43511, #39071, #16644, #39365, #12210, #29623, #48245, #57652, #17208, #45854, #49692, #49396, #35790, #31943, #9239, #27224, #22218, #8647, #13654, #44963, #8945, #40529, #49987, #31649, #44667, #14235, #4811, #13060 ),
 ( #27516, #4518, #17501, #414, #40822, #50275, #17804, #35490, #9823, #40229, #9532, #22520, #36383, #27807, #39931, #45557, #57947, #18100, #123, #58242, #53519, #53821, #31059, #54409, #36096, #5103, #23102, #41112, #13357, #26932, #54113, #49096, #18392, #45264, #26632, #703, #31355, #22811, #10707, #11285, #10997, #28098, #28981, #51445, #6256, #51736, #41989, #38130, #46147, #32520, #41406, #47022, #23682, #2141, #29264, #15702, #28684, #19265, #5966, #5672, #20143, #6552, #50564, #24561, #55862, #37256, #42578 ),
 ( #33407, #10118, #56153, #33696, #1854, #19849, #47312, #37843, #55268, #15414, #41695, #1557, #23394, #24270, #989, #46736, #32813, #14816, #14527, #42287, #50860, #10405, #33109, #55563, #18974, #28390, #46437, #23970, #19548, #36965, #37546, #15112, #51152, #54979, #11574, #35130, #3002, #12141, #34271, #12711, #16574, #16292, #2716, #39290, #34559, #52591, #29554, #33983, #39003, #11862, #52306, #7422, #16864, #57012, #47609, #21574, #30129, #38422, #7710, #53162, #7133, #52876, #29839, #42867, #25712, #48178, #7997 ),
 ( #47891, #56733, #43738, #25134, #30704, #20998, #3290, #25426, #6841, #21283, #43441, #20713, #57302, #34845, #12429, #43159, #52020, #30422, #48455, #25994, #44018, #3570, #39579, #38713, #57582, #17144, #56441, #24852, #2425, #20428, #15996, #13288, #26286, #9170, #49623, #23031, #18324, #54340, #53751, #8871, #41046, #635, #44893, #18617, #36019, #22445, #13879, #17433, #53448, #44300, #31281, #36606, #9463, #48740, #27152, #44594, #57876, #58169, #54629, #49323, #26563, #26865, #14166, #5029, #31874, #8284, #40751 ) ),
 .UNSPECIFIED., .F., .F., .F.,
 ( 4, 4 ),
 ( 4, 1, 1, 1, 1, 1, 1, 1, 1, 1, 1, 1, 1, 1, 1, 1, 1, 1, 1, 1, 1, 1, 1, 1, 1, 1, 1, 1, 1, 1, 1, 1, 1, 1, 1, 1, 1, 1, 1, 1, 1, 1, 1, 1, 1, 1, 1, 1, 1, 1, 1, 1, 1, 1, 1, 1, 1, 1, 1, 1, 1, 1, 1, 1, 4 ),
 ( -0.5168282991433000850, 1.516828299142999992 ),
 ( -0.02000000000000000042, -0.003749999999999999861, 0.01250000000000000069, 0.02875000000000000125, 0.04499999999999999833, 0.06124999999999999889, 0.07749999999999999944, 0.09375000000000000000, 0.1100000000000000006, 0.1262500000000000011, 0.1424999999999999878, 0.1587500000000000022, 0.1749999999999999889, 0.1912500000000000033, 0.2074999999999999900, 0.2237500000000000044, 0.2399999999999999911, 0.2562499999999999778, 0.2725000000000000200, 0.2887500000000000067, 0.3049999999999999933, 0.3212499999999999800, 0.3375000000000000222, 0.3537500000000000089, 0.3699999999999999956, 0.3862499999999999822, 0.4025000000000000244, 0.4187500000000000111, 0.4349999999999999978, 0.4512499999999999845, 0.4675000000000000266, 0.4837500000000000133, 0.5000000000000000000, 0.5162499999999999867, 0.5324999999999999734, 0.5487499999999999600, 0.5649999999999999467, 0.5812500000000000444, 0.5975000000000000311, 0.6137500000000000178, 0.6300000000000000044, 0.6462499999999999911, 0.6624999999999999778, 0.6787499999999999645, 0.6949999999999999512, 0.7112500000000000488, 0.7275000000000000355, 0.7437500000000000222, 0.7600000000000000089, 0.7762499999999999956, 0.7924999999999999822, 0.8087499999999999689, 0.8249999999999999556, 0.8412500000000000533, 0.8575000000000000400, 0.8737500000000000266, 0.8900000000000000133, 0.9062500000000000000, 0.9224999999999999867, 0.9387499999999999734, 0.9549999999999999600, 0.9712499999999999467, 0.9875000000000000444, 1.003749999999999920, 1.020000000000000018 ),
 .UNSPECIFIED. ) ;
#6224=CARTESIAN_POINT ( 'NONE',  ( 8.943349029703989927, -78.80334685903174829, -5.964646307384620094 ) ) ;
#6231=CARTESIAN_POINT ( 'NONE',  ( 5.137083998358000336, -77.21100733245999947, -10.56753840748999984 ) ) ;
#6232=CARTESIAN_POINT ( 'NONE',  ( 9.450616389032896691, -77.74723657863938797, -7.362461627428266375 ) ) ;
#6233=CARTESIAN_POINT ( 'NONE',  ( -8.286771986066998608, -78.77504344720300367, 7.559597915363999832 ) ) ;
#6241=CARTESIAN_POINT ( 'NONE',  ( 0.000000000000000000, -75.15999999999999659, 0.000000000000000000 ) ) ;
#6242=CARTESIAN_POINT ( 'NONE',  ( 11.68767212001979239, -78.62916666666666288, -3.140974612311342451 ) ) ;
#6254=CARTESIAN_POINT ( 'NONE',  ( 10.69076134079912777, -77.86011180829753187, 1.345938505392821005 ) ) ;
#6255=ADVANCED_FACE ( 'NONE', ( #23669 ), #29402, .F. ) ;
#6256=CARTESIAN_POINT ( 'NONE',  ( 9.450487096927000508, -77.83122730632099717, -7.362360902974999455 ) ) ;
#6263=CARTESIAN_POINT ( 'NONE',  ( -7.675142533464999417, -78.39509280558399951, 7.924261572595001191 ) ) ;
#6265=CARTESIAN_POINT ( 'NONE',  ( 5.403345834808000347, -80.29310691901919483, 9.610968446100999429 ) ) ;
#6269=CARTESIAN_POINT ( 'NONE',  ( 10.46898001190309735, -80.37101647696528062, 2.813233871471190195 ) ) ;
#6270=CARTESIAN_POINT ( 'NONE',  ( 6.433795189870999742, -77.43971739268899057, -9.188274595716000803 ) ) ;
#6274=CARTESIAN_POINT ( 'NONE',  ( -12.12824626824999896, -76.58162878623900838, -0.7688881989071000289 ) ) ;
#6277=AXIS2_PLACEMENT_3D ( 'NONE', #19494, #29776, #47832 ) ;
#6279=EDGE_CURVE ( 'NONE', #46546, #9748, #45044, .T. ) ;
#6285=CARTESIAN_POINT ( 'NONE',  ( -10.91036644271999911, -76.79653003390299659, -2.792455208340000272 ) ) ;
#6288=CARTESIAN_POINT ( 'NONE',  ( -7.374560639699022424, -77.72708333333333997, 9.596002108778135309 ) ) ;
#6291=DIRECTION ( 'NONE',  ( 0.000000000000000000, -1.000000000000000000, 1.360822088842000019E-13 ) ) ;
#6299=CARTESIAN_POINT ( 'NONE',  ( 10.32003611956000100, -80.18012082385709505, -3.898536120860000231 ) ) ;
#6310=CARTESIAN_POINT ( 'NONE',  ( 12.00000000000000888, -76.53958333333119413, -1.570796326794872577 ) ) ;
#6315=CARTESIAN_POINT ( 'NONE',  ( 0.000000000000000000, -80.79999999999999716, 0.000000000000000000 ) ) ;
#6347=CARTESIAN_POINT ( 'NONE',  ( -0.4536591235910606423, -79.47852630003501417, 10.74087249166092306 ) ) ;
#6356=CARTESIAN_POINT ( 'NONE',  ( 0.000000000000000000, -82.09999999999999432, 0.000000000000000000 ) ) ;
#6359=CARTESIAN_POINT ( 'NONE',  ( 4.692082659980980175, -80.26118559034645727, -9.672370880052689301 ) ) ;
#6361=CARTESIAN_POINT ( 'NONE',  ( -6.926502605637190335, -77.16933908148428145, -8.221045740255387813 ) ) ;
#6365=EDGE_CURVE ( 'NONE', #15288, #47432, #40856, .T. ) ;
#6366=CARTESIAN_POINT ( 'NONE',  ( -3.970056213021999625, -79.03565890873500166, 11.35542513096999961 ) ) ;
#6371=CARTESIAN_POINT ( 'NONE',  ( 10.38571723084000098, -77.33241475543599108, -5.879822389739000066 ) ) ;
#6376=EDGE_LOOP ( 'NONE', ( #18160, #56694, #21293, #30665 ) ) ;
#6386=CARTESIAN_POINT ( 'NONE',  ( 10.90226209911854127, -79.80000000000003979, 4.526743382750034961 ) ) ;
#6390=CARTESIAN_POINT ( 'NONE',  ( 7.778176538613999824, -76.45230952192000018, -8.035785801754000701 ) ) ;
#6393=CARTESIAN_POINT ( 'NONE',  ( -5.027353609631000531, -76.73535067984099101, 10.04038870902000014 ) ) ;
#6400=CARTESIAN_POINT ( 'NONE',  ( -8.246369313880999030, -79.51135969142900706, 8.832712023146999769 ) ) ;
#6401=CARTESIAN_POINT ( 'NONE',  ( -8.746972750979978173, -78.05079177105272947, 6.251516341120114006 ) ) ;
#6421=CARTESIAN_POINT ( 'NONE',  ( -1.632746748298000039, -81.09541249912808780, 11.17026117058999901 ) ) ;
#6424=CARTESIAN_POINT ( 'NONE',  ( -10.54491486739000017, -77.92936695826499260, -3.823987582478999947 ) ) ;
#6430=ORIENTED_EDGE ( 'NONE', *, *, #7238, .F. ) ;
#6440=CARTESIAN_POINT ( 'NONE',  ( 1.659836960048000076, -79.12275712511198833, 11.81542141165000004 ) ) ;
#6445=B_SPLINE_CURVE_WITH_KNOTS ( 'NONE', 3,
 ( #14651, #37383, #14944, #50985, #28519, #42121, #28811, #1687, #46859, #34972, #15832, #16125, #11989, #30551, #42996, #12553, #57140, #7551, #43569, #21123, #16705, #34103, #52716, #48017, #25550, #2553, #47443, #12269, #29678, #20554, #30258, #24974, #48583, #11704, #26129, #3133, #51858, #39128, #8128, #34687, #44150, #47728, #38550, #56565, #56282, #53002, #11413, #16415, #39424, #43282, #16991, #52144, #57430, #7263, #29967, #29393, #33819, #20267, #38259, #6971, #25264, #2837, #7837, #20833, #38840, #48298, #3414, #25839, #56857, #43866, #21414, #12869, #3733, #35294, #3447, #21453, #39741, #39460, #20874, #57464, #52184, #53042, #38877, #20594, #21734, #11740, #57751, #53324, #48619, #3170, #56606, #30004, #34144, #30872, #43034, #17308, #7874, #26168, #17025, #48907, #38591, #16454, #52752, #29717, #25013, #21160, #30296, #52465, #2596, #34722, #34436, #56897, #35009, #12306, #48335, #47765, #7300, #12589, #12024, #25302, #30588, #8166, #16166 ),
 .UNSPECIFIED., .F., .F.,
 ( 4, 2, 1, 2, 2, 1, 2, 2, 2, 2, 1, 2, 2, 1, 1, 1, 2, 2, 2, 2, 2, 2, 2, 2, 2, 2, 2, 2, 1, 1, 1, 2, 2, 2, 2, 1, 1, 1, 1, 2, 2, 2, 2, 2, 2, 2, 2, 2, 2, 1, 1, 2, 2, 2, 2, 2, 2, 1, 1, 2, 2, 2, 1, 2, 2, 1, 1, 1, 2, 2, 2, 4 ),
 ( 0.000000000000000000, 0.06250000000001762479, 0.07031250000001984524, 0.07128906250002013667, 0.07226562500002041423, 0.07421875000002099709, 0.07812500000002214895, 0.09375000000002668699, 0.1250000000000358602, 0.1406250000000404121, 0.1425781250000410227, 0.1428222656250410227, 0.1430664062500410505, 0.1435546875000410227, 0.1445312500000409672, 0.1484375000000408562, 0.1562500000000406342, 0.1875000000000399125, 0.2500000000000383582, 0.2812500000000378031, 0.2851562500000378031, 0.2890625000000377476, 0.2968750000000377476, 0.3125000000000378031, 0.3750000000000384137, 0.3906250000000385803, 0.3925781250000386358, 0.3930664062500386913, 0.3935546875000386913, 0.3945312500000385803, 0.3984375000000378031, 0.4062500000000363043, 0.4375000000000301426, 0.4687500000000240363, 0.4843750000000209832, 0.4921875000000193734, 0.4960937500000185407, 0.4980468750000181521, 0.4990234375000179301, 0.4995117187500178746, 0.5000000000000177636, 0.5625000000000000000, 0.5703124999999977796, 0.5781249999999954481, 0.5937499999999908962, 0.6249999999999816813, 0.6406249999999771294, 0.6425781249999765743, 0.6435546874999763522, 0.6445312499999760192, 0.6484374999999749090, 0.6562499999999727995, 0.6874999999999640288, 0.7499999999999467093, 0.7812499999999379385, 0.7851562499999369393, 0.7871093749999364952, 0.7890624999999360512, 0.7968749999999341638, 0.8124999999999303890, 0.8749999999999151790, 0.8906249999999114042, 0.8925781249999109601, 0.8928222656249110711, 0.8930664062499110711, 0.8935546874999115152, 0.8945312499999122924, 0.8984374999999158451, 0.9062499999999222844, 0.9374999999999481526, 0.9687499999999741318, 1.000000000000000000 ),
 .UNSPECIFIED. ) ;
#6451=CARTESIAN_POINT ( 'NONE',  ( 10.91653581620999880, -78.32390417293299834, 0.06787400445098999702 ) ) ;
#6469=CARTESIAN_POINT ( 'NONE',  ( -6.018890980713000438, -76.04965686829399374, 10.70471907396000155 ) ) ;
#6470=PLANE ( 'NONE',  #31757 ) ;
#6473=CARTESIAN_POINT ( 'NONE',  ( 7.808618912244999599, -78.93627664175009784, -8.052551227705000869 ) ) ;
#6481=CARTESIAN_POINT ( 'NONE',  ( 4.400069678882000623, -77.16361025341399227, -11.21761009915999985 ) ) ;
#6486=CARTESIAN_POINT ( 'NONE',  ( -6.155296265070999695, -79.10392148219399644, -9.015968826447998907 ) ) ;
#6490=CARTESIAN_POINT ( 'NONE',  ( -10.75000000000000000, -77.50000000000000000, 0.000000000000000000 ) ) ;
#6499=CARTESIAN_POINT ( 'NONE',  ( -9.774834661796999669, -79.23523028421899994, 5.593440076811999617 ) ) ;
#6502=CARTESIAN_POINT ( 'NONE',  ( 0.000000000000000000, -90.29999999999999716, -9.699999999999990408 ) ) ;
#6511=DIRECTION ( 'NONE',  ( 0.000000000000000000, 0.7071067811866525998, -0.7071067811864425456 ) ) ;
#6512=CARTESIAN_POINT ( 'NONE',  ( -1.407249236881253918, -78.48544456714265038, 10.74983227778450257 ) ) ;
#6516=EDGE_LOOP ( 'NONE', ( #2728, #28800, #9166, #4919 ) ) ;
#6518=CARTESIAN_POINT ( 'NONE',  ( 5.788238289111504287, -78.77040165266161864, -9.060210061007026638 ) ) ;
#6523=CARTESIAN_POINT ( 'NONE',  ( -12.00000000000000000, -77.89999999999999147, -2.795183092923000262E-14 ) ) ;
#6527=CARTESIAN_POINT ( 'NONE',  ( 10.58946819037999987, -78.55715270318900423, -3.698823201301000285 ) ) ;
#6534=CARTESIAN_POINT ( 'NONE',  ( -7.712802233773871308, -77.41457454146333816, -8.144586586592856392 ) ) ;
#6549=CARTESIAN_POINT ( 'NONE',  ( 11.68767212001979239, -79.62916666666666288, -3.140974612311342451 ) ) ;
#6551=CARTESIAN_POINT ( 'NONE',  ( 9.662219778377666657, -79.31367287321590709, -4.763839899825916824 ) ) ;
#6552=CARTESIAN_POINT ( 'NONE',  ( 11.79843486695000010, -77.37002894411699572, -2.076781258317999868 ) ) ;
#6560=CARTESIAN_POINT ( 'NONE',  ( 7.384237969039999072, -77.14222102750099452, -8.196021229627000082 ) ) ;
#6562=CARTESIAN_POINT ( 'NONE',  ( -11.68767212001979061, -78.32083333333333997, -3.140974612311365988 ) ) ;
#6564=ORIENTED_EDGE ( 'NONE', *, *, #46709, .F. ) ;
#6567=CARTESIAN_POINT ( 'NONE',  ( 0.7038322923064118664, -80.46990387931118960, 10.74953000798084624 ) ) ;
#6568=CARTESIAN_POINT ( 'NONE',  ( -11.14038684213999986, -78.32459623601998544, 1.307628137226999998 ) ) ;
#6572=CARTESIAN_POINT ( 'NONE',  ( 3.274231746039999891, -77.15535827300999472, -11.82472670181999952 ) ) ;
#6604=CARTESIAN_POINT ( 'NONE',  ( 1.099819419251000019, -79.56550200271298934, 11.16281809564999961 ) ) ;
#6609=FACE_BOUND ( 'NONE', #20185, .T. ) ;
#6615=CARTESIAN_POINT ( 'NONE',  ( -2.813789756862251856, -76.60416666666665719, -10.47020627418439709 ) ) ;
#6623=CARTESIAN_POINT ( 'NONE',  ( 10.40619348602752048, -76.82933193274368477, -2.787222590573924297 ) ) ;
#6629=DIRECTION ( 'NONE',  ( 0.000000000000000000, 1.000000000000000000, 0.000000000000000000 ) ) ;
#6630=CARTESIAN_POINT ( 'NONE',  ( -10.48543666025111776, -78.35833333333332007, 6.043427764450754580 ) ) ;
#6633=DIRECTION ( 'NONE',  ( 1.000000000000000000, 0.000000000000000000, 0.000000000000000000 ) ) ;
#6636=ORIENTED_EDGE ( 'NONE', *, *, #8883, .F. ) ;
#6643=CARTESIAN_POINT ( 'NONE',  ( -2.308100210809882036, -79.49222366784911742, 10.49994118944253785 ) ) ;
#6654=CARTESIAN_POINT ( 'NONE',  ( 10.74987231437827084, -80.34986571895258578, -0.04688819721409577534 ) ) ;
#6657=EDGE_LOOP ( 'NONE', ( #42369, #16118, #3633, #58366, #31617 ) ) ;
#6659=CARTESIAN_POINT ( 'NONE',  ( 11.92746894621999942, -79.46205103218200350, 1.562891678063999867 ) ) ;
#6664=CARTESIAN_POINT ( 'NONE',  ( 0.3849455888886000321, -77.25102680916499764, -11.69935108946000035 ) ) ;
#6678=ORIENTED_EDGE ( 'NONE', *, *, #15474, .T. ) ;
#6681=CARTESIAN_POINT ( 'NONE',  ( 0.8532591808235191477, -79.79999999999998295, -11.75147895264783493 ) ) ;
#6686=CARTESIAN_POINT ( 'NONE',  ( -10.07624512687999996, -76.36960642326199888, -4.852130239470000106 ) ) ;
#6687=CARTESIAN_POINT ( 'NONE',  ( 8.696932689530999738, -76.29999999999999716, -6.318691462144000681 ) ) ;
#6689=CARTESIAN_POINT ( 'NONE',  ( -5.192466827641999849, -76.54473956280799030, -9.696398534197001595 ) ) ;
#6692=AXIS2_PLACEMENT_3D ( 'NONE', #33216, #51261, #28199 ) ;
#6697=CARTESIAN_POINT ( 'NONE',  ( 11.09871289063999988, -79.85894599990470510, 4.778917828262999379 ) ) ;
#6698=CARTESIAN_POINT ( 'NONE',  ( -10.60148741414840856, -78.08680037169739308, 1.782181226894791193 ) ) ;
#6720=CARTESIAN_POINT ( 'NONE',  ( -2.309466437479000156, -77.79318524325600492, 10.97654204954999990 ) ) ;
#6736=CARTESIAN_POINT ( 'NONE',  ( -9.022824479474000015, -78.20036040070399963, 8.159115699504999597 ) ) ;
#6740=CARTESIAN_POINT ( 'NONE',  ( 11.68767212001977995, -79.57083333333332575, 3.140974612311385972 ) ) ;
#6742=VERTEX_POINT ( 'NONE', #18605 ) ;
#6744=CARTESIAN_POINT ( 'NONE',  ( -10.46946769381999864, -78.59626760295098791, -3.092832390908999862 ) ) ;
#6746=VECTOR ( 'NONE', #43139, 1000.000000000000000 ) ;
#6747=CARTESIAN_POINT ( 'NONE',  ( 6.557594696296815684, -80.77712964829170517, -8.547591727114575377 ) ) ;
#6762=CARTESIAN_POINT ( 'NONE',  ( -1.925872869407999843, -76.67857486620199836, -12.12904120624999926 ) ) ;
#6774=CARTESIAN_POINT ( 'NONE',  ( 8.905881360917000222, -78.75077142985099954, 8.286615985300000986 ) ) ;
#6780=CARTESIAN_POINT ( 'NONE',  ( -10.37577574274595804, -79.57882527228287017, 2.833895236981160082 ) ) ;
#6794=CARTESIAN_POINT ( 'NONE',  ( -1.478754609759999950, -78.39090365116300063, -10.94487265352999827 ) ) ;
#6795=CARTESIAN_POINT ( 'NONE',  ( -9.513123067637545560, -76.80684774649085966, 5.706940836106007886 ) ) ;
#6805=CARTESIAN_POINT ( 'NONE',  ( 10.75000000000000000, -78.35000000000000853, 1.923335087985999915E-14 ) ) ;
#6809=CARTESIAN_POINT ( 'NONE',  ( -12.12838880425000099, -77.24017731979098755, 2.901490023383999972 ) ) ;
#6810=CARTESIAN_POINT ( 'NONE',  ( 5.117680542276197286, -78.76455040800591689, -9.453633761533124513 ) ) ;
#6815=CARTESIAN_POINT ( 'NONE',  ( -1.407207572180206867, -79.71460441629234595, -10.68085486824220887 ) ) ;
#6818=CARTESIAN_POINT ( 'NONE',  ( -4.019809786096000259, -79.23806127823398526, 10.47183077952999852 ) ) ;
#6825=CARTESIAN_POINT ( 'NONE',  ( -11.14054172028253475, -78.34061020352532978, 1.307646316399887265 ) ) ;
#6828=CARTESIAN_POINT ( 'NONE',  ( 6.606377239730313988, -80.82291666666665719, 8.596418555780454440 ) ) ;
#6832=EDGE_CURVE ( 'NONE', #13366, #1523, #32261, .T. ) ;
#6833=CARTESIAN_POINT ( 'NONE',  ( 3.714552462503000640, -79.50001896804056400, 11.44155784251000085 ) ) ;
#6840=CARTESIAN_POINT ( 'NONE',  ( 5.413682326552444302, -79.26680726287403900, -9.392823994831353218 ) ) ;
#6841=CARTESIAN_POINT ( 'NONE',  ( 6.917788961650999546, -78.67230555502499101, -9.780606322222999083 ) ) ;
#6844=CARTESIAN_POINT ( 'NONE',  ( -1.407139030276307157, -78.98557530161406248, 10.75050469601710645 ) ) ;
#6846=CARTESIAN_POINT ( 'NONE',  ( 10.02077320556693785, -80.87969032288694393, 3.898277874299578727 ) ) ;
#6849=CARTESIAN_POINT ( 'NONE',  ( 1.483539930421000186, -77.82312960254598977, 10.93164414240999882 ) ) ;
#6851=CARTESIAN_POINT ( 'NONE',  ( 4.292187240357000277, -81.18416302087679526, -9.881207810293000549 ) ) ;
#6859=CARTESIAN_POINT ( 'NONE',  ( -4.531904799951000484, -77.35800836368299827, -10.26060180864999971 ) ) ;
#6868=DIRECTION ( 'NONE',  ( -0.9805806756909162258, 0.1961161351382035567, 2.366670532390040672E-11 ) ) ;
#6891=CARTESIAN_POINT ( 'NONE',  ( -4.410648470793000264, -77.16531204370200214, -9.986067597275999574 ) ) ;
#6905=CARTESIAN_POINT ( 'NONE',  ( -9.393203674808267678, -76.54166666666665719, -5.413904038987171319 ) ) ;
#6930=CARTESIAN_POINT ( 'NONE',  ( -9.662326572316155548, -77.06369712772568903, 4.763895543093616070 ) ) ;
#6940=CARTESIAN_POINT ( 'NONE',  ( 5.230327773973000305, -77.87272937556599572, -9.843691987646998598 ) ) ;
#6945=CARTESIAN_POINT ( 'NONE',  ( 6.063733907601372763, -80.27314283314856880, -8.876350182253380794 ) ) ;
#6946=CARTESIAN_POINT ( 'NONE',  ( 6.436424241555000592, -79.92391735373439587, 8.610165096135999008 ) ) ;
#6949=CARTESIAN_POINT ( 'NONE',  ( -7.858171174022000827, -78.99775398630599454, 9.108036400545000077 ) ) ;
#6954=ORIENTED_EDGE ( 'NONE', *, *, #36938, .F. ) ;
#6955=ORIENTED_EDGE ( 'NONE', *, *, #19142, .T. ) ;
#6965=CARTESIAN_POINT ( 'NONE',  ( -10.52189733146974326, -76.98116804080198960, 2.543646231316468054 ) ) ;
#6969=CARTESIAN_POINT ( 'NONE',  ( -0.1587686074110454537, -79.80000000000001137, -11.79452369934064571 ) ) ;
#6971=CARTESIAN_POINT ( 'NONE',  ( -5.385664337791607359, -80.01701569195293473, 9.304641679316141278 ) ) ;
#6974=CARTESIAN_POINT ( 'NONE',  ( 9.886069181790999139, -76.61296857046200159, -5.228720670581999741 ) ) ;
#6977=CARTESIAN_POINT ( 'NONE',  ( -10.01344192488999951, -76.42684861441699695, -4.821887891087000888 ) ) ;
#6981=FACE_OUTER_BOUND ( 'NONE', #43714, .T. ) ;
#6984=CARTESIAN_POINT ( 'NONE',  ( 3.462695758895999898, -79.92846326159968839, 11.57713085889000126 ) ) ;
#6985=CARTESIAN_POINT ( 'NONE',  ( 11.91015624972854425, -76.21015625001426486, 0.9351146918447083012 ) ) ;
#6990=CARTESIAN_POINT ( 'NONE',  ( 10.74999999999999645, -80.23958333333330017, -1.407171709420461436 ) ) ;
#6993=EDGE_CURVE ( 'NONE', #15223, #24242, #57790, .T. ) ;
#6998=AXIS2_PLACEMENT_3D ( 'NONE', #15497, #10489, #6049 ) ;
#7004=VECTOR ( 'NONE', #20026, 1000.000000000000000 ) ;
#7023=CARTESIAN_POINT ( 'NONE',  ( 3.985687926398000069, -78.60730013205999001, 11.49333817212000142 ) ) ;
#7036=CARTESIAN_POINT ( 'NONE',  ( 3.572416533754999790, -79.98949669345269342, 10.28603406935999942 ) ) ;
#7046=AXIS2_PLACEMENT_3D ( 'NONE', #2459, #20464, #34017 ) ;
#7065=CARTESIAN_POINT ( 'NONE',  ( 10.53043183326000154, -77.29925683053299679, 5.857113494125000486 ) ) ;
#7070=CARTESIAN_POINT ( 'NONE',  ( -9.984422089936529687, -79.56987114508450532, 3.984396093804686512 ) ) ;
#7084=CARTESIAN_POINT ( 'NONE',  ( 6.485260017975245539, -79.37834149910659676, 9.824335988400527242 ) ) ;
#7100=CARTESIAN_POINT ( 'NONE',  ( -0.6836460803099999595, -76.44726687979999724, -12.57002739626000043 ) ) ;
#7101=CARTESIAN_POINT ( 'NONE',  ( -4.675525118886041831, -78.68936016309882575, -9.679868782351919165 ) ) ;
#7105=CARTESIAN_POINT ( 'NONE',  ( 9.700000000000001066, -87.70000000000000284, 0.000000000000000000 ) ) ;
#7106=ADVANCED_FACE ( 'NONE', ( #54833 ), #32661, .T. ) ;
#7109=LINE ( 'NONE', #16547, #9816 ) ;
#7111=CARTESIAN_POINT ( 'NONE',  ( -4.152600241220000044, -79.42871567924700571, -10.41988588363999924 ) ) ;
#7120=CARTESIAN_POINT ( 'NONE',  ( -0.02522437684909708058, -78.47469668865502967, -11.17070649161864537 ) ) ;
#7122=FACE_OUTER_BOUND ( 'NONE', #49064, .T. ) ;
#7133=CARTESIAN_POINT ( 'NONE',  ( 11.81379047889000056, -77.32936970626499829, 1.987564636421000008 ) ) ;
#7140=CARTESIAN_POINT ( 'NONE',  ( 1.589707373765000042, -78.16322009697699968, -10.80037945888999928 ) ) ;
#7148=CARTESIAN_POINT ( 'NONE',  ( -10.54491486739000017, -77.79378985171199190, -3.823987582478999947 ) ) ;
#7153=CARTESIAN_POINT ( 'NONE',  ( -6.524356864576000170, -76.99668890759399176, 10.25272229717000094 ) ) ;
#7180=CARTESIAN_POINT ( 'NONE',  ( -9.204454400623999888, -78.11858404876599593, -5.869700187727000085 ) ) ;
#7186=EDGE_CURVE ( 'NONE', #33872, #17785, #24652, .T. ) ;
#7213=CARTESIAN_POINT ( 'NONE',  ( 10.75000000000000178, -80.25615977947786917, 0.8321152720824881444 ) ) ;
#7228=CARTESIAN_POINT ( 'NONE',  ( -8.584476293286000370, -76.58844565707200047, 6.698613553322000591 ) ) ;
#7233=LINE ( 'NONE', #25237, #9155 ) ;
#7235=CARTESIAN_POINT ( 'NONE',  ( 7.102684642307564467, -79.91784024040764223, 8.111683265999065640 ) ) ;
#7236=CARTESIAN_POINT ( 'NONE',  ( 2.039279229571573815, -79.98945650679056030, -11.03009289294175410 ) ) ;
#7237=CARTESIAN_POINT ( 'NONE',  ( 3.552363299575000077, -79.64717257337099454, -11.49294985030999960 ) ) ;
#7238=EDGE_CURVE ( 'NONE', #31099, #22708, #3517, .T. ) ;
#7240=CARTESIAN_POINT ( 'NONE',  ( 2.417503760557000447, -80.18084841004029784, 10.77648496335999972 ) ) ;
#7241=ORIENTED_EDGE ( 'NONE', *, *, #4965, .F. ) ;
#7262=CARTESIAN_POINT ( 'NONE',  ( 6.590460453269219698, -79.79999999999999716, 9.896017889727964700 ) ) ;
#7263=CARTESIAN_POINT ( 'NONE',  ( -6.807492820124149802, -80.02998060238465428, 8.319674890179079796 ) ) ;
#7266=CARTESIAN_POINT ( 'NONE',  ( -9.831705185582000794, -76.36214915056999075, 5.330239850318999828 ) ) ;
#7269=CARTESIAN_POINT ( 'NONE',  ( 1.838208114491000078, -76.75291386027500096, 10.96086719000000009 ) ) ;
#7275=CARTESIAN_POINT ( 'NONE',  ( 10.20754100699015865, -76.23359375000963212, 6.252571624904344816 ) ) ;
#7287=ADVANCED_FACE ( 'NONE', ( #52019 ), #43158, .F. ) ;
#7292=CARTESIAN_POINT ( 'NONE',  ( 10.78853149093999875, -80.47676253975309635, -3.242959171380999983 ) ) ;
#7300=CARTESIAN_POINT ( 'NONE',  ( 4.442379490556849220, -79.94120693519379017, 9.789819061409028578 ) ) ;
#7315=DIRECTION ( 'NONE',  ( -1.000000000000000000, 0.000000000000000000, 1.155082973713998813E-13 ) ) ;
#7320=CARTESIAN_POINT ( 'NONE',  ( -2.787277769084570256, -80.70420168586483101, -10.40646178475631878 ) ) ;
#7323=VECTOR ( 'NONE', #26923, 1000.000000000000000 ) ;
#7330=CARTESIAN_POINT ( 'NONE',  ( 9.789819849890999848, -78.85111807705811771, -6.904744247936999813 ) ) ;
#7339=CARTESIAN_POINT ( 'NONE',  ( 10.16964605767000052, -76.20095892987599484, -6.884832982024000181 ) ) ;
#7350=CARTESIAN_POINT ( 'NONE',  ( -4.148749056195000229, -78.34383169849499495, 11.43548913926000132 ) ) ;
#7359=CARTESIAN_POINT ( 'NONE',  ( -2.713839119949000178, -79.36594721108400563, -11.84948027859999975 ) ) ;
#7361=CARTESIAN_POINT ( 'NONE',  ( 12.00000000000000000, -79.65000000000000568, 0.000000000000000000 ) ) ;
#7367=ORIENTED_EDGE ( 'NONE', *, *, #53025, .T. ) ;
#7368=CARTESIAN_POINT ( 'NONE',  ( 9.886237701395979016, -76.56117323583245593, -5.228809800238466643 ) ) ;
#7369=CARTESIAN_POINT ( 'NONE',  ( 1.200560589828618463, -79.41667105627126944, 11.71043212083842455 ) ) ;
#7383=CARTESIAN_POINT ( 'NONE',  ( -3.791916262795000048, -77.22593890759399926, 12.00392988483999979 ) ) ;
#7384=CARTESIAN_POINT ( 'NONE',  ( -4.602027720686207246, -78.68996782829300685, -9.715060958940219038 ) ) ;
#7386=VERTEX_POINT ( 'NONE', #3000 ) ;
#7394=CARTESIAN_POINT ( 'NONE',  ( 1.099819419251000019, -79.70107910926499528, 11.16281809564999961 ) ) ;
#7399=VERTEX_POINT ( 'NONE', #39002 ) ;
#7404=CARTESIAN_POINT ( 'NONE',  ( -0.8254061940140534626, -77.46904722746734251, -11.18661314154779873 ) ) ;
#7408=EDGE_CURVE ( 'NONE', #10164, #42165, #45675, .T. ) ;
#7409=CARTESIAN_POINT ( 'NONE',  ( 9.393203674808260573, -80.79166666666664298, 5.413904038987188194 ) ) ;
#7418=ORIENTED_EDGE ( 'NONE', *, *, #36938, .T. ) ;
#7422=CARTESIAN_POINT ( 'NONE',  ( -11.92766985523999956, -77.57353354507900178, -1.116582401450000095 ) ) ;
#7423=DIRECTION ( 'NONE',  ( 0.000000000000000000, -1.000000000000000000, 0.000000000000000000 ) ) ;
#7430=CARTESIAN_POINT ( 'NONE',  ( 6.160618408503998999, -78.35387449799000592, 9.012333039518999556 ) ) ;
#7434=VERTEX_POINT ( 'NONE', #36018 ) ;
#7438=CARTESIAN_POINT ( 'NONE',  ( 5.120381413209000421, -79.16733796702099824, 11.15193929233999981 ) ) ;
#7445=CARTESIAN_POINT ( 'NONE',  ( -10.48589328409999943, -77.03442164589898766, 6.142604583596000367 ) ) ;
#7449=CARTESIAN_POINT ( 'NONE',  ( -10.85854583389000005, -79.12701249839500406, 1.947746583844000012 ) ) ;
#7451=LINE ( 'NONE', #11025, #30110 ) ;
#7469=EDGE_LOOP ( 'NONE', ( #26825, #36934, #24829, #25157 ) ) ;
#7472=CARTESIAN_POINT ( 'NONE',  ( 6.035973157159999936, -78.24568698277398937, -8.925829823522999362 ) ) ;
#7476=CARTESIAN_POINT ( 'NONE',  ( 5.986115112277999195, -80.02851983374358724, 9.486000076385000312 ) ) ;
#7493=CARTESIAN_POINT ( 'NONE',  ( 10.69384760718000038, -78.41447285264899847, -5.399785902169999652 ) ) ;
#7501=CARTESIAN_POINT ( 'NONE',  ( -10.62993649278000063, -77.79662084572800040, 3.720001978191000092 ) ) ;
#7503=CARTESIAN_POINT ( 'NONE',  ( 9.700000000000001066, -90.29999999999999716, 0.000000000000000000 ) ) ;
#7522=CARTESIAN_POINT ( 'NONE',  ( -3.491544874602000359, -78.30851086359500357, -10.58601217070000189 ) ) ;
#7527=CARTESIAN_POINT ( 'NONE',  ( 7.528911431583733105, -80.28673327718702524, -7.673874507591956551 ) ) ;
#7529=CARTESIAN_POINT ( 'NONE',  ( -11.20698691283975457, -79.85327479178147314, -0.4743978281313153689 ) ) ;
#7530=CARTESIAN_POINT ( 'NONE',  ( -9.625846388754000671, -79.04949995641999294, -7.214584339064000318 ) ) ;
#7532=CARTESIAN_POINT ( 'NONE',  ( -10.43948758838000046, -79.85401229401848866, -4.225051887250999449 ) ) ;
#7533=CARTESIAN_POINT ( 'NONE',  ( 8.596672926062478126, -77.40213772681489957, 6.606658478622017938 ) ) ;
#7550=CARTESIAN_POINT ( 'NONE',  ( 0.9278077006636087365, -79.79999999999996874, 11.94918470935973254 ) ) ;
#7551=CARTESIAN_POINT ( 'NONE',  ( -10.22334447120701739, -80.07501482205131538, 3.323462178327394323 ) ) ;
#7553=DIRECTION ( 'NONE',  ( 0.000000000000000000, -1.000000000000000000, 0.000000000000000000 ) ) ;
#7555=CARTESIAN_POINT ( 'NONE',  ( 8.332845033087998843, -76.02681988274399316, -7.273191856730000460 ) ) ;
#7558=CARTESIAN_POINT ( 'NONE',  ( -11.01492454107000007, -76.40176667242799624, -1.480222743997000157 ) ) ;
#7564=CARTESIAN_POINT ( 'NONE',  ( -2.338276403494333966, -77.99259153130903144, 10.49268290638878831 ) ) ;
#7578=CARTESIAN_POINT ( 'NONE',  ( 12.09999999999999964, -92.79999999999999716, 0.000000000000000000 ) ) ;
#7581=CARTESIAN_POINT ( 'NONE',  ( 3.228614917279000185, -80.89813014380396794, -10.79283437469000084 ) ) ;
#7586=CARTESIAN_POINT ( 'NONE',  ( 0.000000000000000000, -76.10312499993298729, 0.000000000000000000 ) ) ;
#7591=ORIENTED_EDGE ( 'NONE', *, *, #5130, .T. ) ;
#7600=CARTESIAN_POINT ( 'NONE',  ( 6.958153983328000614, -78.86512485273199502, -9.837675768602998971 ) ) ;
#7617=CARTESIAN_POINT ( 'NONE',  ( -10.34301771562546435, -80.31833399541898189, 4.325112870545561705 ) ) ;
#7626=CARTESIAN_POINT ( 'NONE',  ( 12.07535958108000074, -76.73373452783998516, -2.237927141218000404 ) ) ;
#7636=CARTESIAN_POINT ( 'NONE',  ( 7.897520336252998874, -77.19073956883799781, -9.100831677656000096 ) ) ;
#7644=CARTESIAN_POINT ( 'NONE',  ( 10.80460657740000130, -79.40475467006099564, -5.315329678968999438 ) ) ;
#7646=ADVANCED_FACE ( 'NONE', ( #35417 ), #53447, .F. ) ;
#7652=DIRECTION ( 'NONE',  ( 0.000000000000000000, -1.000000000000000000, 0.000000000000000000 ) ) ;
#7661=CYLINDRICAL_SURFACE ( 'NONE', #25666, 12.00000000000000000 ) ;
#7667=CARTESIAN_POINT ( 'NONE',  ( -10.47018971533259446, -78.57921329502835306, 2.813858375529144862 ) ) ;
#7671=CARTESIAN_POINT ( 'NONE',  ( -3.213275664864000181, -77.36312553470499154, -12.04962829498999888 ) ) ;
#7672=CARTESIAN_POINT ( 'NONE',  ( 0.03357693874575778253, -78.72534147169611174, -10.74990560618915936 ) ) ;
#7680=CARTESIAN_POINT ( 'NONE',  ( 6.605974356996339836, -79.77709823288482482, -8.595918735704922042 ) ) ;
#7683=CARTESIAN_POINT ( 'NONE',  ( 2.315902194296999728, -78.54323222745999544, -10.97517055051999968 ) ) ;
#7692=CARTESIAN_POINT ( 'NONE',  ( -10.86673736094340192, -76.86984768142733060, -2.781288557130109584 ) ) ;
#7702=CARTESIAN_POINT ( 'NONE',  ( -0.9103933733443999587, -79.76897164566861420, -11.99492895764000089 ) ) ;
#7707=EDGE_CURVE ( 'NONE', #51047, #29449, #33036, .T. ) ;
#7710=CARTESIAN_POINT ( 'NONE',  ( 7.919842512018000491, -77.38362833711200039, 8.988445846368000147 ) ) ;
#7714=CARTESIAN_POINT ( 'NONE',  ( -4.902828564081697316, -76.30798797490987795, 11.02313175347633667 ) ) ;
#7720=ORIENTED_EDGE ( 'NONE', *, *, #40419, .F. ) ;
#7730=CARTESIAN_POINT ( 'NONE',  ( -6.587271542083999343, -76.92896184318099984, 10.35158977641000000 ) ) ;
#7734=CARTESIAN_POINT ( 'NONE',  ( 8.500810681529999968, -79.90288448085529183, -7.210465973013999275 ) ) ;
#7738=B_SPLINE_CURVE_WITH_KNOTS ( 'NONE', 3,
 ( #40555, #36407, #22242, #4541, #31967, #22833, #8373, #40845, #439, #22545 ),
 .UNSPECIFIED., .F., .F.,
 ( 4, 2, 2, 2, 4 ),
 ( 0.000000000000000000, 0.2500000000000000555, 0.5000000000000001110, 0.7500000000000000000, 1.000000000000000000 ),
 .UNSPECIFIED. ) ;
#7740=CARTESIAN_POINT ( 'NONE',  ( 7.374560639698993114, -76.97708333333332575, -9.596002108778149520 ) ) ;
#7750=ORIENTED_EDGE ( 'NONE', *, *, #30956, .T. ) ;
#7757=CARTESIAN_POINT ( 'NONE',  ( 7.977342298186999692, -77.38320278771699634, 7.452340293345999456 ) ) ;
#7763=CARTESIAN_POINT ( 'NONE',  ( 10.93160348586000019, -78.96630245667299164, 2.513594203403000105 ) ) ;
#7782=CARTESIAN_POINT ( 'NONE',  ( 11.53501176087999980, -78.92992984570099679, -3.234124663588000104 ) ) ;
#7787=( NAMED_UNIT ( * ) PLANE_ANGLE_UNIT ( ) SI_UNIT ( $, .RADIAN. ) );
#7788=CARTESIAN_POINT ( 'NONE',  ( -6.841895596235000099, -78.46354745617999527, -8.800175226803998996 ) ) ;
#7793=CARTESIAN_POINT ( 'NONE',  ( -12.00000000000000000, -76.89999999999999147, 0.000000000000000000 ) ) ;
#7807=CARTESIAN_POINT ( 'NONE',  ( 2.927762776937000044, -77.28751179411899841, -10.63625589685999984 ) ) ;
#7808=B_SPLINE_CURVE_WITH_KNOTS ( 'NONE', 3,
 ( #23739, #23448, #50625, #41753 ),
 .UNSPECIFIED., .F., .F.,
 ( 4, 4 ),
 ( 0.000000000000000000, 1.000000000000000000 ),
 .UNSPECIFIED. ) ;
#7813=CARTESIAN_POINT ( 'NONE',  ( 4.114391408450323695, -80.25633541559250261, -9.931419796240385622 ) ) ;
#7815=CARTESIAN_POINT ( 'NONE',  ( -2.710460912692370439, -79.74432941977380551, 10.88462266706781811 ) ) ;
#7819=CARTESIAN_POINT ( 'NONE',  ( -0.7406579117306999471, -79.37821989574298698, 12.00660533699000077 ) ) ;
#7821=CARTESIAN_POINT ( 'NONE',  ( -9.774834661796999669, -79.28204909097999575, 5.593440076811999617 ) ) ;
#7831=ORIENTED_EDGE ( 'NONE', *, *, #48162, .F. ) ;
#7837=CARTESIAN_POINT ( 'NONE',  ( -4.946691137268142135, -80.01318923639908576, 9.544298021765493800 ) ) ;
#7839=CARTESIAN_POINT ( 'NONE',  ( -11.08400893143999966, -76.34452448127198920, -1.489506537590000068 ) ) ;
#7843=AXIS2_PLACEMENT_3D ( 'NONE', #42634, #20200, #11635 ) ;
#7845=CARTESIAN_POINT ( 'NONE',  ( 5.347250836987999634, -76.22619307850399650, 9.743024754427001000 ) ) ;
#7853=CARTESIAN_POINT ( 'NONE',  ( 1.358370974174965440, -80.96534657823993086, 10.66387759044030403 ) ) ;
#7869=CARTESIAN_POINT ( 'NONE',  ( -8.535194087266999574, -80.21887704144299391, 7.565591427388000056 ) ) ;
#7874=CARTESIAN_POINT ( 'NONE',  ( 1.796156089042924897, -79.96199394507185332, 10.59866495730046410 ) ) ;
#7879=SHAPE_REPRESENTATION ( 'Push Button Case', ( #43526 ), #23620 ) ;
#7885=VERTEX_POINT ( 'NONE', #25346 ) ;
#7886=CARTESIAN_POINT ( 'NONE',  ( -11.93030759001999996, -78.70234896019000814, -1.692197530282999907 ) ) ;
#7888=VERTEX_POINT ( 'NONE', #43361 ) ;
#7889=AXIS2_PLACEMENT_3D ( 'NONE', #30989, #45485, #49028 ) ;
#7902=B_SPLINE_CURVE_WITH_KNOTS ( 'NONE', 3,
 ( #46500, #33466, #19908, #51503, #42047, #55624 ),
 .UNSPECIFIED., .F., .F.,
 ( 4, 2, 4 ),
 ( 0.000000000000000000, 0.5000000000000000000, 1.000000000000000000 ),
 .UNSPECIFIED. ) ;
#7905=CARTESIAN_POINT ( 'NONE',  ( 7.483561698776001414, -78.47130766112512390, 9.354804580292000793 ) ) ;
#7923=CARTESIAN_POINT ( 'NONE',  ( 12.25187917533000004, -78.62878573459099130, 0.8290103756198000662 ) ) ;
#7928=CARTESIAN_POINT ( 'NONE',  ( -4.762553456520412176, -79.51167294223473903, 9.637703495840463930 ) ) ;
#7931=CARTESIAN_POINT ( 'NONE',  ( 4.684330217986999223, -79.78092145310699834, -10.80673261319000034 ) ) ;
#7933=CARTESIAN_POINT ( 'NONE',  ( 7.815903581356871577, -79.71875000000000000, 9.154229383352316063 ) ) ;
#7940=ADVANCED_FACE ( 'NONE', ( #12068 ), #38349, .T. ) ;
#7955=SURFACE_SIDE_STYLE ('',( #53123 ) ) ;
#7957=ORIENTED_EDGE ( 'NONE', *, *, #47949, .F. ) ;
#7959=CARTESIAN_POINT ( 'NONE',  ( 10.42437852075000038, -76.52923235641000588, -7.057286423715000367 ) ) ;
#7969=CARTESIAN_POINT ( 'NONE',  ( -5.751434148371999733, -77.83215719852289283, -9.630115047516998317 ) ) ;
#7972=CARTESIAN_POINT ( 'NONE',  ( 10.54265532893000135, -78.67941394246899733, 3.830212845596999927 ) ) ;
#7980=CARTESIAN_POINT ( 'NONE',  ( 7.189039685305540495, -77.07583944371667428, -9.673072753243905808 ) ) ;
#7991=CARTESIAN_POINT ( 'NONE',  ( -5.413904038987206846, -77.91666666666665719, 9.393203674808249914 ) ) ;
#7997=CARTESIAN_POINT ( 'NONE',  ( 0.3864029911681999829, -77.19372312914599377, -11.74364478040999948 ) ) ;
#8014=CARTESIAN_POINT ( 'NONE',  ( -9.811892674444001372, -75.99338179775399738, -7.560764302057000563 ) ) ;
#8019=CARTESIAN_POINT ( 'NONE',  ( -0.2253802134100999777, -78.26452830333799682, -10.88640714497000062 ) ) ;
#8022=B_SPLINE_CURVE_WITH_KNOTS ( 'NONE', 3,
 ( #8465, #9648, #18509, #9065, #36215, #36792, #36503, #53639, #54528, #14066, #31770, #18800, #27050, #5218, #13180, #58064, #26461, #32063 ),
 .UNSPECIFIED., .F., .F.,
 ( 4, 2, 2, 2, 2, 2, 2, 2, 4 ),
 ( 0.000000000000000000, 0.1249999999999999722, 0.2499999999999999445, 0.3749999999999998890, 0.4999999999999998890, 0.6249999999999998890, 0.7499999999999997780, 0.8749999999999998890, 1.000000000000000000 ),
 .UNSPECIFIED. ) ;
#8027=CARTESIAN_POINT ( 'NONE',  ( -11.33781659400000130, -78.29521678053998812, 4.716958136547999558 ) ) ;
#8040=CARTESIAN_POINT ( 'NONE',  ( -7.134970007453478757, -81.00000000000001421, -8.203445754864530315 ) ) ;
#8041=CARTESIAN_POINT ( 'NONE',  ( 5.122310662682999727, -77.73727524673999767, -9.640399341584998893 ) ) ;
#8046=CARTESIAN_POINT ( 'NONE',  ( -9.735611069857000643, -79.15695685768498890, 5.570995215215999607 ) ) ;
#8063=CARTESIAN_POINT ( 'NONE',  ( 11.54819794350999906, -79.30280790634400034, -3.557883190958000430 ) ) ;
#8065=CARTESIAN_POINT ( 'NONE',  ( 3.249499231398999655, -78.84854189942899438, -11.53069031867000049 ) ) ;
#8072=CARTESIAN_POINT ( 'NONE',  ( 3.113304451009999863, -78.49783470746899638, -10.55022916317000181 ) ) ;
#8073=CARTESIAN_POINT ( 'NONE',  ( 7.228832758458999308, -77.14294861368399836, 8.635852100895000660 ) ) ;
#8076=VERTEX_POINT ( 'NONE', #50419 ) ;
#8079=AXIS2_PLACEMENT_3D ( 'NONE', #55797, #33913, #28912 ) ;
#8095=CARTESIAN_POINT ( 'NONE',  ( 3.988644160859999399, -78.36298354959900792, -10.40888963995999994 ) ) ;
#8101=CARTESIAN_POINT ( 'NONE',  ( 0.02474134673687657798, -80.22542497378589132, -10.74983343428174187 ) ) ;
#8105=CARTESIAN_POINT ( 'NONE',  ( 6.536979956083999177, -79.23682303308700625, -10.09826910480999906 ) ) ;
#8108=CARTESIAN_POINT ( 'NONE',  ( -1.407186781496920336, -77.48544845159872807, 10.68067397006091745 ) ) ;
#8111=ORIENTED_EDGE ( 'NONE', *, *, #27080, .F. ) ;
#8116=CARTESIAN_POINT ( 'NONE',  ( -4.041492642110999789, -79.16823080598898343, -10.14108984350000142 ) ) ;
#8122=ORIENTED_EDGE ( 'NONE', *, *, #28150, .F. ) ;
#8123=EDGE_LOOP ( 'NONE', ( #39523, #1832, #37365, #46970, #42879 ) ) ;
#8128=CARTESIAN_POINT ( 'NONE',  ( -8.588659815671681130, -80.04882308261660739, 6.465083054473538482 ) ) ;
#8135=CARTESIAN_POINT ( 'NONE',  ( -4.873207417809000574, -76.93853187307900043, 9.732535352345999868 ) ) ;
#8144=CARTESIAN_POINT ( 'NONE',  ( -1.059394002417758163, -80.98296073876636569, 10.69789347654190337 ) ) ;
#8166=CARTESIAN_POINT ( 'NONE',  ( 6.092940285862026073, -79.92743084948268972, 8.866677603556114562 ) ) ;
#8168=ORIENTED_EDGE ( 'NONE', *, *, #53762, .T. ) ;
#8174=VERTEX_POINT ( 'NONE', #3078 ) ;
#8193=CARTESIAN_POINT ( 'NONE',  ( -6.577349813594124406, -80.77474465748072419, 9.078716047411401036 ) ) ;
#8194=CARTESIAN_POINT ( 'NONE',  ( 2.697636866285999968, -77.79307477553111028, -11.67213861177999945 ) ) ;
#8195=LINE ( 'NONE', #31188, #26519 ) ;
#8202=CARTESIAN_POINT ( 'NONE',  ( -12.27595451887999900, -75.99604523835098746, 0.3505736730271999391 ) ) ;
#8204=AXIS2_PLACEMENT_3D ( 'NONE', #45857, #18977, #36969 ) ;
#8205=CARTESIAN_POINT ( 'NONE',  ( -1.078908860263670499, -78.21713606389884887, -10.72771984716255567 ) ) ;
#8211=CARTESIAN_POINT ( 'NONE',  ( 7.091067894987999942, -78.54739778831900310, -10.02559399679999963 ) ) ;
#8217=CARTESIAN_POINT ( 'NONE',  ( -4.048145914920218580, -79.50588259898441379, 9.958952688048560375 ) ) ;
#8221=CARTESIAN_POINT ( 'NONE',  ( -2.688164603868000047, -79.29822014667099950, -11.73737721775999887 ) ) ;
#8229=VERTEX_POINT ( 'NONE', #29629 ) ;
#8248=CARTESIAN_POINT ( 'NONE',  ( -8.566065236488999091, -77.18668866757499814, -8.735497583133000177 ) ) ;
#8259=CARTESIAN_POINT ( 'NONE',  ( -10.93308570624999732, -78.26793868655188646, -2.507139558745000052 ) ) ;
#8279=CARTESIAN_POINT ( 'NONE',  ( -10.47020627418440242, -77.97916666666668561, 2.813789756862221214 ) ) ;
#8283=CARTESIAN_POINT ( 'NONE',  ( -10.68110250243102399, -79.11058856173531240, -1.407228983746247941 ) ) ;
#8284=CARTESIAN_POINT ( 'NONE',  ( 1.720939166139000109, -77.13497768101099439, -11.69973432676000158 ) ) ;
#8287=CARTESIAN_POINT ( 'NONE',  ( -8.118170145944999305, -78.64206171986300831, -8.748189294319999476 ) ) ;
#8296=CARTESIAN_POINT ( 'NONE',  ( -12.27099179350999947, -79.32713975210698720, -0.08468213707432999116 ) ) ;
#8300=CARTESIAN_POINT ( 'NONE',  ( 5.151324428776999476, -77.67092400397599761, 9.964033682248000900 ) ) ;
#8303=CARTESIAN_POINT ( 'NONE',  ( 12.02938582184000005, -76.71030382554799587, 2.954811323672000167 ) ) ;
#8305=CARTESIAN_POINT ( 'NONE',  ( 9.678374330664796688, -76.78695867686717236, 4.842468990515385485 ) ) ;
#8306=ORIENTED_EDGE ( 'NONE', *, *, #36214, .T. ) ;
#8307=CARTESIAN_POINT ( 'NONE',  ( -1.769784341028000085, -79.82117545184989638, -11.00556513567000039 ) ) ;
#8316=CARTESIAN_POINT ( 'NONE',  ( 6.187157694146999454, -78.15957020342199257, 10.60730214752000045 ) ) ;
#8322=CARTESIAN_POINT ( 'NONE',  ( 10.65991607774613747, -78.83964975953574594, -1.400468160174369148 ) ) ;
#8326=ORIENTED_EDGE ( 'NONE', *, *, #2481, .T. ) ;
#8328=CARTESIAN_POINT ( 'NONE',  ( -5.762797186001000327, -77.55987522413700219, 9.407013499219999630 ) ) ;
#8332=CARTESIAN_POINT ( 'NONE',  ( 3.371435477143000181, -79.34761125869799514, -10.69820234502000034 ) ) ;
#8341=AXIS2_PLACEMENT_3D ( 'NONE', #12135, #30123, #57005 ) ;
#8349=CARTESIAN_POINT ( 'NONE',  ( 1.476561009027000049, -79.44184242973399535, 11.99329713346000048 ) ) ;
#8358=CARTESIAN_POINT ( 'NONE',  ( -11.21475409559999825, -76.81611249766200444, 1.031226285144000165 ) ) ;
#8361=VERTEX_POINT ( 'NONE', #27231 ) ;
#8365=EDGE_CURVE ( 'NONE', #34885, #23335, #17214, .T. ) ;
#8366=CARTESIAN_POINT ( 'NONE',  ( -3.513443458492000016, -78.29796450147399867, -10.65240647004999985 ) ) ;
#8373=CARTESIAN_POINT ( 'NONE',  ( -7.901937438446521966, -76.05000000000001137, 8.782705132841526208 ) ) ;
#8376=CARTESIAN_POINT ( 'NONE',  ( 9.107239040596999402, -78.07663815498800375, 6.625115969983998987 ) ) ;
#8382=CARTESIAN_POINT ( 'NONE',  ( 1.795800964791006482, -80.23879961656356841, -10.60311702371338960 ) ) ;
#8390=CARTESIAN_POINT ( 'NONE',  ( 2.047466772651000078, -79.96295766602578681, -11.07437783411999987 ) ) ;
#8400=CARTESIAN_POINT ( 'NONE',  ( 4.528616239255999432, -78.73244931796000401, -9.933126443765001312 ) ) ;
#8418=CARTESIAN_POINT ( 'NONE',  ( 10.68461344661000112, -76.26131943937400592, -2.075949589353000224 ) ) ;
#8426=CARTESIAN_POINT ( 'NONE',  ( 11.84266115483542237, -77.53516788874328824, -2.236516232491893241 ) ) ;
#8427=CARTESIAN_POINT ( 'NONE',  ( -0.9320940738602599973, -80.98202026695135203, 10.70948474841207876 ) ) ;
#8428=CARTESIAN_POINT ( 'NONE',  ( -2.895922040489999905, -80.29737158873430758, 10.88681414971999928 ) ) ;
#8440=VERTEX_POINT ( 'NONE', #8072 ) ;
#8451=CARTESIAN_POINT ( 'NONE',  ( 0.02140828840467117605, -77.22524110190225599, -10.74993023099652412 ) ) ;
#8459=CARTESIAN_POINT ( 'NONE',  ( 7.972949129781999211, -77.44073956883799781, -9.187753233325999247 ) ) ;
#8465=CARTESIAN_POINT ( 'NONE',  ( 12.00000000000000000, -78.54999999999999716, 0.000000000000000000 ) ) ;
#8467=VERTEX_POINT ( 'NONE', #18399 ) ;
#8474=CARTESIAN_POINT ( 'NONE',  ( -10.85772169724999969, -76.68550427251300050, 1.763485056683000041 ) ) ;
#8496=CARTESIAN_POINT ( 'NONE',  ( -3.157677208335999630, -77.12823906290799414, -10.45009290908999944 ) ) ;
#8498=CARTESIAN_POINT ( 'NONE',  ( -12.26242965668000018, -77.86916490272500369, 0.6546740380507000134 ) ) ;
#8505=CARTESIAN_POINT ( 'NONE',  ( -1.812920252538464894, -78.78700244415333032, 11.90997463893260466 ) ) ;
#8506=CARTESIAN_POINT ( 'NONE',  ( -6.455508761419999963, -79.33931358023599500, -10.30055883293000107 ) ) ;
#8507=CARTESIAN_POINT ( 'NONE',  ( -8.273492252229999622, -80.01569584820420289, 7.333619062208000194 ) ) ;
#8509=CARTESIAN_POINT ( 'NONE',  ( 11.01642476345000077, -77.09896080093798787, 2.111041454437999842 ) ) ;
#8527=FACE_OUTER_BOUND ( 'NONE', #34502, .T. ) ;
#8536=CARTESIAN_POINT ( 'NONE',  ( -8.953452373791000340, -77.06374045265999939, 8.338029955349002265 ) ) ;
#8546=CARTESIAN_POINT ( 'NONE',  ( -10.05535668103000191, -78.21346600054846476, 4.970705447719998560 ) ) ;
#8550=CARTESIAN_POINT ( 'NONE',  ( 11.15679540746000065, -79.65992229053399853, 1.159321710118000004 ) ) ;
#8551=LINE ( 'NONE', #11835, #41220 ) ;
#8560=EDGE_CURVE ( 'NONE', #52300, #20296, #49210, .T. ) ;
#8562=DIRECTION ( 'NONE',  ( -4.860927510790000040E-11, -1.000000000000000000, -3.762819604792999951E-10 ) ) ;
#8566=CARTESIAN_POINT ( 'NONE',  ( -3.970056213021999625, -79.05176450532758281, 11.35542513096999961 ) ) ;
#8567=CARTESIAN_POINT ( 'NONE',  ( 10.75000000000000000, -77.75000000000000000, 0.000000000000000000 ) ) ;
#8569=CARTESIAN_POINT ( 'NONE',  ( 10.75000000000000000, -77.75000000000000000, 0.000000000000000000 ) ) ;
#8570=TOROIDAL_SURFACE ( 'NONE', #13283, 12.50000000000000000, 1.500000000000000000 ) ;
#8575=CARTESIAN_POINT ( 'NONE',  ( -10.74991650949179345, -79.10538127169735390, -0.7036244177452357640 ) ) ;
#8579=CARTESIAN_POINT ( 'NONE',  ( -1.355082891136000001, -77.69253568003099986, -11.85745557885999979 ) ) ;
#8586=FACE_OUTER_BOUND ( 'NONE', #16509, .T. ) ;
#8593=CARTESIAN_POINT ( 'NONE',  ( 3.305503757990000402, -77.08763120859698859, -11.93766403289999900 ) ) ;
#8597=AXIS2_PLACEMENT_3D ( 'NONE', #14048, #17604, #32042 ) ;
#8598=CARTESIAN_POINT ( 'NONE',  ( 0.9420327262254000189, -78.77294003937198852, -10.99155624668999920 ) ) ;
#8605=B_SPLINE_CURVE_WITH_KNOTS ( 'NONE', 3,
 ( #12534, #33591, #30240, #17249, #20036, #21679, #48564, #43550, #28868, #25821, #38024, #8108, #51629, #29946, #35237, #3395, #43850, #7533, #3115, #57119, #34668, #53269 ),
 .UNSPECIFIED., .F., .F.,
 ( 4, 2, 2, 2, 2, 2, 2, 2, 2, 2, 4 ),
 ( 0.000000000000000000, 0.1250000000000001665, 0.2500000000000003331, 0.3125000000000002776, 0.3750000000000002776, 0.4375000000000002220, 0.5000000000000002220, 0.6250000000000001110, 0.7500000000000001110, 0.8750000000000000000, 1.000000000000000000 ),
 .UNSPECIFIED. ) ;
#8606=CARTESIAN_POINT ( 'NONE',  ( 6.606416481926000728, -77.99679431087899673, -10.35137867379999932 ) ) ;
#8609=CARTESIAN_POINT ( 'NONE',  ( -10.47020627418440242, -79.47916666666667140, 2.813789756862221214 ) ) ;
#8620=CARTESIAN_POINT ( 'NONE',  ( -10.75275020201999965, -78.15907477017699989, -2.465785609032999925 ) ) ;
#8624=CARTESIAN_POINT ( 'NONE',  ( 2.039250879084999912, -79.90565398600709557, -11.02993955029000084 ) ) ;
#8627=EDGE_CURVE ( 'NONE', #8467, #14636, #2294, .T. ) ;
#8638=LINE ( 'NONE', #25777, #25028 ) ;
#8644=CARTESIAN_POINT ( 'NONE',  ( -12.41539209960999912, -79.37769575988599513, -0.6693894873470999096 ) ) ;
#8646=CARTESIAN_POINT ( 'NONE',  ( -7.560044382379633277, -78.03705853110491830, 7.642724606814406130 ) ) ;
#8647=CARTESIAN_POINT ( 'NONE',  ( 0.4844284812283000119, -77.57346407451200321, 11.97002061314999999 ) ) ;
#8654=CARTESIAN_POINT ( 'NONE',  ( 5.284336329618000150, -77.98727524673999767, -9.945338310677000138 ) ) ;
#8672=CARTESIAN_POINT ( 'NONE',  ( -10.58739904582000158, -77.80427472496999997, -3.839393962977000196 ) ) ;
#8679=CARTESIAN_POINT ( 'NONE',  ( 4.117763575831188128, -80.25636342326222916, -9.930021758596684123 ) ) ;
#8685=CARTESIAN_POINT ( 'NONE',  ( 3.485296502184999756, -79.24083078338598796, 10.58807389768000107 ) ) ;
#8689=LINE ( 'NONE', #49739, #2339 ) ;
#8693=VECTOR ( 'NONE', #29369, 1000.000000000000000 ) ;
#8696=CARTESIAN_POINT ( 'NONE',  ( -2.665716224216999830, -79.53555764342200973, 10.70493771085999946 ) ) ;
#8697=CARTESIAN_POINT ( 'NONE',  ( 3.140974612311377090, -76.44583333331208053, -11.68767212001978528 ) ) ;
#8698=ADVANCED_FACE ( 'NONE', ( #52740 ), #57453, .T. ) ;
#8715=CARTESIAN_POINT ( 'NONE',  ( -10.90118402791000030, -76.46949373684098816, -1.464937909874000077 ) ) ;
#8719=FACE_OUTER_BOUND ( 'NONE', #47836, .T. ) ;
#8723=CARTESIAN_POINT ( 'NONE',  ( -2.055177818477693652, -80.99049588671762478, 10.56044713659669654 ) ) ;
#8724=CARTESIAN_POINT ( 'NONE',  ( -11.09105850093000001, -80.31987609346899148, 1.974238845993000258 ) ) ;
#8730=CARTESIAN_POINT ( 'NONE',  ( 0.000000000000000000, -75.15999999999999659, 0.000000000000000000 ) ) ;
#8734=VECTOR ( 'NONE', #27908, 1000.000000000000000 ) ;
#8737=EDGE_LOOP ( 'NONE', ( #1444, #8168 ) ) ;
#8750=CARTESIAN_POINT ( 'NONE',  ( -4.886687280655466203, -77.18749172000538294, -9.575324941435306769 ) ) ;
#8759=CARTESIAN_POINT ( 'NONE',  ( -10.02269271100999859, -77.64430565866300071, 6.688901441487999477 ) ) ;
#8764=CARTESIAN_POINT ( 'NONE',  ( 7.374239324226436132, -76.57642972729847486, -9.595271688162245738 ) ) ;
#8771=CARTESIAN_POINT ( 'NONE',  ( -11.76955644394622880, -79.80000000000001137, -2.210969502171932888 ) ) ;
#8775=AXIS2_PLACEMENT_3D ( 'NONE', #7586, #2873, #42159 ) ;
#8777=CARTESIAN_POINT ( 'NONE',  ( 2.228685126279000173, -78.01010929892113666, 11.77068507109000350 ) ) ;
#8795=CARTESIAN_POINT ( 'NONE',  ( 0.1355484243949000023, -77.40060249292598371, 10.91590548763000079 ) ) ;
#8797=CARTESIAN_POINT ( 'NONE',  ( -12.15819904699000098, -78.38462189577700201, -1.724521706148000044 ) ) ;
#8806=CARTESIAN_POINT ( 'NONE',  ( 8.107625576107000853, -78.93752314293499239, 8.443305427288999354 ) ) ;
#8807=CARTESIAN_POINT ( 'NONE',  ( 10.49124522239000079, -80.36320440064619675, -3.841552970220999619 ) ) ;
#8810=CARTESIAN_POINT ( 'NONE',  ( 2.976864594307000011, -77.48026960296300558, -10.81463766284999828 ) ) ;
#8828=CARTESIAN_POINT ( 'NONE',  ( 0.000000000000000000, -75.15999999999999659, 0.000000000000000000 ) ) ;
#8838=CARTESIAN_POINT ( 'NONE',  ( -4.866794825236000044, -76.53096485469599486, 11.22503275805000023 ) ) ;
#8846=CARTESIAN_POINT ( 'NONE',  ( 7.508079800428999917, -76.93335787946290338, -8.333477563431999968 ) ) ;
#8850=CARTESIAN_POINT ( 'NONE',  ( 9.376438147752001129, -79.60544960453100316, -6.156339679782000474 ) ) ;
#8864=CARTESIAN_POINT ( 'NONE',  ( 6.606377239730347739, -79.67708333333331439, -8.596418555780422466 ) ) ;
#8865=CARTESIAN_POINT ( 'NONE',  ( 0.000000000000000000, -76.00000000000000000, 0.000000000000000000 ) ) ;
#8871=CARTESIAN_POINT ( 'NONE',  ( 6.035966914210000311, -77.83129677688799575, 10.34809972146999968 ) ) ;
#8873=CARTESIAN_POINT ( 'NONE',  ( 8.737371597357999065, -78.88622555867699759, 8.129823451939000023 ) ) ;
#8878=CARTESIAN_POINT ( 'NONE',  ( 4.654517711782999889, -79.86653908624468556, 9.874757255799998745 ) ) ;
#8883=EDGE_CURVE ( 'NONE', #7888, #28871, #11772, .T. ) ;
#8888=CARTESIAN_POINT ( 'NONE',  ( -7.770178157204999714, -76.43843624521699098, 9.495887966417999593 ) ) ;
#8890=CARTESIAN_POINT ( 'NONE',  ( -0.5976101762332876044, -76.87935536903508194, 10.80570671848152031 ) ) ;
#8893=CARTESIAN_POINT ( 'NONE',  ( -1.629741404508999958, -78.59554001676799828, 11.02717296151999982 ) ) ;
#8902=AXIS2_PLACEMENT_3D ( 'NONE', #1799, #19212, #10654 ) ;
#8903=CARTESIAN_POINT ( 'NONE',  ( 12.18149635271999820, -78.56650993477799716, -1.551427017228999894 ) ) ;
#8916=ORIENTED_EDGE ( 'NONE', *, *, #17963, .T. ) ;
#8921=CARTESIAN_POINT ( 'NONE',  ( -7.301194973305000779, -79.12972051468399570, 8.515319286630999684 ) ) ;
#8922=CARTESIAN_POINT ( 'NONE',  ( 7.988132153045272688, -81.00000000000000000, 7.420399617384452640 ) ) ;
#8942=CARTESIAN_POINT ( 'NONE',  ( 8.788067143180999352, -78.75025020734798886, 8.070261318923000360 ) ) ;
#8943=CARTESIAN_POINT ( 'NONE',  ( 10.96037575245999918, -76.49979439517699120, -3.836821987761000141 ) ) ;
#8944=CARTESIAN_POINT ( 'NONE',  ( -7.815187951055542648, -78.03981183751436390, 7.382325091166371145 ) ) ;
#8945=CARTESIAN_POINT ( 'NONE',  ( 10.46934363224000109, -77.49207612824099556, 5.823135730235999397 ) ) ;
#8951=CARTESIAN_POINT ( 'NONE',  ( 3.456234606873382020, -80.94905652473062219, 10.18103548260220315 ) ) ;
#8954=CARTESIAN_POINT ( 'NONE',  ( -4.618124570880000057, -78.30012939816998596, 10.14532039989999923 ) ) ;
#8955=CARTESIAN_POINT ( 'NONE',  ( -7.374560639699022424, -78.22708333333335418, 9.596002108778135309 ) ) ;
#8956=CARTESIAN_POINT ( 'NONE',  ( 11.10501747946000073, -80.56036808024779816, -1.836383218517000149 ) ) ;
#8962=CARTESIAN_POINT ( 'NONE',  ( -4.531904799951000484, -77.29021981040699529, -10.26060180864999971 ) ) ;
#8973=CARTESIAN_POINT ( 'NONE',  ( -7.800315838420999626, -76.64709394048399815, 7.658422569234000221 ) ) ;
#8980=CARTESIAN_POINT ( 'NONE',  ( -10.45237130512470181, -80.11958314839849038, -2.607326810107436277 ) ) ;
#8987=CARTESIAN_POINT ( 'NONE',  ( 8.769046271958000460, -78.51943148693000296, -7.066663249742999753 ) ) ;
#8998=CARTESIAN_POINT ( 'NONE',  ( 10.32003611956000100, -79.86239375944418839, -3.898536120860000231 ) ) ;
#9015=CIRCLE ( 'NONE', #8079, 11.59999999999999964 ) ;
#9016=CARTESIAN_POINT ( 'NONE',  ( -9.669536374352000863, -76.41932985286300095, 5.242320344620000405 ) ) ;
#9019=CARTESIAN_POINT ( 'NONE',  ( -11.09105850093000001, -80.25208754019278956, 1.974238845993000258 ) ) ;
#9026=CARTESIAN_POINT ( 'NONE',  ( -12.09999999999999964, -92.79999999999999716, 0.000000000000000000 ) ) ;
#9049=CARTESIAN_POINT ( 'NONE',  ( 7.893016554558063724, -77.29077850116276238, -7.298496125915765020 ) ) ;
#9052=ORIENTED_EDGE ( 'NONE', *, *, #53943, .T. ) ;
#9060=CARTESIAN_POINT ( 'NONE',  ( -11.68231536908000123, -77.67143497408700625, 2.952842578158000109 ) ) ;
#9065=CARTESIAN_POINT ( 'NONE',  ( 10.48543666025108401, -78.59166666666666856, 6.043427764450814976 ) ) ;
#9070=CARTESIAN_POINT ( 'NONE',  ( -11.99583751076623450, -79.79999999999998295, -0.3766131536002892410 ) ) ;
#9073=FACE_OUTER_BOUND ( 'NONE', #12657, .T. ) ;
#9075=CARTESIAN_POINT ( 'NONE',  ( 4.458743082292000004, -77.49465230586955045, 11.11915799896999957 ) ) ;
#9082=EDGE_CURVE ( 'NONE', #33152, #15494, #10419, .T. ) ;
#9095=CARTESIAN_POINT ( 'NONE',  ( 8.827997450462000018, -78.32663815498800375, 6.421979991006000255 ) ) ;
#9097=CARTESIAN_POINT ( 'NONE',  ( 2.739292792226000195, -77.58421086662899313, -11.85237552491999935 ) ) ;
#9106=CARTESIAN_POINT ( 'NONE',  ( 10.38178191893000069, -80.29547733623329009, -3.801471066729000370 ) ) ;
#9111=CARTESIAN_POINT ( 'NONE',  ( -0.8253947190445000137, -77.45303325996100341, -11.18645762290999990 ) ) ;
#9114=AXIS2_PLACEMENT_3D ( 'NONE', #13093, #58275, #39965 ) ;
#9136=CARTESIAN_POINT ( 'NONE',  ( -11.87094579582000087, -77.21343299368299995, -3.415941325536000051 ) ) ;
#9137=CARTESIAN_POINT ( 'NONE',  ( -9.691523086186688118, -78.63578696449211236, -4.654780356785987117 ) ) ;
#9141=AXIS2_PLACEMENT_3D ( 'NONE', #15079, #19520, #37513 ) ;
#9145=AXIS2_PLACEMENT_3D ( 'NONE', #22696, #40708, #18280 ) ;
#9146=CARTESIAN_POINT ( 'NONE',  ( -7.803863155890000236, -78.18622965754646259, 8.057160196619001624 ) ) ;
#9151=VERTEX_POINT ( 'NONE', #29283 ) ;
#9155=VECTOR ( 'NONE', #48554, 1000.000000000000114 ) ;
#9164=DIRECTION ( 'NONE',  ( -1.000000000000000000, 0.000000000000000000, 0.000000000000000000 ) ) ;
#9166=ORIENTED_EDGE ( 'NONE', *, *, #57691, .T. ) ;
#9170=CARTESIAN_POINT ( 'NONE',  ( -11.96278216175999987, -77.99407266942999684, 0.6386762756999999624 ) ) ;
#9172=FACE_OUTER_BOUND ( 'NONE', #4217, .T. ) ;
#9176=CARTESIAN_POINT ( 'NONE',  ( -8.741790450690999137, -79.97548445825189845, 6.538842841549999285 ) ) ;
#9181=CARTESIAN_POINT ( 'NONE',  ( -6.606377239730371720, -77.42708333333332860, 8.596418555780411808 ) ) ;
#9183=CARTESIAN_POINT ( 'NONE',  ( 3.336775769941000114, -77.01990414418399666, -12.05060136398000026 ) ) ;
#9185=CARTESIAN_POINT ( 'NONE',  ( -3.057614831332267524, -76.89783470746864680, 10.38130180429175375 ) ) ;
#9188=CARTESIAN_POINT ( 'NONE',  ( -10.43948758838000046, -79.80719348725739337, -4.225051887250999449 ) ) ;
#9198=CARTESIAN_POINT ( 'NONE',  ( 0.000000000000000000, -75.15999999999999659, 0.000000000000000000 ) ) ;
#9209=CARTESIAN_POINT ( 'NONE',  ( -2.271373002040000255, -77.53263888113500002, 10.79548975578000025 ) ) ;
#9215=CARTESIAN_POINT ( 'NONE',  ( -11.06493808903000087, -79.27921809696499622, -1.839906431680000010 ) ) ;
#9216=CARTESIAN_POINT ( 'NONE',  ( 5.643768039804604619, -81.00000000000002842, 9.293348226988427996 ) ) ;
#9235=CARTESIAN_POINT ( 'NONE',  ( 12.31534470299000006, -79.13438534395299939, 1.709481828355000177 ) ) ;
#9236=CARTESIAN_POINT ( 'NONE',  ( 8.726902940210999660, -75.87452899014900254, 6.502829119990000351 ) ) ;
#9237=CARTESIAN_POINT ( 'NONE',  ( -5.166105824225122767, -78.01496696634453087, 9.427318864941536702 ) ) ;
#9239=CARTESIAN_POINT ( 'NONE',  ( -9.964549960864999889, -77.65485202078399141, 6.650098383618000319 ) ) ;
#9241=CARTESIAN_POINT ( 'NONE',  ( -12.00000000000000000, -79.39999999999999147, 0.000000000000000000 ) ) ;
#9242=CARTESIAN_POINT ( 'NONE',  ( -10.74987180213209292, -79.09496495074813538, 0.7036268749256830990 ) ) ;
#9247=CARTESIAN_POINT ( 'NONE',  ( 10.72689817447000138, -77.61922082312399596, -3.031213639016000272 ) ) ;
#9249=CARTESIAN_POINT ( 'NONE',  ( 4.142522846324000696, -80.80321295308820595, 10.21795800799999832 ) ) ;
#9255=CARTESIAN_POINT ( 'NONE',  ( -9.998780405325002008, -77.23574712440399992, -5.083552005986999411 ) ) ;
#9259=CARTESIAN_POINT ( 'NONE',  ( -7.711243899566701643, -78.56159779477874849, -7.536022382359825578 ) ) ;
#9265=CARTESIAN_POINT ( 'NONE',  ( 10.22699339414000086, -77.49142057354099222, 4.434321446068000050 ) ) ;
#9273=CARTESIAN_POINT ( 'NONE',  ( -10.75744095928762789, -78.87276644371578982, -3.177903864377569665 ) ) ;
#9277=CARTESIAN_POINT ( 'NONE',  ( 6.836697942985000331, -79.21359444038398578, 8.804212730688998789 ) ) ;
#9288=EDGE_CURVE ( 'NONE', #6742, #24385, #31500, .T. ) ;
#9305=CARTESIAN_POINT ( 'NONE',  ( 10.77194460988999936, -76.78804022114499617, 1.560654010453999874 ) ) ;
#9309=CARTESIAN_POINT ( 'NONE',  ( -0.3187246912203000049, -80.64335745824000412, 11.26088853021000169 ) ) ;
#9316=CARTESIAN_POINT ( 'NONE',  ( 7.496935112050000072, -80.71873919278517917, 8.408636027568000770 ) ) ;
#9322=ADVANCED_FACE ( 'NONE', ( #37686 ), #14378, .F. ) ;
#9328=CARTESIAN_POINT ( 'NONE',  ( -3.584700322809565520, -79.50216406493034071, 10.13469974220001113 ) ) ;
#9332=ORIENTED_EDGE ( 'NONE', *, *, #5039, .T. ) ;
#9343=ADVANCED_FACE ( 'NONE', ( #30842 ), #828, .F. ) ;
#9345=CARTESIAN_POINT ( 'NONE',  ( -2.166067413260452490, -77.20901008302325863, -10.53065413872945300 ) ) ;
#9349=CARTESIAN_POINT ( 'NONE',  ( -0.9103933733443999587, -79.82065460235210708, -11.99492895764000089 ) ) ;
#9354=CARTESIAN_POINT ( 'NONE',  ( -4.109499447189000065, -78.59383169849499495, 11.32730267836999971 ) ) ;
#9360=ORIENTED_EDGE ( 'NONE', *, *, #20685, .F. ) ;
#9371=CARTESIAN_POINT ( 'NONE',  ( 10.42503750987000011, -77.35900572875097225, -5.902083371034001047 ) ) ;
#9373=CARTESIAN_POINT ( 'NONE',  ( 8.852642474645792348, -77.09067155497332635, -8.178101815369201333 ) ) ;
#9391=CARTESIAN_POINT ( 'NONE',  ( 10.75000000000000000, -80.25000000000000000, -1.651583051307000043E-14 ) ) ;
#9399=ORIENTED_EDGE ( 'NONE', *, *, #32337, .F. ) ;
#9401=CARTESIAN_POINT ( 'NONE',  ( 9.651204802600000576, -80.43314977265349341, 5.628321366006999504 ) ) ;
#9404=CARTESIAN_POINT ( 'NONE',  ( 8.196653188619999142, -77.64368766097399543, 7.657217973713000170 ) ) ;
#9407=AXIS2_PLACEMENT_3D ( 'NONE', #5695, #23704, #1580 ) ;
#9430=CARTESIAN_POINT ( 'NONE',  ( -6.111832503000000472, -76.17462612386199794, 10.87001744695999861 ) ) ;
#9437=CARTESIAN_POINT ( 'NONE',  ( -6.043427764450786555, -78.88333333333333997, -10.48543666025110177 ) ) ;
#9463=CARTESIAN_POINT ( 'NONE',  ( -11.61454496413000115, -77.47861567637899327, 2.935712811417999557 ) ) ;
#9465=CARTESIAN_POINT ( 'NONE',  ( 8.321246128606000880, -78.19452423951800313, -8.715080868295999039 ) ) ;
#9469=CARTESIAN_POINT ( 'NONE',  ( -11.01515889844999840, -78.95448538877499800, 0.6066373079611000474 ) ) ;
#9479=DIRECTION ( 'NONE',  ( 0.000000000000000000, -1.000000000000000000, 0.000000000000000000 ) ) ;
#9482=CARTESIAN_POINT ( 'NONE',  ( -11.13008859988999966, -78.70448538877499800, 0.6129668257943999832 ) ) ;
#9484=CARTESIAN_POINT ( 'NONE',  ( 4.254218938430716079, -79.70414273500806246, -11.04225118825767993 ) ) ;
#9488=CARTESIAN_POINT ( 'NONE',  ( -8.035240866938249127, -76.44166666666666288, 7.229432123683928069 ) ) ;
#9498=CARTESIAN_POINT ( 'NONE',  ( 10.63720963964777688, -78.83845499315577854, -1.560381659779633168 ) ) ;
#9499=CARTESIAN_POINT ( 'NONE',  ( -5.413884141668839689, -77.68335102312344986, -9.393024699257772170 ) ) ;
#9501=CARTESIAN_POINT ( 'NONE',  ( 7.597989044191865382, -76.06501007995230168, 8.084992307224259989 ) ) ;
#9504=CARTESIAN_POINT ( 'NONE',  ( -2.562437971592963937, -76.44121971063705701, 11.92753260506139057 ) ) ;
#9505=CARTESIAN_POINT ( 'NONE',  ( 8.941640842993423988, -78.85745151639218875, 7.898998304516130275 ) ) ;
#9506=CARTESIAN_POINT ( 'NONE',  ( 3.507155896972999898, -79.11580003895399216, 10.65448112794999957 ) ) ;
#9518=CARTESIAN_POINT ( 'NONE',  ( -12.00000000000000178, -78.41041666666667709, -1.570796326794897668 ) ) ;
#9527=CARTESIAN_POINT ( 'NONE',  ( 11.10214774708000007, -79.58624754497100184, -5.597531737657999606 ) ) ;
#9529=CARTESIAN_POINT ( 'NONE',  ( -9.420416572830998092, -76.25741179485200405, -6.585164207577999917 ) ) ;
#9530=CARTESIAN_POINT ( 'NONE',  ( -7.628363392376307672, -78.03778907345090943, 7.574339073857688120 ) ) ;
#9532=CARTESIAN_POINT ( 'NONE',  ( -0.7928179559538000021, -78.75362403072900008, -11.95355612866999984 ) ) ;
#9538=CARTESIAN_POINT ( 'NONE',  ( 7.849383194069857517, -80.91008263851306026, 7.345942549935802646 ) ) ;
#9541=CARTESIAN_POINT ( 'NONE',  ( 6.099615176083999835, -78.63114111160000164, -9.019941877331000057 ) ) ;
#9542=CARTESIAN_POINT ( 'NONE',  ( 11.90625000002000000, -76.20625000001498961, 3.701036097655999965E-09 ) ) ;
#9543=CARTESIAN_POINT ( 'NONE',  ( -10.27832156847999912, -80.35961828462440337, 4.298059050626999777 ) ) ;
#9548=CARTESIAN_POINT ( 'NONE',  ( 5.151324428776999476, -77.53534689742400587, 9.964033682248000900 ) ) ;
#9556=CARTESIAN_POINT ( 'NONE',  ( 5.246383657897999875, -77.46100733245999947, -10.79237965019999912 ) ) ;
#9558=CARTESIAN_POINT ( 'NONE',  ( 9.608679508909999001, -77.00116639950799424, 5.650475968096999146 ) ) ;
#9564=CARTESIAN_POINT ( 'NONE',  ( -10.74981572755469550, -80.10331782357827990, -0.4067125980479509018 ) ) ;
#9570=CARTESIAN_POINT ( 'NONE',  ( 6.277205522164990725, -79.03065722717676067, 10.03106614420215337 ) ) ;
#9571=CARTESIAN_POINT ( 'NONE',  ( -8.320158381697998706, -78.76455857394600457, 7.590054615178000397 ) ) ;
#9576=CIRCLE ( 'NONE', #21812, 14.00000000000000000 ) ;
#9588=ORIENTED_EDGE ( 'NONE', *, *, #17784, .T. ) ;
#9602=CARTESIAN_POINT ( 'NONE',  ( -0.9849936891751999157, -80.88413894626904721, -11.22225356808999841 ) ) ;
#9609=CARTESIAN_POINT ( 'NONE',  ( 5.365883907697000410, -80.23717621672710720, 9.905345355165000143 ) ) ;
#9618=CARTESIAN_POINT ( 'NONE',  ( -3.790933506348975524, -79.50381487114017887, 10.05939893380695516 ) ) ;
#9634=CARTESIAN_POINT ( 'NONE',  ( 3.266381872689648080, -77.24970252057229914, -10.26631233854832281 ) ) ;
#9641=CARTESIAN_POINT ( 'NONE',  ( -10.75000000000000178, -80.49266322307225607, 0.9911140733791250490 ) ) ;
#9643=CARTESIAN_POINT ( 'NONE',  ( 9.752895431365999457, -78.82452710374299443, -6.878701514737999290 ) ) ;
#9648=CARTESIAN_POINT ( 'NONE',  ( 11.99999999999999822, -78.56041666666666856, 1.570796326794923203 ) ) ;
#9658=CARTESIAN_POINT ( 'NONE',  ( -1.963210506780999953, -76.37706369595299805, -11.00998129987999974 ) ) ;
#9659=CARTESIAN_POINT ( 'NONE',  ( 10.75000000000000000, -78.75000000000000000, 0.000000000000000000 ) ) ;
#9661=CARTESIAN_POINT ( 'NONE',  ( -11.12866505422999985, -76.33403960801499011, -1.495507578120999881 ) ) ;
#9683=B_SPLINE_CURVE_WITH_KNOTS ( 'NONE', 3,
 ( #2859, #12007, #38574, #43591, #20855, #29986, #16723, #47469, #11723, #16147, #34125, #39151, #21435, #34706, #12288, #34992, #17009, #53023 ),
 .UNSPECIFIED., .F., .F.,
 ( 4, 2, 2, 2, 2, 2, 2, 2, 4 ),
 ( 0.000000000000000000, 0.1250000000000000555, 0.2500000000000001110, 0.3750000000000001665, 0.5000000000000002220, 0.6250000000000002220, 0.7500000000000002220, 0.8750000000000001110, 1.000000000000000000 ),
 .UNSPECIFIED. ) ;
#9691=CARTESIAN_POINT ( 'NONE',  ( -5.785951846261999876, -80.29104072104459533, -9.693547939119000034 ) ) ;
#9692=CARTESIAN_POINT ( 'NONE',  ( 10.75000000000000000, -80.75000000000000000, 3.489821576044999869E-14 ) ) ;
#9694=CARTESIAN_POINT ( 'NONE',  ( -9.524774638983998898, -77.28961520195100832, 5.924253427062000199 ) ) ;
#9700=CARTESIAN_POINT ( 'NONE',  ( -1.147008567282696401, -76.10208333332839459, 10.94791666671693164 ) ) ;
#9718=EDGE_CURVE ( 'NONE', #7434, #46988, #19640, .T. ) ;
#9740=CARTESIAN_POINT ( 'NONE',  ( -11.94395460750000204, -77.18299661749800578, 2.857367593729999822 ) ) ;
#9741=CARTESIAN_POINT ( 'NONE',  ( 11.70000000000000107, -80.79999999999999716, 0.000000000000000000 ) ) ;
#9748=VERTEX_POINT ( 'NONE', #45475 ) ;
#9755=CARTESIAN_POINT ( 'NONE',  ( 11.43454631689000145, -77.73332587731398746, -3.800910706745999956 ) ) ;
#9758=CARTESIAN_POINT ( 'NONE',  ( 9.892383529026000488, -79.17237613278999220, -4.882876457188000785 ) ) ;
#9766=CARTESIAN_POINT ( 'NONE',  ( -9.904718956742000202, -75.92565473334099124, -7.632293584405999809 ) ) ;
#9771=CARTESIAN_POINT ( 'NONE',  ( 3.350422000336999773, -79.35815762081898583, -10.63152260923000014 ) ) ;
#9773=CARTESIAN_POINT ( 'NONE',  ( -12.00000000000000000, -77.39999999999999147, 0.000000000000000000 ) ) ;
#9780=CARTESIAN_POINT ( 'NONE',  ( 13.89999999999999858, -80.79999999999999716, 0.000000000000000000 ) ) ;
#9791=CARTESIAN_POINT ( 'NONE',  ( 7.614890194919533783, -78.78764436229195667, -7.587871591982528585 ) ) ;
#9800=CARTESIAN_POINT ( 'NONE',  ( -3.545693839590635221, -77.44881410897738760, 11.44325331982801863 ) ) ;
#9801=CARTESIAN_POINT ( 'NONE',  ( 2.179295889402999897, -78.62554586492200315, 11.00312592022000047 ) ) ;
#9802=CARTESIAN_POINT ( 'NONE',  ( 1.426370643901660129, -81.00000000000002842, 10.71686120634390171 ) ) ;
#9803=VERTEX_POINT ( 'NONE', #23317 ) ;
#9810=CARTESIAN_POINT ( 'NONE',  ( 12.00000000000000711, -77.63958333333333428, -1.570796326794872355 ) ) ;
#9811=CARTESIAN_POINT ( 'NONE',  ( -10.47020627418440242, -80.97916666666665719, 2.813789756862221214 ) ) ;
#9816=VECTOR ( 'NONE', #43412, 1000.000000000000000 ) ;
#9820=CARTESIAN_POINT ( 'NONE',  ( 7.691874984900000101, -79.55148891412299861, -9.768577294637001529 ) ) ;
#9821=CARTESIAN_POINT ( 'NONE',  ( 0.1582166208049999856, -76.01502919452599372, 11.37418021090000053 ) ) ;
#9822=CARTESIAN_POINT ( 'NONE',  ( 10.43518326032827126, -77.86936012529750428, 2.584052442912811109 ) ) ;
#9823=CARTESIAN_POINT ( 'NONE',  ( 6.917788961650999546, -78.80788266157699695, -9.780606322222999083 ) ) ;
#9826=ADVANCED_FACE ( 'NONE', ( #909 ), #54040, .F. ) ;
#9830=CARTESIAN_POINT ( 'NONE',  ( 4.104553908884746249, -80.94404747578096249, 9.935402628773564615 ) ) ;
#9833=CARTESIAN_POINT ( 'NONE',  ( -0.9453041629244000044, -78.27289305516799800, 11.10679974661999836 ) ) ;
#9834=CARTESIAN_POINT ( 'NONE',  ( 10.16964605767000052, -76.35263817687363996, -6.884832982024001069 ) ) ;
#9835=CARTESIAN_POINT ( 'NONE',  ( -6.468715003314000178, -80.88375601109909496, 8.928767417134999107 ) ) ;
#9840=B_SPLINE_CURVE_WITH_KNOTS ( 'NONE', 3,
 ( #54720, #19578, #29014, #55892, #32259, #28714, #50599, #19293, #19879, #33138, #37872, #36993, #6288, #24303, #42018, #46466, #55594, #50888 ),
 .UNSPECIFIED., .F., .F.,
 ( 4, 2, 2, 2, 2, 2, 2, 2, 4 ),
 ( 0.000000000000000000, 0.1249999999999999722, 0.2499999999999999445, 0.3749999999999998890, 0.4999999999999998890, 0.6249999999999998890, 0.7499999999999997780, 0.8749999999999998890, 1.000000000000000000 ),
 .UNSPECIFIED. ) ;
#9842=CARTESIAN_POINT ( 'NONE',  ( -10.05535668103000191, -78.22957133974199451, 4.970705447719999448 ) ) ;
#9851=CARTESIAN_POINT ( 'NONE',  ( -11.16978667388999824, -77.28678420793599457, -1.438690452479999937 ) ) ;
#9858=CARTESIAN_POINT ( 'NONE',  ( -7.555765981425745181, -80.16344139804368751, -7.646384711791143651 ) ) ;
#9862=CARTESIAN_POINT ( 'NONE',  ( -2.693529710394999999, -79.78555764342200973, 10.81663063389000001 ) ) ;
#9875=B_SPLINE_CURVE_WITH_KNOTS ( 'NONE', 3,
 ( #10721, #24285, #28404, #2156, #20157, #46160, #23985, #24866, #14830, #6567, #16010, #5686, #46451, #41709, #50872, #10418, #5979, #42002, #1570, #28699, #6269, #1868, #19863 ),
 .UNSPECIFIED., .F., .F.,
 ( 4, 2, 2, 2, 2, 2, 1, 2, 2, 2, 2, 4 ),
 ( 0.000000000000000000, 0.1249999999999999722, 0.2500000000000000000, 0.3750000000000000000, 0.5000000000000001110, 0.5625000000000001110, 0.6250000000000001110, 0.6875000000000001110, 0.7500000000000000000, 0.8125000000000000000, 0.8750000000000000000, 1.000000000000000000 ),
 .UNSPECIFIED. ) ;
#9894=CARTESIAN_POINT ( 'NONE',  ( -11.09105850093000001, -80.18429898691658764, 1.974238845993000258 ) ) ;
#9897=CARTESIAN_POINT ( 'NONE',  ( 5.969195881079206956, -76.15416666614690655, -10.35833566983218113 ) ) ;
#9912=CARTESIAN_POINT ( 'NONE',  ( -8.508616545356863625, -79.54773900155933575, 6.572652578013081559 ) ) ;
#9915=VECTOR ( 'NONE', #40824, 1000.000000000000000 ) ;
#9924=CARTESIAN_POINT ( 'NONE',  ( 5.209925396217442994, -77.11090969355151969, -10.71737960282440838 ) ) ;
#9927=CARTESIAN_POINT ( 'NONE',  ( -7.388662270317944980, -77.16469925202929403, -7.808743162194972776 ) ) ;
#9932=CARTESIAN_POINT ( 'NONE',  ( -8.734850699938000673, -79.64135281726700555, 8.271005326623001253 ) ) ;
#9933=CARTESIAN_POINT ( 'NONE',  ( -8.359900899578630415E-07, -76.12787248224110215, -11.82848710057588626 ) ) ;
#9936=CARTESIAN_POINT ( 'NONE',  ( 4.358044849164000922, -77.27815612458898897, -11.11047130621000001 ) ) ;
#9951=CARTESIAN_POINT ( 'NONE',  ( -11.26971213774734082, -79.79999999999996874, -3.998637387020187006 ) ) ;
#9954=CARTESIAN_POINT ( 'NONE',  ( 1.849737152796000039, -76.56009456256700219, 11.02961253862999946 ) ) ;
#9957=CARTESIAN_POINT ( 'NONE',  ( -5.300820900011999903, -76.40928543398199224, -9.898738636383001221 ) ) ;
#9988=EDGE_CURVE ( 'NONE', #49218, #15698, #3660, .T. ) ;
#9990=CARTESIAN_POINT ( 'NONE',  ( 10.10893382724000134, -80.98827613352290200, -5.281770763473000230 ) ) ;
#9993=CARTESIAN_POINT ( 'NONE',  ( -3.633103876188000125, -77.30293106922299273, 10.61219425078000000 ) ) ;
#9998=CARTESIAN_POINT ( 'NONE',  ( 9.472494285633610289, -80.99999999999998579, -5.606341685433056554 ) ) ;
#10010=CARTESIAN_POINT ( 'NONE',  ( 10.96171043400000045, -78.53938061935399162, -5.535041421897999747 ) ) ;
#10014=CARTESIAN_POINT ( 'NONE',  ( 12.00000000000000000, -79.14999999999999147, 0.000000000000000000 ) ) ;
#10020=CARTESIAN_POINT ( 'NONE',  ( 2.343379474233999726, -79.93084841004029784, 10.44606179296999926 ) ) ;
#10021=CARTESIAN_POINT ( 'NONE',  ( 4.706446445480565177E-05, -80.72503824655814242, -10.81748136418979556 ) ) ;
#10030=EDGE_LOOP ( 'NONE', ( #41450, #9332, #23209 ) ) ;
#10037=CARTESIAN_POINT ( 'NONE',  ( 11.13784153760999907, -76.41850151303799521, 5.174080857020999957 ) ) ;
#10038=CIRCLE ( 'NONE', #6998, 11.05000000000000071 ) ;
#10044=CARTESIAN_POINT ( 'NONE',  ( -0.2721098858049000313, -79.12693104276253564, 11.21356619464000026 ) ) ;
#10052=CARTESIAN_POINT ( 'NONE',  ( -3.532272164985999829, -77.47550115664098769, 11.39993665757999963 ) ) ;
#10055=CARTESIAN_POINT ( 'NONE',  ( 3.449307203194000415, -79.30855784779899409, 10.47874105986000082 ) ) ;
#10063=CARTESIAN_POINT ( 'NONE',  ( -10.25000000000000000, -82.09999999999999432, 0.000000000000000000 ) ) ;
#10064=CARTESIAN_POINT ( 'NONE',  ( -11.68767212001980127, -77.87916666666664867, 3.140974612311317138 ) ) ;
#10069=CARTESIAN_POINT ( 'NONE',  ( 5.709935245961999861, -78.54106733076498870, 9.573465417320001336 ) ) ;
#10071=CARTESIAN_POINT ( 'NONE',  ( -2.813789756862300262, -79.89583333333330017, 10.47020627418438465 ) ) ;
#10078=AXIS2_PLACEMENT_3D ( 'NONE', #13489, #13189, #31479 ) ;
#10088=CARTESIAN_POINT ( 'NONE',  ( 9.947560812465606972, -78.81912883275374782, -4.075256179118199817 ) ) ;
#10094=CARTESIAN_POINT ( 'NONE',  ( 11.41797009976014365, -76.32802149572208350, 4.296752358342962985 ) ) ;
#10095=CARTESIAN_POINT ( 'NONE',  ( 11.81395210335005608, -77.31316753185872415, 1.987591828291500384 ) ) ;
#10096=CARTESIAN_POINT ( 'NONE',  ( -11.20683111097000051, -79.83726082427419612, -0.4743912329535999728 ) ) ;
#10097=ORIENTED_EDGE ( 'NONE', *, *, #17538, .T. ) ;
#10102=CARTESIAN_POINT ( 'NONE',  ( 11.00000000012632739, -76.04999999999999716, 1.151917305286630722 ) ) ;
#10104=CARTESIAN_POINT ( 'NONE',  ( -11.68767212001978706, -77.42083333333333428, -3.140974612311364655 ) ) ;
#10115=CARTESIAN_POINT ( 'NONE',  ( 4.822953412158000219, -79.03010945140999866, -11.45989370067999857 ) ) ;
#10116=CARTESIAN_POINT ( 'NONE',  ( 7.124885535347999621, -76.25294931795998821, -8.714606029085999239 ) ) ;
#10117=CARTESIAN_POINT ( 'NONE',  ( 10.05221862648209274, -77.87898788867025246, 3.817045573893846022 ) ) ;
#10118=CARTESIAN_POINT ( 'NONE',  ( 2.956870837876000468, -78.92095621112599702, 11.44999256673999888 ) ) ;
#10124=CARTESIAN_POINT ( 'NONE',  ( 6.018017909193484449, -80.92806936818854524, 8.908428929804006913 ) ) ;
#10127=CARTESIAN_POINT ( 'NONE',  ( -10.89229298341999908, -77.37409373610799435, 2.369082973246999568 ) ) ;
#10129=CARTESIAN_POINT ( 'NONE',  ( -5.340898366833999766, -80.30592291261719140, 9.777117507691999165 ) ) ;
#10135=CARTESIAN_POINT ( 'NONE',  ( 11.19180402071999936, -77.45363786841799936, 0.7494220128532999015 ) ) ;
#10145=CARTESIAN_POINT ( 'NONE',  ( -7.743768518152000624, -77.34125689393900416, -8.177286450628999503 ) ) ;
#10151=CARTESIAN_POINT ( 'NONE',  ( -7.590654613722642274, -80.16307491009121122, -7.611717479442802414 ) ) ;
#10156=DIRECTION ( 'NONE',  ( 0.000000000000000000, 0.000000000000000000, 1.000000000000000000 ) ) ;
#10157=CARTESIAN_POINT ( 'NONE',  ( 7.779872909029999839, -79.77157567883000411, 7.821464818102998429 ) ) ;
#10164=VERTEX_POINT ( 'NONE', #16282 ) ;
#10171=CARTESIAN_POINT ( 'NONE',  ( 8.596418555780450887, -78.19791666666668561, -6.606377239730321982 ) ) ;
#10174=ORIENTED_EDGE ( 'NONE', *, *, #26394, .T. ) ;
#10185=B_SPLINE_CURVE_WITH_KNOTS ( 'NONE', 3,
 ( #1624, #37904, #28456, #46504, #37320, #5738, #42638, #15479, #15764, #55337, #33470, #42352, #47376, #23745, #33759, #42052, #19615, #37613 ),
 .UNSPECIFIED., .F., .F.,
 ( 4, 2, 2, 2, 2, 2, 2, 2, 4 ),
 ( 0.000000000000000000, 0.1250000000000000000, 0.2500000000000000000, 0.3750000000000000000, 0.5000000000000000000, 0.6250000000000000000, 0.7500000000000000000, 0.8750000000000000000, 1.000000000000000000 ),
 .UNSPECIFIED. ) ;
#10188=CARTESIAN_POINT ( 'NONE',  ( -2.895922040489999905, -80.16179448218190373, 10.88681414971999928 ) ) ;
#10196=VERTEX_POINT ( 'NONE', #52583 ) ;
#10199=DIRECTION ( 'NONE',  ( -1.156375342703999878E-13, -0.000000000000000000, -1.000000000000000000 ) ) ;
#10203=CARTESIAN_POINT ( 'NONE',  ( 8.082598614575715601, -79.40746475772557744, 7.120178426330225463 ) ) ;
#10221=CARTESIAN_POINT ( 'NONE',  ( -7.858171174022000827, -79.13333109285899525, 9.108036400545000077 ) ) ;
#10225=CARTESIAN_POINT ( 'NONE',  ( -9.926966510012999123, -77.57657859425000879, 6.625016102256999773 ) ) ;
#10239=CARTESIAN_POINT ( 'NONE',  ( -6.332001867507876192, -79.79999999999999716, -10.05727774830502952 ) ) ;
#10243=CARTESIAN_POINT ( 'NONE',  ( 8.154961773732001262, -76.00829183880699702, 7.653135223926000208 ) ) ;
#10251=DIRECTION ( 'NONE',  ( 0.000000000000000000, 0.000000000000000000, -1.000000000000000000 ) ) ;
#10255=AXIS2_PLACEMENT_3D ( 'NONE', #5097, #41689, #14228 ) ;
#10258=CARTESIAN_POINT ( 'NONE',  ( -6.043427764450833628, -79.31666666666667709, 10.48543666025107335 ) ) ;
#10268=CARTESIAN_POINT ( 'NONE',  ( 4.570427068259999892, -77.21806133255499560, 11.39767413300000065 ) ) ;
#10275=CARTESIAN_POINT ( 'NONE',  ( 11.36098558129999958, -80.53363121547570813, 1.007794481568000222 ) ) ;
#10278=CARTESIAN_POINT ( 'NONE',  ( 6.329984427697000093, -78.22896673128499856, 9.260097609460000712 ) ) ;
#10284=CARTESIAN_POINT ( 'NONE',  ( 10.49753343895564228, -81.00000000000001421, -3.287627937531071964 ) ) ;
#10288=CARTESIAN_POINT ( 'NONE',  ( 10.07210119001000059, -80.48527584695288795, 5.045985883512999592 ) ) ;
#10296=VERTEX_POINT ( 'NONE', #44224 ) ;
#10297=CARTESIAN_POINT ( 'NONE',  ( -0.8050603620646999969, -78.87859328629799904, -12.13813858862000217 ) ) ;
#10311=ORIENTED_EDGE ( 'NONE', *, *, #41008, .F. ) ;
#10316=CARTESIAN_POINT ( 'NONE',  ( -10.86658628928999981, -76.76993982145202722, -2.781249891074999869 ) ) ;
#10326=CARTESIAN_POINT ( 'NONE',  ( 11.61133755414000035, -76.91029437269800439, 3.999933378912999604 ) ) ;
#10330=CARTESIAN_POINT ( 'NONE',  ( 3.113304451009999863, -78.39783470746900207, -10.55022916317000181 ) ) ;
#10331=VERTEX_POINT ( 'NONE', #48946 ) ;
#10338=AXIS2_PLACEMENT_3D ( 'NONE', #52132, #57124, #48004 ) ;
#10339=CARTESIAN_POINT ( 'NONE',  ( 10.38571723084000098, -77.28559594867499527, -5.879822389739000066 ) ) ;
#10342=CARTESIAN_POINT ( 'NONE',  ( 10.84306248592000088, -79.26733954020500050, -1.266239280945999912 ) ) ;
#10349=CARTESIAN_POINT ( 'NONE',  ( -9.596002108778193929, -77.84791666666664867, 7.374560639698937159 ) ) ;
#10355=CARTESIAN_POINT ( 'NONE',  ( -9.839357990653688546, -79.50291255989223771, 6.574323847643208651 ) ) ;
#10360=CARTESIAN_POINT ( 'NONE',  ( -1.639985762054531282, -78.73658472870678793, 11.09648843833229925 ) ) ;
#10369=ORIENTED_EDGE ( 'NONE', *, *, #1869, .T. ) ;
#10371=CARTESIAN_POINT ( 'NONE',  ( 8.590462643448541158, -78.79883893288808849, -6.463108130307494648 ) ) ;
#10374=CARTESIAN_POINT ( 'NONE',  ( -10.07624512687999996, -76.28571183916568543, -4.852130239470000106 ) ) ;
#10380=CARTESIAN_POINT ( 'NONE',  ( -11.75000000000000000, -76.04999999999999716, -3.652443742841000169E-09 ) ) ;
#10381=CARTESIAN_POINT ( 'NONE',  ( -10.26957973897401288, -78.50685741050436661, 6.168932106361120660 ) ) ;
#10382=CARTESIAN_POINT ( 'NONE',  ( -8.286771986066998608, -78.70725489392698648, 7.559597915363999832 ) ) ;
#10386=EDGE_LOOP ( 'NONE', ( #18505, #23185, #50809, #49279 ) ) ;
#10391=DIRECTION ( 'NONE',  ( -1.000000000000000000, 0.000000000000000000, 0.000000000000000000 ) ) ;
#10392=CARTESIAN_POINT ( 'NONE',  ( 12.00000000000000711, -78.63958333333333428, -1.570796326794872355 ) ) ;
#10401=ORIENTED_EDGE ( 'NONE', *, *, #57193, .F. ) ;
#10404=CARTESIAN_POINT ( 'NONE',  ( -0.7463658975004607843, -77.98057452693001323, 10.72557968341309120 ) ) ;
#10405=CARTESIAN_POINT ( 'NONE',  ( 7.483561698776000526, -78.38741300779199150, 9.354804580292000793 ) ) ;
#10410=CARTESIAN_POINT ( 'NONE',  ( 9.552523027918807585, -80.88808154937647998, 4.930511287832971767 ) ) ;
#10413=CARTESIAN_POINT ( 'NONE',  ( -7.719769492146999923, -76.89709394048399815, 7.579341418041000367 ) ) ;
#10415=CARTESIAN_POINT ( 'NONE',  ( -1.680151650566999999, -81.07168981312450740, -10.89699058823000044 ) ) ;
#10418=CARTESIAN_POINT ( 'NONE',  ( 7.103480459865705754, -80.41785787807644681, 8.098525061049892670 ) ) ;
#10419=B_SPLINE_CURVE_WITH_KNOTS ( 'NONE', 3,
 ( #32831, #55286, #23699, #55582 ),
 .UNSPECIFIED., .F., .F.,
 ( 4, 4 ),
 ( 0.000000000000000000, 1.000000000000000000 ),
 .UNSPECIFIED. ) ;
#10420=CARTESIAN_POINT ( 'NONE',  ( -7.849238557987999521, -76.70433613164000519, 7.706455349885999340 ) ) ;
#10431=CARTESIAN_POINT ( 'NONE',  ( 5.172078487859000262, -77.61362032395699373, 10.00417756108999967 ) ) ;
#10443=CARTESIAN_POINT ( 'NONE',  ( 8.679422240859999249, -78.58715855134300909, -6.994438423095999724 ) ) ;
#10458=CARTESIAN_POINT ( 'NONE',  ( -6.606377239730330864, -78.07291666666665719, -8.596418555780440229 ) ) ;
#10464=CARTESIAN_POINT ( 'NONE',  ( -8.012523733904361123, -76.96708638852499007, -8.990154430768209082 ) ) ;
#10477=CARTESIAN_POINT ( 'NONE',  ( 8.596187401860602151, -76.79807390516880616, -6.606220740437996675 ) ) ;
#10489=DIRECTION ( 'NONE',  ( 0.000000000000000000, 1.000000000000000000, 0.000000000000000000 ) ) ;
#10494=CARTESIAN_POINT ( 'NONE',  ( -2.494193680512617473, -79.49363092753210935, 10.45664570855439912 ) ) ;
#10510=CARTESIAN_POINT ( 'NONE',  ( -4.807621802239022912, -76.07083333332734298, 10.81449558221754970 ) ) ;
#10513=ORIENTED_EDGE ( 'NONE', *, *, #26492, .T. ) ;
#10514=CARTESIAN_POINT ( 'NONE',  ( 11.90415444617999974, -79.87240057246600600, -1.731350929957999885 ) ) ;
#10516=DIRECTION ( 'NONE',  ( 0.000000000000000000, 1.000000000000000000, 0.000000000000000000 ) ) ;
#10517=CARTESIAN_POINT ( 'NONE',  ( -11.70000000000000107, -76.00000000000000000, 0.000000000000000000 ) ) ;
#10520=CARTESIAN_POINT ( 'NONE',  ( -8.118170145944999305, -78.68888052662400412, -8.748189294319999476 ) ) ;
#10521=ORIENTED_EDGE ( 'NONE', *, *, #10974, .T. ) ;
#10522=ORIENTED_EDGE ( 'NONE', *, *, #50298, .T. ) ;
#10523=CARTESIAN_POINT ( 'NONE',  ( -1.407171709420465211, -78.88541666666664298, 10.74999999999999467 ) ) ;
#10527=ORIENTED_EDGE ( 'NONE', *, *, #1954, .F. ) ;
#10535=CARTESIAN_POINT ( 'NONE',  ( -5.243548408265479743, -79.79999999999998295, -10.63019555954501705 ) ) ;
#10539=CARTESIAN_POINT ( 'NONE',  ( -8.075725583014000009, -76.25911125869799889, -7.736700848913999451 ) ) ;
#10540=CARTESIAN_POINT ( 'NONE',  ( 5.112147531402400524, -76.43689203955935341, 9.547208415643030577 ) ) ;
#10552=CARTESIAN_POINT ( 'NONE',  ( -9.075114011589430874, -78.05511120107294687, 5.762976831777519848 ) ) ;
#10557=CARTESIAN_POINT ( 'NONE',  ( -1.570796326794937636, -79.28541666666666288, 11.99999999999999467 ) ) ;
#10566=CARTESIAN_POINT ( 'NONE',  ( 4.484119338316999936, -77.02815612458898897, -11.43188768503999952 ) ) ;
#10572=CARTESIAN_POINT ( 'NONE',  ( 7.638540051645000162, -81.09319419153379727, 8.469952564609000589 ) ) ;
#10575=CARTESIAN_POINT ( 'NONE',  ( 10.29113596735999892, -77.68423987124899099, 4.462133020506000136 ) ) ;
#10580=CARTESIAN_POINT ( 'NONE',  ( 4.483565756030909455, -76.07604166666334322, 10.08190381434128824 ) ) ;
#10582=DIRECTION ( 'NONE',  ( 1.000000000000000000, 0.000000000000000000, 0.000000000000000000 ) ) ;
#10583=CARTESIAN_POINT ( 'NONE',  ( 1.618170588614999961, -80.33478741693470226, -11.14857479085000058 ) ) ;
#10591=CARTESIAN_POINT ( 'NONE',  ( 3.002529760384999857, -79.11371401997000419, 11.62679918156999825 ) ) ;
#10598=CARTESIAN_POINT ( 'NONE',  ( -6.605942102368285163, -77.67293223250510437, -8.595925543322636031 ) ) ;
#10602=EDGE_CURVE ( 'NONE', #4925, #44663, #49738, .T. ) ;
#10604=VERTEX_POINT ( 'NONE', #14027 ) ;
#10608=CARTESIAN_POINT ( 'NONE',  ( 0.000000000000000000, -76.10312499993298729, -11.80312499993000053 ) ) ;
#10622=CARTESIAN_POINT ( 'NONE',  ( -3.164411967817999827, -77.23815627913698734, -11.86639179494000018 ) ) ;
#10626=CARTESIAN_POINT ( 'NONE',  ( -11.06493808903000087, -79.26311275777169385, -1.839906431680000010 ) ) ;
#10628=CARTESIAN_POINT ( 'NONE',  ( 0.000000000000000000, -76.10312499993298729, 0.000000000000000000 ) ) ;
#10635=CARTESIAN_POINT ( 'NONE',  ( -8.937463246932001226, -77.95036040070399963, 8.081925660605000061 ) ) ;
#10646=CARTESIAN_POINT ( 'NONE',  ( -12.11464257907000075, -79.76545167379698853, -1.005257255610999989 ) ) ;
#10654=DIRECTION ( 'NONE',  ( -1.000000000000000000, 0.000000000000000000, 0.000000000000000000 ) ) ;
#10656=CARTESIAN_POINT ( 'NONE',  ( -0.2732061834123999944, -79.15352125521398818, 11.25874428786999992 ) ) ;
#10658=CARTESIAN_POINT ( 'NONE',  ( -11.08419787132735124, -76.36051769991946969, -1.489531927970142000 ) ) ;
#10659=CARTESIAN_POINT ( 'NONE',  ( 10.75000000000000000, -79.75000000000000000, 0.000000000000000000 ) ) ;
#10665=CARTESIAN_POINT ( 'NONE',  ( 9.376568502766771118, -79.55367501876179404, -6.156425267692819503 ) ) ;
#10673=ORIENTED_EDGE ( 'NONE', *, *, #15474, .F. ) ;
#10675=CARTESIAN_POINT ( 'NONE',  ( 8.973809496257258544, -78.80375026939715610, -5.918774935595488174 ) ) ;
#10682=CARTESIAN_POINT ( 'NONE',  ( -8.149016987013476765, -78.61537467219939401, -8.781430036993665311 ) ) ;
#10684=CARTESIAN_POINT ( 'NONE',  ( 11.21485848424000054, -80.15017646456679756, -0.2123177049684000228 ) ) ;
#10690=CARTESIAN_POINT ( 'NONE',  ( 11.19195961368080461, -77.60522894247633019, 0.7494324316197222835 ) ) ;
#10693=CARTESIAN_POINT ( 'NONE',  ( -7.374560639698973574, -77.47291666666666288, -9.596002108778167283 ) ) ;
#10703=EDGE_LOOP ( 'NONE', ( #38288, #24157, #39616, #39345, #10673, #56164 ) ) ;
#10705=CARTESIAN_POINT ( 'NONE',  ( 6.194304543013999798, -76.10681943937400717, 9.822204756253000824 ) ) ;
#10706=CARTESIAN_POINT ( 'NONE',  ( 9.532032162674793696, -77.88842254387341768, 4.970338045911559810 ) ) ;
#10707=CARTESIAN_POINT ( 'NONE',  ( 2.228685126279000173, -77.99400319886400723, 11.77068507108999995 ) ) ;
#10714=CARTESIAN_POINT ( 'NONE',  ( -9.301504212792000459, -78.50403817759199399, -5.931589059777999218 ) ) ;
#10721=CARTESIAN_POINT ( 'NONE',  ( -10.75000000000000000, -80.59999999999999432, 0.000000000000000000 ) ) ;
#10722=CARTESIAN_POINT ( 'NONE',  ( 0.2654799511899000319, -78.46077795102900154, -11.21373274707999990 ) ) ;
#10726=CARTESIAN_POINT ( 'NONE',  ( -2.486393044377000372, -77.11762553470499881, -12.01527121392999931 ) ) ;
#10735=CARTESIAN_POINT ( 'NONE',  ( 7.228832758458999308, -77.09612980692300255, 8.635852100895000660 ) ) ;
#10738=DIRECTION ( 'NONE',  ( 0.000000000000000000, 1.000000000000000000, 0.000000000000000000 ) ) ;
#10747=CARTESIAN_POINT ( 'NONE',  ( 11.02987528609000023, -80.20735716685899774, -0.2088156359816000229 ) ) ;
#10768=CARTESIAN_POINT ( 'NONE',  ( 10.75000000000000000, -76.85000000000000853, 0.000000000000000000 ) ) ;
#10783=CARTESIAN_POINT ( 'NONE',  ( -10.97713377773999888, -78.34134770576399376, -2.517240518847000175 ) ) ;
#10793=CARTESIAN_POINT ( 'NONE',  ( 7.344871482613403835, -79.41513455956103940, 7.849784798595977442 ) ) ;
#10805=CARTESIAN_POINT ( 'NONE',  ( 5.137083998358000336, -77.21100733245999947, -10.56753840748999984 ) ) ;
#10806=CARTESIAN_POINT ( 'NONE',  ( 5.627879961911095741, -80.26928327484587555, -9.165441168818450279 ) ) ;
#10808=CARTESIAN_POINT ( 'NONE',  ( -6.241704289952512141, -77.17585973208710470, -8.752229220649864416 ) ) ;
#10812=CARTESIAN_POINT ( 'NONE',  ( 10.52307592342000042, -79.42414610975299638, 5.828552047478999576 ) ) ;
#10819=CARTESIAN_POINT ( 'NONE',  ( -11.88268207399999987, -77.63083722509800566, -1.112370969927999997 ) ) ;
#10829=VERTEX_POINT ( 'NONE', #14314 ) ;
#10834=CARTESIAN_POINT ( 'NONE',  ( -9.614379292984539305, -79.79999999999998295, -7.044348044756020499 ) ) ;
#10838=CARTESIAN_POINT ( 'NONE',  ( 7.995633008690000487, -76.50993067858900076, 7.819446035993999899 ) ) ;
#10841=CARTESIAN_POINT ( 'NONE',  ( 7.809513865093999918, -76.50961320193900406, -8.068161004599000208 ) ) ;
#10846=AXIS2_PLACEMENT_3D ( 'NONE', #32814, #50861, #5967 ) ;
#10849=B_SPLINE_CURVE_WITH_KNOTS ( 'NONE', 3,
 ( #54700, #46744, #37555, #33119, #32823, #37264, #28400, #41704, #41997, #1280, #50283, #32530, #51161, #55872, #15423, #42297, #19273, #19557, #5112, #55278, #27815, #46446, #19857, #15121, #1862, #9834, #28106, #713, #33415, #14824, #51453, #50868, #14244, #50573, #32240 ),
 .UNSPECIFIED., .F., .F.,
 ( 4, 1, 1, 1, 1, 1, 1, 1, 1, 1, 1, 1, 1, 1, 1, 1, 1, 1, 1, 1, 1, 1, 1, 1, 1, 1, 1, 1, 1, 1, 1, 1, 4 ),
 ( 0.000000000000000000, 0.01250277026799517452, 0.04500258559214889015, 0.07750240091630128392, 0.1100022162404669240, 0.1425020315645531277, 0.1750018468888378809, 0.2075016622129902677, 0.2400014775371426823, 0.2725012928612950969, 0.3050011081854474559, 0.3375009235095998705, 0.3700007388337522296, 0.4025005541579046442, 0.4350003694820570588, 0.4675001848062094179, 0.5000000001303618324, 0.5324998154545141915, 0.5649996307786665506, 0.5974994461028189097, 0.6299992614269713798, 0.6624990767511239609, 0.6949988920752763200, 0.7274987073994286790, 0.7599985227235809271, 0.7924983380477335082, 0.8249981533718857563, 0.8574979686960381153, 0.8899977840201905854, 0.9224975993443429445, 0.9549974146684953036, 0.9874972299926477737, 1.000000000000000000 ),
 .UNSPECIFIED. ) ;
#10851=CARTESIAN_POINT ( 'NONE',  ( -3.771648689937000309, -79.40887399616899245, 11.60274953364999995 ) ) ;
#10852=CARTESIAN_POINT ( 'NONE',  ( -9.469160009696521385, -78.06080311739077615, 5.094555813102688013 ) ) ;
#10872=CARTESIAN_POINT ( 'NONE',  ( 10.00561547635000004, -80.92054906910999534, -5.227788429194999864 ) ) ;
#10874=DIRECTION ( 'NONE',  ( 0.000000000000000000, -1.000000000000000000, 0.000000000000000000 ) ) ;
#10875=CARTESIAN_POINT ( 'NONE',  ( -4.647088938219000376, -78.31067576028999611, 10.20895072913000057 ) ) ;
#10889=CARTESIAN_POINT ( 'NONE',  ( 10.85897810694999954, -78.47165355494099970, -5.483167429328999809 ) ) ;
#10894=EDGE_LOOP ( 'NONE', ( #7418, #41672, #13119, #968 ) ) ;
#10901=CARTESIAN_POINT ( 'NONE',  ( 8.414343270883998471, -78.37837685893698847, 6.955155862361000807 ) ) ;
#10902=EDGE_LOOP ( 'NONE', ( #3453, #12548, #34200, #29026 ) ) ;
#10917=CARTESIAN_POINT ( 'NONE',  ( 10.16964605767000052, -76.33653603642800078, -6.884832982024000181 ) ) ;
#10918=FACE_BOUND ( 'NONE', #38320, .T. ) ;
#10923=ORIENTED_EDGE ( 'NONE', *, *, #20680, .T. ) ;
#10930=CARTESIAN_POINT ( 'NONE',  ( -10.42801618316999956, -78.39809032934199706, 6.264104809848999977 ) ) ;
#10939=EDGE_CURVE ( 'NONE', #15494, #4925, #2575, .T. ) ;
#10947=CARTESIAN_POINT ( 'NONE',  ( 3.385018580295000135, -79.42588468523199197, -10.74130410002999980 ) ) ;
#10949=CARTESIAN_POINT ( 'NONE',  ( -11.71599595481501765, -79.05733145785083593, -1.136090037544484233 ) ) ;
#10965=CARTESIAN_POINT ( 'NONE',  ( 5.261237598753935707, -78.76578525366345218, -9.374798830089835278 ) ) ;
#10974=EDGE_CURVE ( 'NONE', #31953, #19148, #25390, .T. ) ;
#10975=CARTESIAN_POINT ( 'NONE',  ( -10.47031859815319343, -79.62086369140376974, -2.813909006929614431 ) ) ;
#10978=CARTESIAN_POINT ( 'NONE',  ( 10.63562707217000103, -80.17741280756860078, 3.563914325689000240 ) ) ;
#10980=LINE ( 'NONE', #42554, #6746 ) ;
#10984=CARTESIAN_POINT ( 'NONE',  ( 6.433884635080341141, -77.52351991347129001, -9.188402334806731631 ) ) ;
#10986=CARTESIAN_POINT ( 'NONE',  ( 3.140974612311376646, -77.54583333333334849, -11.68767212001978706 ) ) ;
#10996=CARTESIAN_POINT ( 'NONE',  ( -0.03076778114328541577, -77.97532005365077623, 10.74994462762427716 ) ) ;
#10997=CARTESIAN_POINT ( 'NONE',  ( 9.148490208346998998, -77.93974456801599615, 7.734416031130999514 ) ) ;
#10999=CARTESIAN_POINT ( 'NONE',  ( 10.68072966837468130, -78.86055855974642270, 1.407246846443371613 ) ) ;
#11001=CARTESIAN_POINT ( 'NONE',  ( 8.172550279481720636, -80.90660285001109742, 6.983378171755568076 ) ) ;
#11003=ADVANCED_BREP_SHAPE_REPRESENTATION ( '', ( #36141, #43526 ), #23620 ) ;
#11005=CARTESIAN_POINT ( 'NONE',  ( 0.5383385070467999745, -77.08774834149699018, -11.01870799087000030 ) ) ;
#11007=CARTESIAN_POINT ( 'NONE',  ( 1.570796326794909881, -78.43541666666668277, -11.99999999999999822 ) ) ;
#11014=CARTESIAN_POINT ( 'NONE',  ( 7.508079800428999917, -76.94946321865599259, -8.333477563431999968 ) ) ;
#11019=CARTESIAN_POINT ( 'NONE',  ( 12.07337922597999835, -76.31749961810498917, -1.385301795592000174 ) ) ;
#11025=CARTESIAN_POINT ( 'NONE',  ( 12.09999999997999964, -92.79999999999999716, 2.688172647412999614E-10 ) ) ;
#11041=CARTESIAN_POINT ( 'NONE',  ( -8.235122208958999934, -78.83228563835899649, 7.512480467459000444 ) ) ;
#11055=CARTESIAN_POINT ( 'NONE',  ( -8.982117338527000783, -79.64721103171800110, 6.718606902359000266 ) ) ;
#11073=CARTESIAN_POINT ( 'NONE',  ( -12.00000000000000000, -77.39999999999999147, 0.000000000000000000 ) ) ;
#11089=CARTESIAN_POINT ( 'NONE',  ( -9.700000000000001066, -87.20000000000000284, 0.000000000000000000 ) ) ;
#11090=CARTESIAN_POINT ( 'NONE',  ( 7.511969992774096383, -79.41342506424436465, 7.689912663504889778 ) ) ;
#11094=B_SPLINE_CURVE_WITH_KNOTS ( 'NONE', 3,
 ( #54445, #35828, #53556, #13981, #54146, #35230, #44123, #3672, #22554, #13686, #21673, #31683, #3953, #39678, #53260, #44701, #57685, #26966 ),
 .UNSPECIFIED., .F., .F.,
 ( 4, 2, 2, 2, 2, 2, 2, 2, 4 ),
 ( 0.000000000000000000, 0.1250000000000000000, 0.2499999999999999722, 0.3750000000000000000, 0.5000000000000000000, 0.6250000000000000000, 0.7500000000000000000, 0.8750000000000000000, 1.000000000000000000 ),
 .UNSPECIFIED. ) ;
#11102=CARTESIAN_POINT ( 'NONE',  ( 8.658023998471257698, -80.29953180223905918, -6.377467274757659510 ) ) ;
#11103=CARTESIAN_POINT ( 'NONE',  ( -6.959349728372989041, -77.16901490944738384, -8.193258774412282008 ) ) ;
#11107=CARTESIAN_POINT ( 'NONE',  ( 7.520016693046000178, -79.74484475749498813, -9.389162645085001202 ) ) ;
#11128=CARTESIAN_POINT ( 'NONE',  ( 11.66152884693005731, -79.80000000000001137, 1.849687133078396606 ) ) ;
#11130=CARTESIAN_POINT ( 'NONE',  ( 10.75000000000000000, -78.35000000000000853, 1.923335087985999915E-14 ) ) ;
#11132=CARTESIAN_POINT ( 'NONE',  ( -10.67244467921999984, -76.81272073173599324, 2.904229794498999873 ) ) ;
#11134=CARTESIAN_POINT ( 'NONE',  ( -6.551127804292855572, -76.52735550355730254, 8.658837545241746980 ) ) ;
#11137=CARTESIAN_POINT ( 'NONE',  ( -5.246643863826999876, -76.47701249839499837, -9.797568585289999632 ) ) ;
#11145=CARTESIAN_POINT ( 'NONE',  ( 10.89405075708000048, -79.72170167379699990, -5.492612443427000279 ) ) ;
#11146=CARTESIAN_POINT ( 'NONE',  ( -10.54835816730423304, -78.08464500269199959, 2.072073882157521307 ) ) ;
#11151=CARTESIAN_POINT ( 'NONE',  ( 12.00000000000000000, -79.16041666666664867, 1.570796326794922093 ) ) ;
#11167=CARTESIAN_POINT ( 'NONE',  ( -10.58728162385000005, -77.87489427226098826, 3.705074683290000337 ) ) ;
#11181=CARTESIAN_POINT ( 'NONE',  ( -3.634457760627999523, -77.72550115664098769, 11.72972702006000034 ) ) ;
#11192=CARTESIAN_POINT ( 'NONE',  ( 7.599690325503999588, -78.75968566096200618, -7.837095951096998192 ) ) ;
#11194=ORIENTED_EDGE ( 'NONE', *, *, #45937, .F. ) ;
#11208=CARTESIAN_POINT ( 'NONE',  ( 12.07535958108000074, -76.80152308111600234, -2.237927141218000404 ) ) ;
#11211=CARTESIAN_POINT ( 'NONE',  ( 0.9578316561261159823, -78.88180395574651982, -11.17589679220000143 ) ) ;
#11218=CARTESIAN_POINT ( 'NONE',  ( 12.13705548371000020, -78.69651279900399743, 0.8212409526314999875 ) ) ;
#11228=CARTESIAN_POINT ( 'NONE',  ( 8.596418555780418913, -77.30208333333331439, 6.606377239730356621 ) ) ;
#11232=CARTESIAN_POINT ( 'NONE',  ( 12.00000000000000711, -78.13958333333333428, -1.570796326794872355 ) ) ;
#11236=CARTESIAN_POINT ( 'NONE',  ( -9.845147265217999433, -79.31693931322499225, -5.468732932272000191 ) ) ;
#11238=AXIS2_PLACEMENT_3D ( 'NONE', #14585, #49461, #45908 ) ;
#11239=CARTESIAN_POINT ( 'NONE',  ( 10.96304720905350472, -79.33042955265048590, 4.455755102610416074 ) ) ;
#11251=CARTESIAN_POINT ( 'NONE',  ( -12.09770333016000166, -77.34888712250798903, -3.481192270638000075 ) ) ;
#11252=CARTESIAN_POINT ( 'NONE',  ( 2.115012927989350811, -78.74089074757185358, -10.53979812572510255 ) ) ;
#11262=CARTESIAN_POINT ( 'NONE',  ( 3.371435477143000181, -79.48318836525099584, -10.69820234502000034 ) ) ;
#11263=EDGE_CURVE ( 'NONE', #3715, #30430, #55707, .T. ) ;
#11269=AXIS2_PLACEMENT_3D ( 'NONE', #44390, #13675, #31672 ) ;
#11270=CARTESIAN_POINT ( 'NONE',  ( 3.113304451009999863, -78.49783470746899638, -10.55022916317000181 ) ) ;
#11273=CYLINDRICAL_SURFACE ( 'NONE', #29446, 10.75000000000000000 ) ;
#11279=CARTESIAN_POINT ( 'NONE',  ( 6.536979956083999177, -79.32071718295554774, -10.09826910480999906 ) ) ;
#11282=CARTESIAN_POINT ( 'NONE',  ( -0.4777645602529999591, -78.99535082056300439, -12.42424180296999836 ) ) ;
#11285=CARTESIAN_POINT ( 'NONE',  ( 6.035966914210000311, -77.96687388343998748, 10.34809972146999968 ) ) ;
#11289=CARTESIAN_POINT ( 'NONE',  ( 9.577959642148309527, -80.88765258768701472, 4.880894207245643379 ) ) ;
#11292=CARTESIAN_POINT ( 'NONE',  ( 10.58169901997000117, -78.23167474757299544, 3.119195446298999919 ) ) ;
#11294=CARTESIAN_POINT ( 'NONE',  ( -8.105251711770002032, -80.46822472744669597, 7.304004154415999039 ) ) ;
#11300=CARTESIAN_POINT ( 'NONE',  ( -5.859445663532000914, -77.68484447970500639, 9.564779511708000115 ) ) ;
#11313=CARTESIAN_POINT ( 'NONE',  ( -7.374560639698971798, -76.87291666666666856, -9.596002108778163731 ) ) ;
#11314=CARTESIAN_POINT ( 'NONE',  ( 9.596002108778172612, -79.49791666666665435, -7.374560639698962028 ) ) ;
#11333=CARTESIAN_POINT ( 'NONE',  ( 1.589707373765000042, -77.71003890373799550, -10.80037945888999928 ) ) ;
#11343=PLANE ( 'NONE',  #57444 ) ;
#11357=CARTESIAN_POINT ( 'NONE',  ( 10.74995922344125532, -76.84496094653090381, -0.7036252426051674558 ) ) ;
#11374=CARTESIAN_POINT ( 'NONE',  ( -6.606527024733162001, -77.02724138212725791, 8.596707079130210261 ) ) ;
#11380=MECHANICAL_DESIGN_GEOMETRIC_PRESENTATION_REPRESENTATION('',(#5834),#36932);
#11385=CARTESIAN_POINT ( 'NONE',  ( -7.585478157043000103, -77.20580276511299189, -8.010134550088000793 ) ) ;
#11390=CARTESIAN_POINT ( 'NONE',  ( 10.75315169796065895, -80.34831015543626620, -0.2582170068313175415 ) ) ;
#11393=CARTESIAN_POINT ( 'NONE',  ( -9.625846388754000671, -79.25286561624899662, -7.214584339064000318 ) ) ;
#11399=EDGE_LOOP ( 'NONE', ( #27641, #45226, #12220, #14278, #15571 ) ) ;
#11412=CARTESIAN_POINT ( 'NONE',  ( -8.014512096362414795, -79.79999999999998295, -8.788959260803750340 ) ) ;
#11413=CARTESIAN_POINT ( 'NONE',  ( -6.960157075943352645, -80.03140959141880728, 8.192335473613402641 ) ) ;
#11415=CARTESIAN_POINT ( 'NONE',  ( -4.800187936532999800, -76.31198526659200354, 10.10109298474000106 ) ) ;
#11418=CARTESIAN_POINT ( 'NONE',  ( -10.93116861664999995, -76.37668473043899553, 2.007280421741000076 ) ) ;
#11426=CARTESIAN_POINT ( 'NONE',  ( -12.18267985468999903, -79.51314988871099843, -0.6568425513276999750 ) ) ;
#11427=CARTESIAN_POINT ( 'NONE',  ( -8.955948465137943515, -78.05351281406913699, 5.945725506398519045 ) ) ;
#11447=CARTESIAN_POINT ( 'NONE',  ( 10.07210119001000059, -80.53695791176038199, 5.045985883512999592 ) ) ;
#11470=CARTESIAN_POINT ( 'NONE',  ( 9.940990682305997694, -78.95998123256899248, -7.011364793726000855 ) ) ;
#11478=ORIENTED_EDGE ( 'NONE', *, *, #35451, .F. ) ;
#11479=CARTESIAN_POINT ( 'NONE',  ( -1.433413778493000112, -78.18772245792399644, -10.60928646434000200 ) ) ;
#11507=CARTESIAN_POINT ( 'NONE',  ( 11.16396169635999946, -78.72364211442699400, 4.832020119862000307 ) ) ;
#11511=CARTESIAN_POINT ( 'NONE',  ( 4.528616239255999432, -79.18563051119899399, -9.933126443765001312 ) ) ;
#11526=CARTESIAN_POINT ( 'NONE',  ( 9.160466309606078994, -76.05310292770596448, -6.106013103578413315 ) ) ;
#11527=CARTESIAN_POINT ( 'NONE',  ( -6.394497296648475881, -79.12919937753510169, -9.959691579247014204 ) ) ;
#11541=CARTESIAN_POINT ( 'NONE',  ( 10.32668202803999868, -76.46150529199699974, -6.991146065296999446 ) ) ;
#11542=CARTESIAN_POINT ( 'NONE',  ( 4.892781134374668106, -78.76262618940380378, -9.574018988073637715 ) ) ;
#11544=ADVANCED_FACE ( 'NONE', ( #29964 ), #3981, .F. ) ;
#11549=CARTESIAN_POINT ( 'NONE',  ( -10.75000000000000000, -79.59999999999999432, 0.000000000000000000 ) ) ;
#11552=CARTESIAN_POINT ( 'NONE',  ( 2.179295889402999897, -78.69333441819799191, 11.00312592022000047 ) ) ;
#11555=ORIENTED_EDGE ( 'NONE', *, *, #10939, .F. ) ;
#11560=CARTESIAN_POINT ( 'NONE',  ( -8.650006198296225080, -77.90482871549633614, -7.141358535548220310 ) ) ;
#11574=CARTESIAN_POINT ( 'NONE',  ( -11.06076315227999984, -78.03473190728298903, 4.601693484369000053 ) ) ;
#11577=CARTESIAN_POINT ( 'NONE',  ( 10.20083256551678019, -78.87618565247994695, 3.463754871957966941 ) ) ;
#11582=CARTESIAN_POINT ( 'NONE',  ( 10.17013595917000046, -78.17720206157000007, -4.274350120612000481 ) ) ;
#11593=CARTESIAN_POINT ( 'NONE',  ( -8.729704736441000534, -77.71208082270700856, 7.043462628994999974 ) ) ;
#11605=CARTESIAN_POINT ( 'NONE',  ( 2.273403379124000026E-14, -92.33215535459000023, 0.000000000000000000 ) ) ;
#11622=CARTESIAN_POINT ( 'NONE',  ( 3.906270390259000358, -78.22752942077299565, -10.19392449069000151 ) ) ;
#11635=DIRECTION ( 'NONE',  ( -1.000000000000000000, 0.000000000000000000, 0.000000000000000000 ) ) ;
#11639=CARTESIAN_POINT ( 'NONE',  ( 2.813789756862274505, -76.64583333333334281, -10.47020627418438821 ) ) ;
#11646=CARTESIAN_POINT ( 'NONE',  ( 6.917788961650999546, -78.87567121485298571, -9.780606322222999083 ) ) ;
#11662=CARTESIAN_POINT ( 'NONE',  ( 1.407118610985540252, -76.96474581824523398, 10.75041648542711314 ) ) ;
#11665=VECTOR ( 'NONE', #48965, 1000.000000000000000 ) ;
#11671=CARTESIAN_POINT ( 'NONE',  ( 11.12972475151000040, -77.95443840457200224, -0.6195381557079999713 ) ) ;
#11680=CARTESIAN_POINT ( 'NONE',  ( 8.962230876647016231, -80.15077933492216289, 6.668113489195105714 ) ) ;
#11681=CARTESIAN_POINT ( 'NONE',  ( 9.785129497364000173, -79.19891811065798493, -6.997026981537000090 ) ) ;
#11683=CARTESIAN_POINT ( 'NONE',  ( -11.25198206936999945, -79.82677595101669965, -0.4763024974861999605 ) ) ;
#11690=ORIENTED_EDGE ( 'NONE', *, *, #41232, .F. ) ;
#11694=ORIENTED_EDGE ( 'NONE', *, *, #9288, .F. ) ;
#11701=CARTESIAN_POINT ( 'NONE',  ( 0.000000000000000000, -87.70000000000000284, 0.000000000000000000 ) ) ;
#11702=EDGE_CURVE ( 'NONE', #40725, #54085, #32903, .T. ) ;
#11704=CARTESIAN_POINT ( 'NONE',  ( -8.693530819781495111, -80.05018064888071194, 6.323148125732028113 ) ) ;
#11706=CARTESIAN_POINT ( 'NONE',  ( 10.02574878253000001, -76.68821439642898952, 4.955627619753999902 ) ) ;
#11708=EDGE_CURVE ( 'NONE', #32124, #33417, #27861, .T. ) ;
#11710=CARTESIAN_POINT ( 'NONE',  ( -10.60592548576000027, -76.86996292289100552, 2.886128316406999961 ) ) ;
#11716=CARTESIAN_POINT ( 'NONE',  ( -9.008069698304732142, -78.05420658299554759, 5.866654319817532937 ) ) ;
#11717=DIRECTION ( 'NONE',  ( 0.000000000000000000, 1.000000000000000000, 0.000000000000000000 ) ) ;
#11723=CARTESIAN_POINT ( 'NONE',  ( -4.882675258918448336, -79.20818948587456987, 11.01334000465016416 ) ) ;
#11740=CARTESIAN_POINT ( 'NONE',  ( -1.495312310314963478, -79.98653854018940024, 10.64535603553911614 ) ) ;
#11742=ORIENTED_EDGE ( 'NONE', *, *, #49273, .F. ) ;
#11743=CARTESIAN_POINT ( 'NONE',  ( 10.74995494553095021, -77.34974026310845829, -0.04523175681011006727 ) ) ;
#11767=EDGE_CURVE ( 'NONE', #19797, #9151, #7808, .T. ) ;
#11772=B_SPLINE_CURVE_WITH_KNOTS ( 'NONE', 3,
 ( #20794, #29924, #51820, #48538, #30216, #6930, #2510, #34356, #20514, #11374, #38511, #56527, #52104, #11662, #29638, #47691, #43241, #52393, #4829, #39663, #36114, #22236, #3937, #27533 ),
 .UNSPECIFIED., .F., .F.,
 ( 4, 2, 2, 2, 2, 2, 2, 2, 2, 2, 2, 4 ),
 ( 0.000000000000000000, 0.06249999999999995837, 0.1249999999999999167, 0.1874999999999999167, 0.2499999999999999445, 0.3749999999999999445, 0.5000000000000000000, 0.6250000000000000000, 0.7500000000000000000, 0.8750000000000000000, 0.9374999999999998890, 1.000000000000000000 ),
 .UNSPECIFIED. ) ;
#11788=CARTESIAN_POINT ( 'NONE',  ( 0.9776138843420000279, -78.07253854425700013, -12.12546088519999898 ) ) ;
#11790=CARTESIAN_POINT ( 'NONE',  ( 6.586108526242999694, -80.17391735373439587, 8.810401493720998900 ) ) ;
#11796=CARTESIAN_POINT ( 'NONE',  ( 5.817551787861000356, -79.78979933005598468, -10.15771087481999935 ) ) ;
#11804=CARTESIAN_POINT ( 'NONE',  ( -6.043427764450784778, -77.98333333333330586, -10.48543666025109822 ) ) ;
#11807=LINE ( 'NONE', #29781, #20133 ) ;
#11808=CARTESIAN_POINT ( 'NONE',  ( 3.005800864929102367, -78.90401322919130678, 11.38072746178960237 ) ) ;
#11822=CARTESIAN_POINT ( 'NONE',  ( 8.300816029147002340, -77.44509101131500017, -8.570629797104999170 ) ) ;
#11823=CARTESIAN_POINT ( 'NONE',  ( 0.06764921458087505557, -78.72558927515626692, -10.74974898025365988 ) ) ;
#11833=CARTESIAN_POINT ( 'NONE',  ( -0.2291600886666000092, -78.45728611218200399, -11.06898422383999936 ) ) ;
#11835=CARTESIAN_POINT ( 'NONE',  ( -11.05000000000000071, -81.00000000000000000, 0.000000000000000000 ) ) ;
#11850=EDGE_CURVE ( 'NONE', #39177, #22144, #44210, .T. ) ;
#11855=EDGE_CURVE ( 'NONE', #56550, #4324, #50072, .T. ) ;
#11862=CARTESIAN_POINT ( 'NONE',  ( -8.557169117579000783, -77.62779217592600389, -8.383968101560000719 ) ) ;
#11869=CARTESIAN_POINT ( 'NONE',  ( -10.26277353288999983, -78.05427472496999997, -3.721672393288999903 ) ) ;
#11870=CARTESIAN_POINT ( 'NONE',  ( 9.517603932039000014, -80.81724464549388642, 5.334679179331001109 ) ) ;
#11874=CARTESIAN_POINT ( 'NONE',  ( 1.341570204796000088, -79.46030790634399921, -12.19772931051000064 ) ) ;
#11876=CARTESIAN_POINT ( 'NONE',  ( 9.070694317316998934, -78.13394183500699341, 6.598531290616000078 ) ) ;
#11881=CARTESIAN_POINT ( 'NONE',  ( -7.624585833192999651, -77.14761986081299483, -9.463128976555999827 ) ) ;
#11885=CARTESIAN_POINT ( 'NONE',  ( -6.167563198928999846, -79.63052105083700383, 9.285244464097999639 ) ) ;
#11903=CARTESIAN_POINT ( 'NONE',  ( -5.029463238270672321, -80.99999999999998579, -9.703467947973461349 ) ) ;
#11904=CARTESIAN_POINT ( 'NONE',  ( -9.269928330473998557, -77.02913032869298604, 5.765743207788000646 ) ) ;
#11928=CARTESIAN_POINT ( 'NONE',  ( -11.06076315227999984, -78.17030901383499497, 4.601693484369000053 ) ) ;
#11935=CARTESIAN_POINT ( 'NONE',  ( 8.229676506584999274, -77.63320278771699634, 7.688067972860000765 ) ) ;
#11937=DIRECTION ( 'NONE',  ( 0.000000000000000000, 1.000000000000000000, 0.000000000000000000 ) ) ;
#11940=CARTESIAN_POINT ( 'NONE',  ( 6.436424241555000592, -80.32391735373440156, 8.610165096135999008 ) ) ;
#11954=CARTESIAN_POINT ( 'NONE',  ( -6.841895596235000099, -78.28127452059300140, -8.800175226803998996 ) ) ;
#11961=CARTESIAN_POINT ( 'NONE',  ( 6.867301783449541119, -80.28033772753711617, -8.270490925764946155 ) ) ;
#11964=CARTESIAN_POINT ( 'NONE',  ( 10.63577493293750464, -80.12563822179964745, 3.563963872659641652 ) ) ;
#11966=CARTESIAN_POINT ( 'NONE',  ( 10.52307592342000042, -79.35635755647699341, 5.828552047478999576 ) ) ;
#11968=CARTESIAN_POINT ( 'NONE',  ( 10.67847671903000162, -80.09913938103490239, 3.578272902691999491 ) ) ;
#11975=FACE_OUTER_BOUND ( 'NONE', #104, .T. ) ;
#11989=CARTESIAN_POINT ( 'NONE',  ( -10.51332871484163789, -80.08341230348659678, 2.247839838564814396 ) ) ;
#11992=CARTESIAN_POINT ( 'NONE',  ( -10.85772169724999969, -76.88886993234198997, 1.763485056683000041 ) ) ;
#11995=CARTESIAN_POINT ( 'NONE',  ( -10.79004770952999870, -76.87832357022099927, 1.752493610282999992 ) ) ;
#11996=EDGE_CURVE ( 'NONE', #41515, #18786, #2480, .T. ) ;
#12001=CARTESIAN_POINT ( 'NONE',  ( -4.122653348105549398, -78.00633941627575041, 9.928033855777968597 ) ) ;
#12002=CARTESIAN_POINT ( 'NONE',  ( 0.000000000000000000, -87.20000000000000284, 0.000000000000000000 ) ) ;
#12007=CARTESIAN_POINT ( 'NONE',  ( 5.462882135474436573, -79.13756601347041908, 10.73736906863111251 ) ) ;
#12024=CARTESIAN_POINT ( 'NONE',  ( 4.982545483063324454, -79.93680840925433984, 9.528384401333727993 ) ) ;
#12031=ORIENTED_EDGE ( 'NONE', *, *, #24078, .T. ) ;
#12037=CARTESIAN_POINT ( 'NONE',  ( 9.846943056836000352, -78.89225416815600056, -6.945033154232000072 ) ) ;
#12062=CARTESIAN_POINT ( 'NONE',  ( 8.174587033571999228, -77.18454464919399527, -8.440297792765999674 ) ) ;
#12068=FACE_OUTER_BOUND ( 'NONE', #8123, .T. ) ;
#12071=CARTESIAN_POINT ( 'NONE',  ( 0.4872551020249000220, -77.38064477680499920, 12.03986520427999984 ) ) ;
#12077=DIRECTION ( 'NONE',  ( 0.000000000000000000, -1.000000000000000000, 0.000000000000000000 ) ) ;
#12080=CARTESIAN_POINT ( 'NONE',  ( 8.185807787635999588, -79.00525020734799853, 8.524724615276998207 ) ) ;
#12082=CARTESIAN_POINT ( 'NONE',  ( 5.462937134022767260, -79.73749999999996874, 10.72588375220489887 ) ) ;
#12089=LINE ( 'NONE', #50745, #42766 ) ;
#12090=CARTESIAN_POINT ( 'NONE',  ( -9.991034349598352904, -79.00462831674920494, 6.345779858256005213 ) ) ;
#12097=DIRECTION ( 'NONE',  ( 0.000000000000000000, -1.000000000000000000, -1.983598470663000190E-13 ) ) ;
#12105=CARTESIAN_POINT ( 'NONE',  ( -12.47961470992000166, -76.81611152454399871, 1.652929733484999941 ) ) ;
#12106=CARTESIAN_POINT ( 'NONE',  ( 0.3551920607923636508, -78.72769057884195831, -10.74440567796370694 ) ) ;
#12116=CARTESIAN_POINT ( 'NONE',  ( 8.645668071321999548, -78.70665028547099951, 7.146365085715999044 ) ) ;
#12124=CARTESIAN_POINT ( 'NONE',  ( 11.01657791821742371, -77.11497476844333221, 2.111070802985992589 ) ) ;
#12134=CARTESIAN_POINT ( 'NONE',  ( 2.121761250100177243, -79.78927564072810696, -11.65386660924905549 ) ) ;
#12135=CARTESIAN_POINT ( 'NONE',  ( 0.000000000000000000, -87.20000000000000284, 0.000000000000000000 ) ) ;
#12140=CARTESIAN_POINT ( 'NONE',  ( 10.74972511287136534, -79.34491661344335967, -0.7035994354972746612 ) ) ;
#12141=CARTESIAN_POINT ( 'NONE',  ( -1.835125225091999823, -77.95334396101199559, 11.83842809849000055 ) ) ;
#12158=CARTESIAN_POINT ( 'NONE',  ( 10.75916580684000046, -78.10670549200499124, 3.171507801093999657 ) ) ;
#12162=CARTESIAN_POINT ( 'NONE',  ( -1.144883253578000248, -76.82350204046299780, 12.33394807668000048 ) ) ;
#12166=CARTESIAN_POINT ( 'NONE',  ( 10.42771306556999988, -79.93012082385709505, -3.939212573787000515 ) ) ;
#12188=B_SPLINE_CURVE_WITH_KNOTS ( 'NONE', 3,
 ( #11270, #47298, #7120, #24255, #20126, #42271, #1838, #6825, #52286, #19832, #20982, #24835, #47006, #51719, #33391, #56996, #43423, #2410, #38405, #55847, #37826, #42851, #52005, #11560, #29537, #47593, #15397, #38115, #38696, #38985, #51137, #29824, #25120, #43143, #10690, #2702, #51428, #10984, #28669, #7404, #56716, #6534, #15685, #46721, #24545, #16274, #2126, #34252, #56137, #33681, #47874, #25407, #12124, #17128, #50119, #36517, #54250, #12412, #12694, #548, #40664, #7692, #21267, #44283, #35112 ),
 .UNSPECIFIED., .F., .F.,
 ( 4, 1, 1, 1, 1, 1, 1, 1, 1, 1, 1, 1, 1, 1, 1, 1, 1, 1, 1, 1, 1, 1, 1, 1, 1, 1, 1, 1, 1, 1, 1, 1, 1, 1, 1, 1, 1, 1, 1, 1, 1, 1, 1, 1, 1, 1, 1, 1, 1, 1, 1, 1, 1, 1, 1, 1, 1, 1, 1, 1, 1, 1, 4 ),
 ( 0.000000000000000000, 0.01249977918653473984, 0.02874978664248292043, 0.04499979409843109929, 0.06124980155437927815, 0.07749980901032745007, 0.09374981646627562892, 0.1099998239222238078, 0.1262498313781720005, 0.1424998388341201516, 0.1587498462900683582, 0.1749998537460165093, 0.1912498612019647160, 0.2074998686579128671, 0.2237498761138610737, 0.2399998835698092525, 0.2562498910257574036, 0.2724998984817056380, 0.2887499059376538169, 0.3049999133936019402, 0.3212499208495501191, 0.3374999283054983534, 0.3537499357614465323, 0.3699999432173946556, 0.3862499506733428345, 0.4024999581292910689, 0.4187499655852392477, 0.4349999730411874266, 0.4512499804971355499, 0.4674999879530837843, 0.4837499954090319632, 0.5000000028649801420, 0.5162500103209283209, 0.5325000177768764997, 0.5487500252328246786, 0.5650000326887728574, 0.5812500401447211473, 0.5975000476006693262, 0.6137500550566175050, 0.6300000625125655729, 0.6462500699685137517, 0.6625000774244619306, 0.6787500848804101095, 0.6950000923363582883, 0.7112500997923065782, 0.7275001072482547571, 0.7437501147042029359, 0.7600001221601511148, 0.7762501296160991826, 0.7925001370720473615, 0.8087501445279955403, 0.8250001519839437192, 0.8412501594398920091, 0.8575001668958401879, 0.8737501743517883668, 0.8900001818077365456, 0.9062501892636847245, 0.9225001967196327923, 0.9387502041755809712, 0.9550002116315291500, 0.9712502190874773289, 0.9875002265434256188, 1.000000000000000000 ),
 .UNSPECIFIED. ) ;
#12191=CARTESIAN_POINT ( 'NONE',  ( -9.786314039287999478, -78.03687501975998941, 4.837708502169000724 ) ) ;
#12196=ORIENTED_EDGE ( 'NONE', *, *, #25391, .F. ) ;
#12210=CARTESIAN_POINT ( 'NONE',  ( 11.36821324764999908, -77.92614517502100568, -3.778861202892000115 ) ) ;
#12217=CARTESIAN_POINT ( 'NONE',  ( 6.163257195008000622, -78.56341404718699550, -9.114053931137998887 ) ) ;
#12219=CARTESIAN_POINT ( 'NONE',  ( -6.603701251060000388, -80.74830188227322481, 9.115088936944999887 ) ) ;
#12220=ORIENTED_EDGE ( 'NONE', *, *, #27751, .T. ) ;
#12237=CARTESIAN_POINT ( 'NONE',  ( -10.86494198988000015, -78.22680183458999181, -2.491513063939999828 ) ) ;
#12243=CARTESIAN_POINT ( 'NONE',  ( -4.098243062044448770, -80.19425443582535706, -9.937901660273714910 ) ) ;
#12246=CARTESIAN_POINT ( 'NONE',  ( 7.313768098873999257, -78.88818067319900251, 9.313141831727000053 ) ) ;
#12249=CARTESIAN_POINT ( 'NONE',  ( -10.80063122475000092, -78.84626760295098791, -3.190662894339999944 ) ) ;
#12269=CARTESIAN_POINT ( 'NONE',  ( -9.936142110726182253, -80.06889634899292219, 4.117545299896771205 ) ) ;
#12272=CARTESIAN_POINT ( 'NONE',  ( 1.546553306619000256, -76.46993419121800173, -11.07619323537999989 ) ) ;
#12275=CARTESIAN_POINT ( 'NONE',  ( 10.06256222744999995, -76.17602919452599508, 4.718524714222000149 ) ) ;
#12281=EDGE_CURVE ( 'NONE', #53816, #41078, #41584, .T. ) ;
#12283=CARTESIAN_POINT ( 'NONE',  ( -0.8442961504774461057, -80.98138397070125905, 10.71670580309706544 ) ) ;
#12288=CARTESIAN_POINT ( 'NONE',  ( -11.29698467241381543, -79.27175061103834253, 4.184771565250528624 ) ) ;
#12293=B_SPLINE_CURVE_WITH_KNOTS ( 'NONE', 3,
 ( #41889, #55468, #55175, #2333, #47218, #55769, #6747, #19166, #1467, #24756, #51057, #42772, #10021, #38324, #7320, #34747, #25323, #43631, #51924, #21183, #48644, #52775, #56344 ),
 .UNSPECIFIED., .F., .F.,
 ( 4, 2, 2, 2, 2, 2, 1, 2, 2, 2, 2, 4 ),
 ( 0.000000000000000000, 0.1250000000000000555, 0.2500000000000000555, 0.3125000000000000000, 0.3749999999999999445, 0.4374999999999998890, 0.4999999999999998890, 0.5624999999999998890, 0.6249999999999998890, 0.7499999999999998890, 0.8749999999999998890, 1.000000000000000000 ),
 .UNSPECIFIED. ) ;
#12297=ORIENTED_EDGE ( 'NONE', *, *, #22440, .F. ) ;
#12306=CARTESIAN_POINT ( 'NONE',  ( 4.250518816003403089, -79.94278005840584456, 9.873894375703258675 ) ) ;
#12311=VECTOR ( 'NONE', #7652, 1000.000000000000000 ) ;
#12317=EDGE_CURVE ( 'NONE', #35080, #38899, #33312, .T. ) ;
#12322=B_SPLINE_CURVE_WITH_KNOTS ( 'NONE', 3,
 ( #15542, #43288, #2841, #11134, #50989, #42706, #6096, #42421, #24106, #20558, #10540, #37971, #28523, #34107, #1691, #47447, #24406, #1990, #19984, #55996, #47157, #2273, #6687 ),
 .UNSPECIFIED., .F., .F.,
 ( 4, 2, 2, 2, 2, 1, 2, 2, 2, 2, 2, 4 ),
 ( 0.000000000000000000, 0.1249999999999998890, 0.2499999999999997780, 0.3749999999999997224, 0.4374999999999997224, 0.4999999999999996669, 0.5624999999999996669, 0.6249999999999997780, 0.7499999999999998890, 0.8749999999999998890, 0.9374999999999998890, 1.000000000000000000 ),
 .UNSPECIFIED. ) ;
#12328=AXIS2_PLACEMENT_3D ( 'NONE', #24426, #20288, #38576 ) ;
#12329=VERTEX_POINT ( 'NONE', #610 ) ;
#12335=CARTESIAN_POINT ( 'NONE',  ( 4.767018142753490118, -80.18960264150359762, 10.03241642955576829 ) ) ;
#12336=CARTESIAN_POINT ( 'NONE',  ( -4.085659785884999451, -78.55269560739655788, 11.26159174134999930 ) ) ;
#12352=CARTESIAN_POINT ( 'NONE',  ( -10.75000000000000000, -80.50000000000000000, -1.711887504597999906E-14 ) ) ;
#12354=CARTESIAN_POINT ( 'NONE',  ( 8.480197680338001476, -78.05907011069199086, -8.881555409017000358 ) ) ;
#12356=CARTESIAN_POINT ( 'NONE',  ( 6.585791278903703194, -80.10725068706773300, 8.809977328666299456 ) ) ;
#12359=CARTESIAN_POINT ( 'NONE',  ( -6.210567785792292739, -79.52403206663427682, 8.774603838976910097 ) ) ;
#12362=CARTESIAN_POINT ( 'NONE',  ( 10.28508546004999857, -79.48465556260299536, 6.261730588902000072 ) ) ;
#12367=CARTESIAN_POINT ( 'NONE',  ( -2.811854283077139804, -79.79375000000001705, 11.70391985135060864 ) ) ;
#12391=CARTESIAN_POINT ( 'NONE',  ( -11.67502321291000023, -76.85709426284898882, -4.708162379318000745 ) ) ;
#12392=CARTESIAN_POINT ( 'NONE',  ( -9.600681700141771913, -78.63729878341381152, -4.836084120192285063 ) ) ;
#12394=VERTEX_POINT ( 'NONE', #41018 ) ;
#12400=CARTESIAN_POINT ( 'NONE',  ( 0.1392748842281999744, -77.12401228047586699, 11.21600254538999941 ) ) ;
#12403=CARTESIAN_POINT ( 'NONE',  ( -8.982117338527000783, -79.85057669154679161, 6.718606902359000266 ) ) ;
#12407=EDGE_LOOP ( 'NONE', ( #25503, #56189, #1674, #55264 ) ) ;
#12412=CARTESIAN_POINT ( 'NONE',  ( 0.5473746484684922642, -76.97879305343433032, -11.20365965675252795 ) ) ;
#12420=ADVANCED_FACE ( 'NONE', ( #39992 ), #50845, .F. ) ;
#12425=ORIENTED_EDGE ( 'NONE', *, *, #54062, .F. ) ;
#12429=CARTESIAN_POINT ( 'NONE',  ( -11.86109855473999986, -78.50952966248199516, -1.682380905046999997 ) ) ;
#12442=FACE_OUTER_BOUND ( 'NONE', #10902, .T. ) ;
#12445=CARTESIAN_POINT ( 'NONE',  ( 10.30382210470000182, -76.14431275097399521, -6.875193506978999558 ) ) ;
#12449=CARTESIAN_POINT ( 'NONE',  ( 10.83083824887000013, -79.43986664982399759, -2.635819302916999618 ) ) ;
#12456=FACE_OUTER_BOUND ( 'NONE', #48156, .T. ) ;
#12468=CARTESIAN_POINT ( 'NONE',  ( -0.8033103333046999195, -77.19254838670400432, -10.88715107357000100 ) ) ;
#12474=CARTESIAN_POINT ( 'NONE',  ( 8.554126827399000987, -79.96012667201070201, -7.255689219360999864 ) ) ;
#12492=CARTESIAN_POINT ( 'NONE',  ( -5.528827828690000779, -79.16377338295399113, -10.74483463111999981 ) ) ;
#12494=CARTESIAN_POINT ( 'NONE',  ( -10.26943924278000075, -78.65863669146300197, 6.168847710360999770 ) ) ;
#12501=CARTESIAN_POINT ( 'NONE',  ( -8.764875654205999567, -77.76938450272599823, 7.071839882566000490 ) ) ;
#12502=CARTESIAN_POINT ( 'NONE',  ( 0.6457562008196999770, -80.45297733623330316, -11.23729128717999970 ) ) ;
#12504=CARTESIAN_POINT ( 'NONE',  ( 9.238576773750208915, -80.29311845634506994, 5.559101997765116820 ) ) ;
#12510=CARTESIAN_POINT ( 'NONE',  ( -4.647088938219000376, -78.10731010046200140, 10.20895072913000057 ) ) ;
#12521=CARTESIAN_POINT ( 'NONE',  ( -10.68734765800000019, -76.66107590507699854, -2.735374635455000369 ) ) ;
#12526=CARTESIAN_POINT ( 'NONE',  ( -5.827680902778979544, -80.17946448389406555, -9.033442447713206036 ) ) ;
#12527=CARTESIAN_POINT ( 'NONE',  ( -11.75935053634283989, -76.25833333328885999, 2.506420011343689414 ) ) ;
#12528=CARTESIAN_POINT ( 'NONE',  ( 11.21501439771859054, -80.09840187879784423, -0.2123206566945571028 ) ) ;
#12531=CARTESIAN_POINT ( 'NONE',  ( -9.625846388754000671, -79.11728850969700488, -7.214584339064000318 ) ) ;
#12533=CARTESIAN_POINT ( 'NONE',  ( -0.2732061834123999944, -79.20034006197499821, 11.25874428786999992 ) ) ;
#12534=CARTESIAN_POINT ( 'NONE',  ( -10.75000000000000000, -77.60000000000000853, 2.252154972635999871E-14 ) ) ;
#12542=CARTESIAN_POINT ( 'NONE',  ( 9.125560752801000319, -79.27717617799699212, -5.991619725684000031 ) ) ;
#12548=ORIENTED_EDGE ( 'NONE', *, *, #14195, .T. ) ;
#12552=CARTESIAN_POINT ( 'NONE',  ( 5.392351874751835084, -79.79999999999999716, 10.61425309677364837 ) ) ;
#12553=CARTESIAN_POINT ( 'NONE',  ( -10.27037232371433895, -80.07614521482391012, 3.176628361632590991 ) ) ;
#12561=CARTESIAN_POINT ( 'NONE',  ( 7.781700644545999523, -76.83820410512299759, 7.610227757096000190 ) ) ;
#12583=CARTESIAN_POINT ( 'NONE',  ( -0.9849936891751999157, -80.86803245780032512, -11.22225356808999841 ) ) ;
#12589=CARTESIAN_POINT ( 'NONE',  ( 4.592783297679469356, -79.93999167834631692, 9.722085715425176744 ) ) ;
#12604=CARTESIAN_POINT ( 'NONE',  ( 0.3923696854197999961, -77.38648093799099570, -11.92498586577000097 ) ) ;
#12632=CARTESIAN_POINT ( 'NONE',  ( -12.00000000000000000, -77.79999999999999716, 0.000000000000000000 ) ) ;
#12641=CARTESIAN_POINT ( 'NONE',  ( -3.600395895414000069, -77.34004702781498963, 11.61979689923000159 ) ) ;
#12646=CARTESIAN_POINT ( 'NONE',  ( -8.988913058593215766, -79.55386370958336784, 5.895957875921411961 ) ) ;
#12648=CARTESIAN_POINT ( 'NONE',  ( -0.7446082967701634914, -78.77994009691290955, 12.02413132939186369 ) ) ;
#12649=CARTESIAN_POINT ( 'NONE',  ( -11.66126045851000015, -79.67109097853600019, 3.001209278140000158 ) ) ;
#12651=CARTESIAN_POINT ( 'NONE',  ( 10.26420232462597149, -79.69374999999999432, 6.287639862081866760 ) ) ;
#12657=EDGE_LOOP ( 'NONE', ( #21849, #57626 ) ) ;
#12674=VERTEX_POINT ( 'NONE', #19606 ) ;
#12676=CARTESIAN_POINT ( 'NONE',  ( 0.03300762091332999637, -76.13364338555700783, 11.93139356344000035 ) ) ;
#12684=CARTESIAN_POINT ( 'NONE',  ( -9.524774638983998898, -77.20572130948103506, 5.924253427061998423 ) ) ;
#12694=CARTESIAN_POINT ( 'NONE',  ( -3.244532303892139424, -76.95155671043232815, -10.73753325156647520 ) ) ;
#12699=FACE_OUTER_BOUND ( 'NONE', #15304, .T. ) ;
#12705=ADVANCED_FACE ( 'NONE', ( #6609, #37312 ), #11343, .F. ) ;
#12711=CARTESIAN_POINT ( 'NONE',  ( 6.035966914210000311, -77.89908533016399872, 10.34809972146999968 ) ) ;
#12714=CARTESIAN_POINT ( 'NONE',  ( 11.83900414546000057, -78.31650993477799716, -1.507807444711000144 ) ) ;
#12723=CARTESIAN_POINT ( 'NONE',  ( -11.88401260600999976, -79.80654510736209772, 3.058538056121000270 ) ) ;
#12728=CARTESIAN_POINT ( 'NONE',  ( -6.508777536021999488, -76.58936719843599406, -10.40112358611999888 ) ) ;
#12730=CARTESIAN_POINT ( 'NONE',  ( -7.391903123959864708, -76.93479338433584758, 7.904442030565260069 ) ) ;
#12732=CARTESIAN_POINT ( 'NONE',  ( 3.609690327934000020, -80.05722375786560008, 10.39335624559999971 ) ) ;
#12739=ADVANCED_FACE ( 'NONE', ( #1912 ), #29319, .T. ) ;
#12746=ORIENTED_EDGE ( 'NONE', *, *, #16607, .F. ) ;
#12754=CARTESIAN_POINT ( 'NONE',  ( -7.639223145873000220, -76.51163981165899486, 7.500260266847000423 ) ) ;
#12757=CARTESIAN_POINT ( 'NONE',  ( 5.865103843792000227, -78.36710291063299394, -9.561319920857000554 ) ) ;
#12774=CARTESIAN_POINT ( 'NONE',  ( -2.478361877531000346, -79.68515284566699108, -11.82696626457999933 ) ) ;
#12783=CARTESIAN_POINT ( 'NONE',  ( -11.00476719864000152, -77.30636667169498821, 2.393546210564999832 ) ) ;
#12785=CARTESIAN_POINT ( 'NONE',  ( -5.300832050426999231, -80.90938799829500283, -9.929493364645999520 ) ) ;
#12792=CARTESIAN_POINT ( 'NONE',  ( 2.854969924326999919, -78.05283741445799706, 10.84745395576000071 ) ) ;
#12797=VECTOR ( 'NONE', #14377, 1000.000000000000000 ) ;
#12800=DIRECTION ( 'NONE',  ( 0.000000000000000000, 1.000000000000000000, 0.000000000000000000 ) ) ;
#12802=CARTESIAN_POINT ( 'NONE',  ( -6.912545260079999920, -78.34900158500600753, -8.891046157644998615 ) ) ;
#12808=CARTESIAN_POINT ( 'NONE',  ( 3.232567627276669242, -80.24941509227865311, -10.25408852723510478 ) ) ;
#12816=CARTESIAN_POINT ( 'NONE',  ( 10.75000000000000000, -78.75000000000000000, 0.000000000000000000 ) ) ;
#12821=EDGE_LOOP ( 'NONE', ( #32412, #48577, #21332, #17018 ) ) ;
#12822=DIRECTION ( 'NONE',  ( 0.000000000000000000, -1.000000000000000000, 0.000000000000000000 ) ) ;
#12824=CARTESIAN_POINT ( 'NONE',  ( 10.84306248592000088, -78.81415834696599632, -1.266239280945999912 ) ) ;
#12834=CARTESIAN_POINT ( 'NONE',  ( 4.110498728239191379, -79.79999999999998295, 11.18969932762453112 ) ) ;
#12838=CARTESIAN_POINT ( 'NONE',  ( 7.486068761172999686, -76.08624778869000238, -8.059700645992000645 ) ) ;
#12842=CARTESIAN_POINT ( 'NONE',  ( -7.489130957889000406, -76.46197497528599740, 7.898313055298999963 ) ) ;
#12845=DIRECTION ( 'NONE',  ( -1.000000000000000000, 0.000000000000000000, 0.000000000000000000 ) ) ;
#12869=CARTESIAN_POINT ( 'NONE',  ( -3.342781753851123305, -80.00035736669231312, 10.21718976228000031 ) ) ;
#12873=CARTESIAN_POINT ( 'NONE',  ( -4.661427456832804239, -77.18932811019587348, -9.686758570029148530 ) ) ;
#12876=VERTEX_POINT ( 'NONE', #18240 ) ;
#12891=ORIENTED_EDGE ( 'NONE', *, *, #50634, .T. ) ;
#12900=CARTESIAN_POINT ( 'NONE',  ( -9.149885487026406139, -80.39887705342988511, -6.477978945181864567 ) ) ;
#12908=DIRECTION ( 'NONE',  ( -0.7071067811864976127, -0.7071067811865975328, 4.006692910709986783E-09 ) ) ;
#12912=AXIS2_PLACEMENT_3D ( 'NONE', #16569, #31495, #34554 ) ;
#12914=B_SPLINE_CURVE_WITH_KNOTS ( 'NONE', 3,
 ( #3773, #35638, #39781, #562, #8205, #45413, #13505, #31797, #27077, #4956, #26208, #44511, #44812, #36531, #53364, #22961 ),
 .UNSPECIFIED., .F., .F.,
 ( 4, 2, 2, 2, 2, 2, 2, 4 ),
 ( 0.000000000000000000, 0.1250000000000000278, 0.2500000000000000555, 0.3750000000000001110, 0.5000000000000001110, 0.7500000000000002220, 0.8750000000000002220, 1.000000000000000000 ),
 .UNSPECIFIED. ) ;
#12920=CARTESIAN_POINT ( 'NONE',  ( -5.597547907814000467, -78.10874741097399010, -9.372450235129999641 ) ) ;
#12921=CARTESIAN_POINT ( 'NONE',  ( -8.353021825866999706, -78.43888052662398991, -9.001266886329000627 ) ) ;
#12925=CARTESIAN_POINT ( 'NONE',  ( -3.691465036726909066, -79.50301741532913979, 10.09624330836405015 ) ) ;
#12928=CARTESIAN_POINT ( 'NONE',  ( 10.90780079584000006, -79.47248173447398756, -5.366096107902000867 ) ) ;
#12929=CARTESIAN_POINT ( 'NONE',  ( -2.510982762904000243, -80.68017688227318729, -10.76696539026999844 ) ) ;
#12956=CARTESIAN_POINT ( 'NONE',  ( -3.152476705098000487, -77.22767140587998824, -11.82163513714000125 ) ) ;
#12964=CARTESIAN_POINT ( 'NONE',  ( 8.196653188619999142, -77.55979376850486062, 7.657217973713000170 ) ) ;
#12966=CARTESIAN_POINT ( 'NONE',  ( 10.89876807034000095, -79.63268594753199636, -2.652350870517000025 ) ) ;
#12970=ORIENTED_EDGE ( 'NONE', *, *, #48133, .F. ) ;
#12984=CARTESIAN_POINT ( 'NONE',  ( 1.099819419251000019, -79.61718521679551941, 11.16281809564999961 ) ) ;
#12985=B_SPLINE_SURFACE_WITH_KNOTS ( 'NONE', 3, 3, ( 
 ( #58172, #57879, #26566, #8873, #17738, #44598, #27155, #40753, #4447, #22448, #18326, #40463, #8287, #39582, #49920, #35726, #13882, #26867, #36319, #31284, #45195, #54342, #21578, #31876, #12714, #44303, #53753, #13290, #49327, #26290, #44895, #4152, #22151, #55, #3859, #49031, #21857, #39866, #40159, #25998, #17436, #44021, #18030, #35421, #36022, #53451, #3573, #8579, #37189, #55203, #32166, #36610, #41626, #14462, #36897, #10052, #27450, #54910, #23903, #32453, #32745, #41049, #10339, #37775, #50793, #41338, #37476 ),
 ( #45488, #42219, #46370, #46662, #19780, #19198, #6189, #55796, #41921, #1784, #55497, #924, #14746, #15346, #5323, #24202, #1493, #28034, #54633, #28317, #23330, #15047, #18904, #50498, #33340, #1206, #9465, #637, #5894, #50205, #51085, #19483, #5031, #33039, #46078, #10635, #45787, #28617, #23033, #18619, #5602, #23613, #14169, #9755, #27740, #20925, #47243, #46955, #48104, #39214, #29198, #38926, #33912, #38352, #25636, #28911, #12071, #20075, #2077, #7065, #51671, #52515, #47819, #7636, #6481, #42506, #43090 ),
 ( #24493, #57228, #29482, #6774, #11507, #11218, #16793, #3220, #20641, #38643, #15633, #38066, #25066, #56374, #20357, #51951, #10930, #15924, #7350, #47541, #16216, #56087, #52231, #21207, #34194, #24783, #56943, #51373, #11788, #29763, #43661, #16502, #33629, #42798, #2648, #2359, #56661, #25349, #43366, #2924, #34485, #30052, #43947, #4373, #30342, #17361, #9097, #53974, #13212, #30634, #30918, #22374, #44229, #22675, #35347, #12641, #3497, #40386, #53372, #48667, #45125, #26790, #13513, #39788, #53088, #58393, #17956 ),
 ( #58096, #17072, #52801, #31207, #17658, #7923, #35947, #49247, #8211, #44818, #3781, #31506, #12921, #21783, #8797, #57801, #35645, #25923, #53672, #4676, #49552, #26213, #27086, #40686, #278, #34775, #12354, #48385, #21500, #57511, #48954, #39506, #35054, #8498, #26494, #22071, #44517, #4069, #40080, #46303, #13805, #852, #51016, #37409, #55131, #14104, #14388, #5826, #27671, #6123, #18836, #54564, #45419, #23833, #36829, #32100, #28549, #10268, #55429, #23259, #36541, #41850, #1429, #45717, #10566, #569, #41556 ) ),
 .UNSPECIFIED., .F., .F., .F.,
 ( 4, 4 ),
 ( 4, 1, 1, 1, 1, 1, 1, 1, 1, 1, 1, 1, 1, 1, 1, 1, 1, 1, 1, 1, 1, 1, 1, 1, 1, 1, 1, 1, 1, 1, 1, 1, 1, 1, 1, 1, 1, 1, 1, 1, 1, 1, 1, 1, 1, 1, 1, 1, 1, 1, 1, 1, 1, 1, 1, 1, 1, 1, 1, 1, 1, 1, 1, 1, 4 ),
 ( -0.1772706441294000235, 1.177270644128999955 ),
 ( -0.02000000000000000042, -0.003749999999999999861, 0.01250000000000000069, 0.02875000000000000125, 0.04499999999999999833, 0.06124999999999999889, 0.07749999999999999944, 0.09375000000000000000, 0.1100000000000000006, 0.1262500000000000011, 0.1424999999999999878, 0.1587500000000000022, 0.1749999999999999889, 0.1912500000000000033, 0.2074999999999999900, 0.2237500000000000044, 0.2399999999999999911, 0.2562499999999999778, 0.2725000000000000200, 0.2887500000000000067, 0.3049999999999999933, 0.3212499999999999800, 0.3375000000000000222, 0.3537500000000000089, 0.3699999999999999956, 0.3862499999999999822, 0.4025000000000000244, 0.4187500000000000111, 0.4349999999999999978, 0.4512499999999999845, 0.4675000000000000266, 0.4837500000000000133, 0.5000000000000000000, 0.5162499999999999867, 0.5324999999999999734, 0.5487499999999999600, 0.5649999999999999467, 0.5812500000000000444, 0.5975000000000000311, 0.6137500000000000178, 0.6300000000000000044, 0.6462499999999999911, 0.6624999999999999778, 0.6787499999999999645, 0.6949999999999999512, 0.7112500000000000488, 0.7275000000000000355, 0.7437500000000000222, 0.7600000000000000089, 0.7762499999999999956, 0.7924999999999999822, 0.8087499999999999689, 0.8249999999999999556, 0.8412500000000000533, 0.8575000000000000400, 0.8737500000000000266, 0.8900000000000000133, 0.9062500000000000000, 0.9224999999999999867, 0.9387499999999999734, 0.9549999999999999600, 0.9712499999999999467, 0.9875000000000000444, 1.003749999999999920, 1.020000000000000018 ),
 .UNSPECIFIED. ) ;
#12992=CYLINDRICAL_SURFACE ( 'NONE', #7889, 12.00000000000000000 ) ;
#12993=DIRECTION ( 'NONE',  ( -0.3090169943748910519, 0.000000000000000000, 0.9510565162951719609 ) ) ;
#12996=CARTESIAN_POINT ( 'NONE',  ( -11.99938675919335651, -76.39122388691224330, 1.256423165442345447 ) ) ;
#13005=CARTESIAN_POINT ( 'NONE',  ( 6.329984427697000093, -78.16117817800899559, 9.260097609460000712 ) ) ;
#13008=CARTESIAN_POINT ( 'NONE',  ( -12.06623464587999983, -76.02337612386199339, -2.225025071791999931 ) ) ;
#13013=CARTESIAN_POINT ( 'NONE',  ( 10.75129243007999946, -78.90912175438100462, 2.472133787718999720 ) ) ;
#13025=CARTESIAN_POINT ( 'NONE',  ( 9.393203674808260573, -78.29166666666665719, 5.413904038987188194 ) ) ;
#13036=CARTESIAN_POINT ( 'NONE',  ( -10.57583826563999985, -76.59334884066400662, -2.706834349011999930 ) ) ;
#13040=CARTESIAN_POINT ( 'NONE',  ( 10.63562707217000103, -80.04183570101619694, 3.563914325689000240 ) ) ;
#13057=CARTESIAN_POINT ( 'NONE',  ( -9.793435742113999254, -78.88928473073799807, 7.469585195921999876 ) ) ;
#13059=CARTESIAN_POINT ( 'NONE',  ( -2.170310836754803852, -77.99131390061577918, 10.52858361609908577 ) ) ;
#13060=CARTESIAN_POINT ( 'NONE',  ( 0.3864029911681999829, -77.32930023569899447, -11.74364478040999948 ) ) ;
#13068=CARTESIAN_POINT ( 'NONE',  ( 8.315675604772998497, -78.01451158974199984, -7.594965687514999786 ) ) ;
#13070=CARTESIAN_POINT ( 'NONE',  ( 1.957338178487000313, -80.18450047619698751, 11.08434491862000115 ) ) ;
#13087=CARTESIAN_POINT ( 'NONE',  ( -2.194598275924000141, -77.88598375397499751, -11.04616236372000060 ) ) ;
#13093=CARTESIAN_POINT ( 'NONE',  ( -5.052420809101000088E-14, -80.84999999994215614, 0.000000000000000000 ) ) ;
#13094=CARTESIAN_POINT ( 'NONE',  ( 2.155490813879537448, -80.24142094974830286, -10.53147914176322075 ) ) ;
#13100=CARTESIAN_POINT ( 'NONE',  ( -10.99597256337999873, -79.40424884139699202, -1.828438666275999935 ) ) ;
#13106=EDGE_CURVE ( 'NONE', #15092, #32066, #14070, .T. ) ;
#13110=CARTESIAN_POINT ( 'NONE',  ( 0.000000000000000000, -75.15999999999999659, 0.000000000000000000 ) ) ;
#13111=CARTESIAN_POINT ( 'NONE',  ( -8.833962032441000645, -79.59003032942598566, 6.607787011616999884 ) ) ;
#13112=CARTESIAN_POINT ( 'NONE',  ( -12.00000000000000178, -76.31041666661776901, -1.570796326794897890 ) ) ;
#13119=ORIENTED_EDGE ( 'NONE', *, *, #57844, .T. ) ;
#13126=CARTESIAN_POINT ( 'NONE',  ( 9.776276929627000456, -76.11132973067898888, -5.431214116490000521 ) ) ;
#13136=ADVANCED_FACE ( 'NONE', ( #11975 ), #47715, .F. ) ;
#13138=DIRECTION ( 'NONE',  ( 0.000000000000000000, -1.000000000000000000, 0.000000000000000000 ) ) ;
#13162=CARTESIAN_POINT ( 'NONE',  ( -4.665370423308930370, -77.18929613357201447, -9.684859775919129277 ) ) ;
#13166=VERTEX_POINT ( 'NONE', #3402 ) ;
#13172=CARTESIAN_POINT ( 'NONE',  ( 5.516244905679999810, -78.96017368086199895, 10.58329673088999989 ) ) ;
#13173=AXIS2_PLACEMENT_3D ( 'NONE', #20172, #10738, #28125 ) ;
#13180=CARTESIAN_POINT ( 'NONE',  ( -10.48543666025111420, -78.75833333333331154, 6.043427764450754580 ) ) ;
#13189=DIRECTION ( 'NONE',  ( 0.000000000000000000, -1.000000000000000000, 0.000000000000000000 ) ) ;
#13191=ADVANCED_FACE ( 'NONE', ( #39119 ), #34961, .F. ) ;
#13210=CARTESIAN_POINT ( 'NONE',  ( -6.797161730763000342, -77.45507517892998806, 8.542479639784000156 ) ) ;
#13212=CARTESIAN_POINT ( 'NONE',  ( -5.342744711435999605, -77.52995223578199102, -10.92875150845999954 ) ) ;
#13221=CARTESIAN_POINT ( 'NONE',  ( -6.472232015619999501, -79.04405766632500274, 10.01728928138000008 ) ) ;
#13223=CARTESIAN_POINT ( 'NONE',  ( -10.11188841328999999, -80.54028613825869343, 4.470155568018000736 ) ) ;
#13226=CARTESIAN_POINT ( 'NONE',  ( 9.668944085725000193, -77.12619714393999004, 5.685915129398999568 ) ) ;
#13241=AXIS2_PLACEMENT_3D ( 'NONE', #38283, #48042, #29988 ) ;
#13242=DIRECTION ( 'NONE',  ( 0.000000000000000000, -1.000000000000000000, 0.000000000000000000 ) ) ;
#13246=ORIENTED_EDGE ( 'NONE', *, *, #46423, .T. ) ;
#13250=ORIENTED_EDGE ( 'NONE', *, *, #24826, .F. ) ;
#13252=CARTESIAN_POINT ( 'NONE',  ( -11.34677089036000019, -76.65391306960999884, -4.575788746496000314 ) ) ;
#13263=CARTESIAN_POINT ( 'NONE',  ( -0.9512330062464997571, -78.13175697154288457, 11.17646036812999633 ) ) ;
#13266=CARTESIAN_POINT ( 'NONE',  ( -10.34326456654000026, -78.87006834348099460, 4.339929572939999147 ) ) ;
#13281=CARTESIAN_POINT ( 'NONE',  ( 5.622824352109999424, -79.91678498981538326, -9.705769245306999693 ) ) ;
#13282=CARTESIAN_POINT ( 'NONE',  ( -10.75000000000000000, -78.00000000000000000, 2.252154972635999871E-14 ) ) ;
#13283=AXIS2_PLACEMENT_3D ( 'NONE', #18215, #32052, #36206 ) ;
#13288=CARTESIAN_POINT ( 'NONE',  ( -9.690626710582000314, -78.04833130027799371, -7.043281791253000357 ) ) ;
#13290=CARTESIAN_POINT ( 'NONE',  ( 4.881373948557000020, -78.23512198850700372, -10.89071580847000220 ) ) ;
#13295=CARTESIAN_POINT ( 'NONE',  ( -6.040190233171999878, -79.94824811525009522, 9.093484917090998820 ) ) ;
#13305=CARTESIAN_POINT ( 'NONE',  ( -10.64045665439999944, -76.48390739571800623, -6.341743875680000642 ) ) ;
#13309=CARTESIAN_POINT ( 'NONE',  ( 8.588590363140999884, -79.97061154526829796, -7.284921508032001114 ) ) ;
#13312=DIRECTION ( 'NONE',  ( -1.000000000000000000, 0.000000000000000000, 0.000000000000000000 ) ) ;
#13317=CARTESIAN_POINT ( 'NONE',  ( -11.90546970521999981, -77.80688910291300431, 3.009247460619000059 ) ) ;
#13330=CARTESIAN_POINT ( 'NONE',  ( 7.037082147462999870, -78.32249282818800395, -8.217099986793998667 ) ) ;
#13334=CARTESIAN_POINT ( 'NONE',  ( -5.268979267983999293, -78.61222999764899555, 9.902321347348999936 ) ) ;
#13335=CARTESIAN_POINT ( 'NONE',  ( -0.4565665923329550457, -81.00000000000000000, 10.78468286928460351 ) ) ;
#13337=ORIENTED_EDGE ( 'NONE', *, *, #24078, .F. ) ;
#13347=CARTESIAN_POINT ( 'NONE',  ( 0.000000000000000000, -75.15999999999999659, 0.000000000000000000 ) ) ;
#13354=CARTESIAN_POINT ( 'NONE',  ( 12.31128233177999931, -79.68873324023100224, -0.3719124246491999908 ) ) ;
#13355=CARTESIAN_POINT ( 'NONE',  ( 8.818917551212999584, -75.94225605456199446, 6.571393569026001025 ) ) ;
#13356=CARTESIAN_POINT ( 'NONE',  ( -6.844313060652878811, -78.03000987509473418, 8.289561653482776293 ) ) ;
#13357=CARTESIAN_POINT ( 'NONE',  ( 0.9627474882855999727, -78.26529635310198785, -11.94107121277999894 ) ) ;
#13363=CARTESIAN_POINT ( 'NONE',  ( -8.674044796698000326, -76.83844565707200047, 6.768505387188000988 ) ) ;
#13364=CARTESIAN_POINT ( 'NONE',  ( 11.99999999999999822, -78.06041666666666856, 1.570796326794923203 ) ) ;
#13366=VERTEX_POINT ( 'NONE', #17550 ) ;
#13373=CARTESIAN_POINT ( 'NONE',  ( -10.17713110909000029, -76.66378392136499542, 4.716330562529999604 ) ) ;
#13379=FACE_OUTER_BOUND ( 'NONE', #27190, .T. ) ;
#13382=CARTESIAN_POINT ( 'NONE',  ( -10.11369910513000114, -76.67433028348600033, 4.686934626122000402 ) ) ;
#13388=FACE_OUTER_BOUND ( 'NONE', #4325, .T. ) ;
#13389=CARTESIAN_POINT ( 'NONE',  ( 0.7641671376257024306, -80.23108036345902860, -10.72413782510657931 ) ) ;
#13393=LINE ( 'NONE', #31394, #17922 ) ;
#13395=CARTESIAN_POINT ( 'NONE',  ( 10.05750832943000006, -79.67661227141499580, 4.806363154649000435 ) ) ;
#13408=FACE_OUTER_BOUND ( 'NONE', #5157, .T. ) ;
#13409=CARTESIAN_POINT ( 'NONE',  ( 5.530078818784999406, -79.80792107344059616, -9.545677681241999224 ) ) ;
#13417=CARTESIAN_POINT ( 'NONE',  ( -2.653227710365042125, -77.00733822163999776, -11.74665041585868153 ) ) ;
#13424=DIRECTION ( 'NONE',  ( 0.000000000000000000, 0.000000000000000000, -1.000000000000000000 ) ) ;
#13430=CARTESIAN_POINT ( 'NONE',  ( 11.68767212001977995, -76.57083333333332575, 3.140974612311385972 ) ) ;
#13434=CARTESIAN_POINT ( 'NONE',  ( 1.328862289696999932, -80.26727390273069318, 11.18676134159000135 ) ) ;
#13455=CARTESIAN_POINT ( 'NONE',  ( 3.140974612311376646, -79.04583333333333428, -11.68767212001978706 ) ) ;
#13462=CARTESIAN_POINT ( 'NONE',  ( 4.066926578147327831, -77.25590895697494886, -9.998169505304765892 ) ) ;
#13467=CARTESIAN_POINT ( 'NONE',  ( -8.850953919802000414, -79.76088734065699271, -8.146641040006999290 ) ) ;
#13468=CYLINDRICAL_SURFACE ( 'NONE', #15261, 9.599999999999999645 ) ;
#13470=CARTESIAN_POINT ( 'NONE',  ( 11.90740810048999876, -78.87878573459099130, 0.8057021066547999100 ) ) ;
#13472=ORIENTED_EDGE ( 'NONE', *, *, #57938, .T. ) ;
#13484=ORIENTED_EDGE ( 'NONE', *, *, #36548, .F. ) ;
#13489=CARTESIAN_POINT ( 'NONE',  ( -5.052420809101000088E-14, -80.84999999994218456, 0.000000000000000000 ) ) ;
#13492=CARTESIAN_POINT ( 'NONE',  ( 9.148490208346998998, -77.95585066807355190, 7.734416031130999514 ) ) ;
#13493=B_SPLINE_CURVE_WITH_KNOTS ( 'NONE', 3,
 ( #20001, #20572, #28829, #52165 ),
 .UNSPECIFIED., .F., .F.,
 ( 4, 4 ),
 ( 0.000000000000000000, 1.000000000000000000 ),
 .UNSPECIFIED. ) ;
#13505=CARTESIAN_POINT ( 'NONE',  ( -3.518954327950687855, -78.19866318821630102, -10.19196483504709505 ) ) ;
#13512=CARTESIAN_POINT ( 'NONE',  ( -9.731251526955000841, -77.56402055093700199, -4.947535720883000643 ) ) ;
#13513=CARTESIAN_POINT ( 'NONE',  ( 10.58601714202000110, -77.15014181984899722, -5.993221192758000804 ) ) ;
#13518=ORIENTED_EDGE ( 'NONE', *, *, #49057, .T. ) ;
#13522=CARTESIAN_POINT ( 'NONE',  ( 5.035646364706000355, -79.91077779019330762, 9.842428139517000574 ) ) ;
#13528=CARTESIAN_POINT ( 'NONE',  ( 5.902036703393280348, -79.79999999999999716, -10.23561245371837103 ) ) ;
#13552=CARTESIAN_POINT ( 'NONE',  ( 7.186413748181999850, -76.51672644249900657, 10.04705466018000060 ) ) ;
#13553=CARTESIAN_POINT ( 'NONE',  ( -9.576266473187072137, -78.63770102887031044, -4.884198570897098080 ) ) ;
#13559=CARTESIAN_POINT ( 'NONE',  ( 2.187315676234173889, -78.39085115783234414, -10.82293057966254146 ) ) ;
#13573=CARTESIAN_POINT ( 'NONE',  ( -1.984586691443999795, -76.09012359603299558, 11.75553522549000007 ) ) ;
#13577=CARTESIAN_POINT ( 'NONE',  ( 10.89876807034000095, -79.48100350178651752, -2.652350870517000025 ) ) ;
#13588=CARTESIAN_POINT ( 'NONE',  ( 8.586577278446998918, -80.32955691727549663, 6.741381070085999738 ) ) ;
#13603=CARTESIAN_POINT ( 'NONE',  ( -8.415968974905998934, -79.83442983025919659, -7.483677623529000122 ) ) ;
#13608=AXIS2_PLACEMENT_3D ( 'NONE', #32712, #32423, #32134 ) ;
#13615=CARTESIAN_POINT ( 'NONE',  ( 1.407171709420391936, -78.36458333333330017, 10.75000000000000178 ) ) ;
#13617=ORIENTED_EDGE ( 'NONE', *, *, #6832, .F. ) ;
#13625=CARTESIAN_POINT ( 'NONE',  ( -9.904830252356999765, -76.53887615466000227, 4.590139709818999769 ) ) ;
#13631=CARTESIAN_POINT ( 'NONE',  ( 3.632329907060999563, -80.11446594902099605, 10.45854222826000068 ) ) ;
#13632=CARTESIAN_POINT ( 'NONE',  ( -3.321932689530000093, -81.00000000000000000, 10.22385755016999909 ) ) ;
#13633=ADVANCED_FACE ( 'NONE', ( #52634 ), #21472, .F. ) ;
#13645=FACE_OUTER_BOUND ( 'NONE', #38302, .T. ) ;
#13651=CARTESIAN_POINT ( 'NONE',  ( 4.651654258968999756, -78.85273590260798926, 11.27872058466000027 ) ) ;
#13652=CARTESIAN_POINT ( 'NONE',  ( -4.555356488974000584, -76.23334861441699672, -10.42320189042000145 ) ) ;
#13653=CARTESIAN_POINT ( 'NONE',  ( -7.605247279250050063, -78.03754162542841755, 7.597531084364455900 ) ) ;
#13654=CARTESIAN_POINT ( 'NONE',  ( 4.458743082292000004, -77.54633475908899243, 11.11915799896999957 ) ) ;
#13661=CARTESIAN_POINT ( 'NONE',  ( -6.940497389897999803, -77.31962105010399000, 8.722619821570999576 ) ) ;
#13663=CARTESIAN_POINT ( 'NONE',  ( -11.12160752800000019, -80.38646597062809462, 0.6534909853495001197 ) ) ;
#13668=CARTESIAN_POINT ( 'NONE',  ( -3.513443458492000016, -78.36575305475099640, -10.65240647004999985 ) ) ;
#13671=CARTESIAN_POINT ( 'NONE',  ( -10.31421052434999908, -76.82175206120300004, 3.823226550887000030 ) ) ;
#13675=DIRECTION ( 'NONE',  ( 0.000000000000000000, -1.000000000000000000, 0.000000000000000000 ) ) ;
#13678=CARTESIAN_POINT ( 'NONE',  ( 11.24465069584000076, -78.02216546898499416, -0.6259355293341001270 ) ) ;
#13686=CARTESIAN_POINT ( 'NONE',  ( -1.407171709420418138, -77.11458333333332860, -10.75000000000000000 ) ) ;
#13687=CARTESIAN_POINT ( 'NONE',  ( 6.085875563858039072, -78.52078921777335552, -9.367360191683120618 ) ) ;
#13693=CARTESIAN_POINT ( 'NONE',  ( 10.86346900787000003, -79.15912175438100462, 2.497927478100999910 ) ) ;
#13708=CARTESIAN_POINT ( 'NONE',  ( 10.74994452723989902, -78.34149450793825054, -1.150020074288363947 ) ) ;
#13721=CARTESIAN_POINT ( 'NONE',  ( 2.020917172280999985, -76.38672914931899527, 10.69515428681999936 ) ) ;
#13725=CARTESIAN_POINT ( 'NONE',  ( 6.985849709488999970, -80.94433431827630443, -8.837815942395002011 ) ) ;
#13726=CARTESIAN_POINT ( 'NONE',  ( 9.596002108778145967, -76.60208333333332575, 7.374560639699001996 ) ) ;
#13728=CARTESIAN_POINT ( 'NONE',  ( 10.75000000000000000, -79.84999999999999432, -2.184490103126999767E-14 ) ) ;
#13731=CARTESIAN_POINT ( 'NONE',  ( -6.474781754604000739, -80.47795770475610766, -9.218806710208998112 ) ) ;
#13735=FACE_OUTER_BOUND ( 'NONE', #33484, .T. ) ;
#13740=DIRECTION ( 'NONE',  ( 0.000000000000000000, 0.000000000000000000, -1.000000000000000000 ) ) ;
#13746=CARTESIAN_POINT ( 'NONE',  ( 10.75000000000000000, -76.75000000000000000, 0.000000000000000000 ) ) ;
#13753=CARTESIAN_POINT ( 'NONE',  ( 0.1205599503558857782, -77.22598671500267642, -10.74930044307334143 ) ) ;
#13762=CARTESIAN_POINT ( 'NONE',  ( -3.103176923767000162, -78.29540922883299459, -11.64328410086999988 ) ) ;
#13763=ORIENTED_EDGE ( 'NONE', *, *, #24578, .T. ) ;
#13781=CARTESIAN_POINT ( 'NONE',  ( -3.545645331619000196, -77.54891093671713520, 11.44309676683000454 ) ) ;
#13783=CARTESIAN_POINT ( 'NONE',  ( 11.84266115483542237, -77.13516788874333940, -2.236516232491894129 ) ) ;
#13788=CARTESIAN_POINT ( 'NONE',  ( -3.708203932498999933, -76.29999999999999716, 11.41267819554000162 ) ) ;
#13802=CARTESIAN_POINT ( 'NONE',  ( -9.269928330473998557, -77.48231152193199023, 5.765743207788000646 ) ) ;
#13804=ADVANCED_FACE ( 'NONE', ( #40641 ), #53057, .F. ) ;
#13805=CARTESIAN_POINT ( 'NONE',  ( 9.377644441546999943, -77.67925969475899706, 7.928150093746000771 ) ) ;
#13810=VECTOR ( 'NONE', #4002, 1000.000000000000000 ) ;
#13815=CARTESIAN_POINT ( 'NONE',  ( 10.18685315996999918, -79.41692849819099820, 6.201925135593000071 ) ) ;
#13816=CARTESIAN_POINT ( 'NONE',  ( 10.19393895163000074, -80.85504031229137922, 4.279748970186999735 ) ) ;
#13817=CIRCLE ( 'NONE', #3458, 9.599999999999999645 ) ;
#13819=DIRECTION ( 'NONE',  ( 0.000000000000000000, 0.000000000000000000, -1.000000000000000000 ) ) ;
#13820=CARTESIAN_POINT ( 'NONE',  ( -8.728447447808001414, -76.78120346591698819, 6.810956705545000212 ) ) ;
#13821=DIRECTION ( 'NONE',  ( -1.000000000000000000, 0.000000000000000000, 0.000000000000000000 ) ) ;
#13839=EDGE_LOOP ( 'NONE', ( #31691, #40500, #36846, #40212 ) ) ;
#13844=CARTESIAN_POINT ( 'NONE',  ( -8.648668203041999902, -77.25441573198799006, -8.819734393706001541 ) ) ;
#13845=EDGE_CURVE ( 'NONE', #12674, #28730, #13393, .T. ) ;
#13856=CARTESIAN_POINT ( 'NONE',  ( -3.140974612311351777, -78.90416666666668277, -11.68767212001978884 ) ) ;
#13870=CARTESIAN_POINT ( 'NONE',  ( 6.725657209017000149, -77.30646084297899279, -9.843613558058999402 ) ) ;
#13875=ORIENTED_EDGE ( 'NONE', *, *, #29617, .T. ) ;
#13879=CARTESIAN_POINT ( 'NONE',  ( 2.697636866285999968, -77.64139156892099436, -11.67213861177999945 ) ) ;
#13882=CARTESIAN_POINT ( 'NONE',  ( -10.23070583620000207, -78.53354445816799512, 6.145580569783000158 ) ) ;
#13886=CARTESIAN_POINT ( 'NONE',  ( -9.543280303650000462, -79.56693931322499225, -5.301053389303000074 ) ) ;
#13896=CARTESIAN_POINT ( 'NONE',  ( 10.74999999999999822, -76.75923966921678243, 1.248172908123839076 ) ) ;
#13897=EDGE_LOOP ( 'NONE', ( #7750, #3537, #50676, #30892 ) ) ;
#13899=CARTESIAN_POINT ( 'NONE',  ( -9.674930971187000850, -79.16750321980599381, 5.536272326541999078 ) ) ;
#13901=CARTESIAN_POINT ( 'NONE',  ( 11.49045096393965082, -79.78080184933774888, -2.827711266468116325 ) ) ;
#13908=DIRECTION ( 'NONE',  ( 0.000000000000000000, -1.000000000000000000, 0.000000000000000000 ) ) ;
#13911=B_SPLINE_CURVE_WITH_KNOTS ( 'NONE', 3,
 ( #29410, #52443, #8723, #21714, #22000, #8144, #48885, #8427, #57727, #17284, #21137, #26716, #58023, #17584, #12283, #35571, #39144, #40312, #48598, #34701, #52732, #7853, #21430, #993, #27229, #4524, #45563, #32526, #36100, #49402, #49697, #54117, #5108, #8951, #40827, #18979, #45268, #36971, #40534, #54984, #129, #9830, #50569, #18105, #49992, #58248, #4817, #10124, #44672, #4225, #23107, #22816, #419, #18397, #22223, #36388, #54415, #13951, #31947, #9538, #27521, #709, #36680, #15706, #32818, #33701, #56157, #11001, #56445, #46740, #42872, #50864, #37260, #46152, #51740, #28395, #2429, #10410, #46442, #42582, #5676, #33411, #11289, #5970, #29269, #6846, #33115, #24856, #51156, #23975, #28986, #16000, #19553, #55274, #23687, #55868, #20432, #1276, #41993, #1561, #38427, #33987, #37551 ),
 .UNSPECIFIED., .F., .F.,
 ( 4, 2, 2, 2, 1, 1, 1, 1, 1, 2, 2, 2, 2, 2, 1, 1, 1, 1, 2, 2, 2, 2, 2, 1, 1, 1, 2, 2, 2, 1, 1, 1, 1, 1, 2, 2, 2, 2, 2, 1, 1, 1, 1, 2, 2, 2, 2, 2, 1, 1, 1, 1, 1, 2, 2, 2, 2, 2, 1, 1, 1, 1, 1, 2, 2, 2, 4 ),
 ( 0.000000000000000000, 0.06249999999999299172, 0.09374999999998949451, 0.1093749999999877598, 0.1171874999999868716, 0.1210937499999864414, 0.1230468749999862610, 0.1240234374999861777, 0.1245117187499861083, 0.1247558593749860389, 0.1249999999999859696, 0.1874999999999704681, 0.2187499999999626965, 0.2343749999999588107, 0.2421874999999568678, 0.2460937499999558964, 0.2480468749999554245, 0.2490234374999552025, 0.2495117187499550637, 0.2499999999999549249, 0.3124999999999380496, 0.3437499999999296119, 0.3593749999999253930, 0.3671874999999233391, 0.3710937499999223954, 0.3730468749999218958, 0.3740234374999217293, 0.3749999999999216183, 0.4374999999999110711, 0.4687499999999057976, 0.4843749999999031886, 0.4921874999999019118, 0.4960937499999012457, 0.4980468749999010236, 0.4990234374999010236, 0.4999999999999010236, 0.5624999999999098499, 0.5937499999999141798, 0.6093749999999164002, 0.6171874999999173994, 0.6210937499999178435, 0.6230468749999181766, 0.6240234374999182876, 0.6245117187499182876, 0.6249999999999183986, 0.6874999999999239497, 0.7187499999999266143, 0.7343749999999279465, 0.7421874999999286127, 0.7460937499999290567, 0.7480468749999292788, 0.7490234374999293898, 0.7495117187499295008, 0.7497558593749296119, 0.7499999999999296119, 0.8124999999999150679, 0.8437499999999077405, 0.8593749999999040767, 0.8671874999999023004, 0.8710937499999014122, 0.8730468749999009681, 0.8740234374999007461, 0.8745117187499007461, 0.8747558593749006350, 0.8749999999999006350, 0.9374999999999502620, 1.000000000000000000 ),
 .UNSPECIFIED. ) ;
#13912=CARTESIAN_POINT ( 'NONE',  ( 5.413904038987143785, -79.33333333333332860, 9.393203674808290771 ) ) ;
#13913=CARTESIAN_POINT ( 'NONE',  ( -8.596418555780466875, -78.44791666666665719, 6.606377239730298001 ) ) ;
#13916=ORIENTED_EDGE ( 'NONE', *, *, #48693, .T. ) ;
#13918=CARTESIAN_POINT ( 'NONE',  ( -3.463640081230069168, -77.69897920905084732, -10.20056251384204771 ) ) ;
#13920=CARTESIAN_POINT ( 'NONE',  ( -11.08400893144000143, -76.26062989717654261, -1.489506537590000068 ) ) ;
#13925=CARTESIAN_POINT ( 'NONE',  ( 5.865103843792000227, -78.43489146390899691, -9.561319920857000554 ) ) ;
#13944=CARTESIAN_POINT ( 'NONE',  ( -1.794013086462000084, -79.82776776362139515, 12.18547446480999952 ) ) ;
#13945=CARTESIAN_POINT ( 'NONE',  ( 8.239941435165000883, -76.45166803430799973, 7.842062413654000252 ) ) ;
#13946=CARTESIAN_POINT ( 'NONE',  ( -7.609103215824061905, -78.03758286351242646, 7.593670151128505630 ) ) ;
#13951=CARTESIAN_POINT ( 'NONE',  ( 7.526684410834897143, -80.91343724093917444, 7.679016378754886851 ) ) ;
#13954=CARTESIAN_POINT ( 'NONE',  ( -4.503658352096000073, -77.48303910811499406, -10.19664954867000084 ) ) ;
#13956=CARTESIAN_POINT ( 'NONE',  ( 4.337443150956000082, -81.11643595646388860, -9.985393166669998877 ) ) ;
#13962=CARTESIAN_POINT ( 'NONE',  ( -10.93308570624999909, -78.28404402574500409, -2.507139558745000052 ) ) ;
#13974=CARTESIAN_POINT ( 'NONE',  ( 10.72689817447000138, -77.43694788753698788, -3.031213639016000272 ) ) ;
#13980=CARTESIAN_POINT ( 'NONE',  ( -5.970499261319586637, -80.17821983607609582, -8.939495840307154495 ) ) ;
#13981=CARTESIAN_POINT ( 'NONE',  ( 9.393203674808285442, -77.20833333333332860, -5.413904038987152667 ) ) ;
#13982=CARTESIAN_POINT ( 'NONE',  ( -11.04080913941738196, -79.33578427474678563, 1.980439979086550117 ) ) ;
#13986=CARTESIAN_POINT ( 'NONE',  ( 11.08725735368000009, -79.64937592841299363, 1.152095891907999992 ) ) ;
#14001=B_SPLINE_CURVE_WITH_KNOTS ( 'NONE', 3,
 ( #1512, #19501, #13901, #5623, #23052, #37496, #55517, #54650, #14767, #9484, #6207, #23634, #41068, #14189, #15064, #32186, #32765, #50226, #41647, #33058, #27762, #1226, #19216, #50812, #28338, #10355, #45805, #46390, #23347, #941, #18923, #24511, #7369, #47838, #2667, #38083, #7084, #25654, #47559, #20662, #11239, #38660, #15367, #25370, #16236, #56106, #29782, #47263, #2944, #48123, #33360, #52533, #56680, #28930, #20944, #38371, #11527, #20093, #43109, #56393, #15944, #34504, #51393, #10949, #29505, #19800, #34215, #12090, #38947, #55814, #52251, #15652, #42815, #43385, #11808, #56962, #2096, #16524, #30073 ),
 .UNSPECIFIED., .F., .F.,
 ( 4, 2, 2, 2, 2, 2, 2, 2, 2, 2, 2, 2, 2, 2, 2, 2, 2, 1, 2, 2, 2, 2, 2, 2, 2, 2, 2, 2, 2, 2, 2, 2, 2, 2, 2, 2, 2, 2, 2, 4 ),
 ( 0.000000000000000000, 0.03125000000000011102, 0.06250000000000022204, 0.07812500000000023592, 0.09375000000000023592, 0.1250000000000002498, 0.1562500000000002776, 0.1875000000000002776, 0.2187500000000002776, 0.2500000000000002776, 0.2656250000000002776, 0.2812500000000002776, 0.3125000000000002776, 0.3437500000000003331, 0.3750000000000003331, 0.4062500000000003331, 0.4218750000000003331, 0.4375000000000003331, 0.4531250000000003331, 0.4687500000000003331, 0.5000000000000003331, 0.5312500000000003331, 0.5625000000000003331, 0.5937500000000003331, 0.6093750000000002220, 0.6250000000000002220, 0.6562500000000002220, 0.6875000000000002220, 0.7187500000000002220, 0.7500000000000002220, 0.7812500000000002220, 0.7968750000000001110, 0.8125000000000001110, 0.8437500000000001110, 0.8750000000000001110, 0.9062500000000001110, 0.9375000000000001110, 0.9687500000000001110, 0.9843750000000000000, 1.000000000000000000 ),
 .UNSPECIFIED. ) ;
#14016=CARTESIAN_POINT ( 'NONE',  ( -6.711381441964999972, -80.12410361490928778, 9.048015653393999713 ) ) ;
#14019=CARTESIAN_POINT ( 'NONE',  ( 11.89973958376643992, -76.19973958328499464, -1.558524492839146403 ) ) ;
#14022=CARTESIAN_POINT ( 'NONE',  ( 0.000000000000000000, -81.00000000000000000, 0.000000000000000000 ) ) ;
#14023=CARTESIAN_POINT ( 'NONE',  ( -11.03620408507000050, -80.41776233274890728, -2.260839449595000161 ) ) ;
#14027=CARTESIAN_POINT ( 'NONE',  ( -10.75000000000000000, -78.60000000000000853, 0.000000000000000000 ) ) ;
#14035=CARTESIAN_POINT ( 'NONE',  ( -3.921304417499244188, -79.50486137303013834, 10.00992689042903905 ) ) ;
#14048=CARTESIAN_POINT ( 'NONE',  ( 0.000000000000000000, -90.29999999999999716, 0.000000000000000000 ) ) ;
#14050=VERTEX_POINT ( 'NONE', #43195 ) ;
#14051=CARTESIAN_POINT ( 'NONE',  ( 6.710021342196546890, -77.27873848259581280, -8.417207788637705690 ) ) ;
#14054=ORIENTED_EDGE ( 'NONE', *, *, #41008, .T. ) ;
#14056=CARTESIAN_POINT ( 'NONE',  ( -11.15966350340000091, -79.67123644811400140, 4.490997254915999548 ) ) ;
#14057=FACE_OUTER_BOUND ( 'NONE', #16344, .T. ) ;
#14058=DIRECTION ( 'NONE',  ( -1.000000000000000000, 0.000000000000000000, 0.000000000000000000 ) ) ;
#14061=CARTESIAN_POINT ( 'NONE',  ( 2.241689414777999989, -78.05124539001899109, 11.83936654731000004 ) ) ;
#14066=CARTESIAN_POINT ( 'NONE',  ( -1.570796326794938524, -78.68541666666666856, 11.99999999999999645 ) ) ;
#14070=B_SPLINE_CURVE_WITH_KNOTS ( 'NONE', 3,
 ( #50972, #19666, #32634, #37076, #46263, #32928, #37954, #24389, #10523, #42689, #55977, #28506, #51558, #46556, #2253, #55682, #6081, #33806 ),
 .UNSPECIFIED., .F., .F.,
 ( 4, 2, 2, 2, 2, 2, 2, 2, 4 ),
 ( 0.000000000000000000, 0.1250000000000000000, 0.2500000000000000000, 0.3750000000000000000, 0.5000000000000000000, 0.6250000000000000000, 0.7500000000000000000, 0.8750000000000000000, 1.000000000000000000 ),
 .UNSPECIFIED. ) ;
#14073=AXIS2_PLACEMENT_3D ( 'NONE', #35220, #26372, #21663 ) ;
#14076=CARTESIAN_POINT ( 'NONE',  ( 0.000000000000000000, -75.15999999999999659, 0.000000000000000000 ) ) ;
#14078=CARTESIAN_POINT ( 'NONE',  ( -1.432420283025999996, -76.08353766477399915, 11.09153081809999897 ) ) ;
#14104=CARTESIAN_POINT ( 'NONE',  ( 6.606416481926000728, -77.54361311763999254, -10.35137867379999932 ) ) ;
#14110=CARTESIAN_POINT ( 'NONE',  ( -3.693060907207000199, -79.52346302158100855, 11.34006851057000098 ) ) ;
#14111=CARTESIAN_POINT ( 'NONE',  ( -1.088868221116000123, -80.19055927822239482, -11.00213361798000022 ) ) ;
#14113=CYLINDRICAL_SURFACE ( 'NONE', #3052, 10.75000000000000000 ) ;
#14120=CARTESIAN_POINT ( 'NONE',  ( -8.156245788203044356, -76.13854166665944945, 7.337572461140913660 ) ) ;
#14156=DIRECTION ( 'NONE',  ( 1.000000000000000000, 0.000000000000000000, 0.000000000000000000 ) ) ;
#14163=EDGE_CURVE ( 'NONE', #46988, #20674, #34831, .T. ) ;
#14166=CARTESIAN_POINT ( 'NONE',  ( 10.42503750987000011, -77.20732252214099844, -5.902083371034000159 ) ) ;
#14169=CARTESIAN_POINT ( 'NONE',  ( 12.04731061283000138, -77.76045519273699824, 0.2409951698105000095 ) ) ;
#14172=CARTESIAN_POINT ( 'NONE',  ( 10.85828250482999913, -79.78483005723899169, 1.128302723381999995 ) ) ;
#14177=EDGE_CURVE ( 'NONE', #13366, #1523, #54666, .T. ) ;
#14182=CARTESIAN_POINT ( 'NONE',  ( 0.4258703671788000023, -76.00112020995099726, -12.49690866505999942 ) ) ;
#14187=CARTESIAN_POINT ( 'NONE',  ( 9.395013887366999938, -79.00408516179498974, 5.999026139886999509 ) ) ;
#14189=CARTESIAN_POINT ( 'NONE',  ( -4.106759750389861630, -79.64664839926052764, -11.09893327577296773 ) ) ;
#14195=EDGE_CURVE ( 'NONE', #13166, #32124, #17517, .T. ) ;
#14203=CARTESIAN_POINT ( 'NONE',  ( 8.197432492207889609, -78.79411831125318599, -6.956612881758995393 ) ) ;
#14210=CARTESIAN_POINT ( 'NONE',  ( -11.14725709413418997, -77.08267626182042420, -4.956903492521361976 ) ) ;
#14211=CARTESIAN_POINT ( 'NONE',  ( -8.885737597169484303, -77.99140041745337726, 8.035151442397836519 ) ) ;
#14212=CARTESIAN_POINT ( 'NONE',  ( 2.315902194296999728, -78.40765512090699474, -10.97517055051999968 ) ) ;
#14213=CARTESIAN_POINT ( 'NONE',  ( -1.714140276207581914, -81.00000000000000000, 10.66650235410891767 ) ) ;
#14222=DIRECTION ( 'NONE',  ( 0.000000000000000000, -1.000000000000000000, 0.000000000000000000 ) ) ;
#14223=CARTESIAN_POINT ( 'NONE',  ( -1.570796326794884790, -78.51458333333332007, -12.00000000000000355 ) ) ;
#14228=DIRECTION ( 'NONE',  ( 1.000000000000000000, 0.000000000000000000, 2.044033345361000115E-13 ) ) ;
#14231=CARTESIAN_POINT ( 'NONE',  ( -3.807671504463999934, -79.34114693175598632, 11.71356677268999924 ) ) ;
#14233=CARTESIAN_POINT ( 'NONE',  ( -11.47220708781999932, -76.21374791087299627, -0.7050395033892999930 ) ) ;
#14234=CARTESIAN_POINT ( 'NONE',  ( 9.574729143547433097, -77.88772600167752103, 4.887204184123924655 ) ) ;
#14235=CARTESIAN_POINT ( 'NONE',  ( 4.374544387491000386, -77.35642955112200525, -11.15253550093999912 ) ) ;
#14239=FACE_OUTER_BOUND ( 'NONE', #54405, .T. ) ;
#14243=CARTESIAN_POINT ( 'NONE',  ( -6.771245932390999478, -78.53127452059300140, -8.709304295962999376 ) ) ;
#14244=CARTESIAN_POINT ( 'NONE',  ( -6.940239200437514633, -76.07416453009285817, 9.811877043595169212 ) ) ;
#14245=CARTESIAN_POINT ( 'NONE',  ( -9.059593803572999704, -80.91060369710268674, 6.284180259888000109 ) ) ;
#14249=CARTESIAN_POINT ( 'NONE',  ( -2.309466437479000156, -77.58981958342698704, 10.97654204954999990 ) ) ;
#14254=CARTESIAN_POINT ( 'NONE',  ( -1.078940792280719041, -78.61703581007959940, -10.72803815209405087 ) ) ;
#14260=CARTESIAN_POINT ( 'NONE',  ( -10.21813353151999948, -76.74205734789899225, 4.735332084273999875 ) ) ;
#14266=CARTESIAN_POINT ( 'NONE',  ( -7.595992864760312102, -80.16301844581369096, -7.606389479688519195 ) ) ;
#14268=EDGE_CURVE ( 'NONE', #10604, #33417, #47146, .T. ) ;
#14273=CARTESIAN_POINT ( 'NONE',  ( -10.64923527428000050, -79.86726667242790256, 3.293689214829000012 ) ) ;
#14278=ORIENTED_EDGE ( 'NONE', *, *, #38507, .T. ) ;
#14280=EDGE_LOOP ( 'NONE', ( #52473, #32853, #53469, #10521 ) ) ;
#14289=ORIENTED_EDGE ( 'NONE', *, *, #1014, .T. ) ;
#14290=EDGE_LOOP ( 'NONE', ( #10097, #39817, #30380 ) ) ;
#14304=CARTESIAN_POINT ( 'NONE',  ( 1.618170588614999961, -80.40257597021090419, -11.14857479085000058 ) ) ;
#14314=CARTESIAN_POINT ( 'NONE',  ( -5.052420809101000088E-14, -80.89999999999999147, -13.99999999999777955 ) ) ;
#14320=CARTESIAN_POINT ( 'NONE',  ( -8.940100391463808194, -79.55319689977089581, 5.969627096040645675 ) ) ;
#14327=B_SPLINE_CURVE_WITH_KNOTS ( 'NONE', 3,
 ( #51229, #24638, #19925, #6630, #14603, #32890, #5462, #2217, #6040, #20218, #37624, #19049, #37334, #37039, #37915, #45929, #50935, #42650 ),
 .UNSPECIFIED., .F., .F.,
 ( 4, 2, 2, 2, 2, 2, 2, 2, 4 ),
 ( 0.000000000000000000, 0.1250000000000000278, 0.2500000000000000555, 0.3750000000000000000, 0.5000000000000000000, 0.6250000000000000000, 0.7500000000000000000, 0.8750000000000001110, 1.000000000000000000 ),
 .UNSPECIFIED. ) ;
#14335=ORIENTED_EDGE ( 'NONE', *, *, #50760, .F. ) ;
#14345=CARTESIAN_POINT ( 'NONE',  ( 11.43454631689000145, -77.91559881290099554, -3.800910706745999956 ) ) ;
#14350=EDGE_CURVE ( 'NONE', #28435, #27557, #55639, .T. ) ;
#14351=CARTESIAN_POINT ( 'NONE',  ( 1.570391623911302492, -76.53481037454862701, -11.99908637137544076 ) ) ;
#14359=CARTESIAN_POINT ( 'NONE',  ( -12.00000000000000000, -79.79999999999999716, 6.639246269807000381E-13 ) ) ;
#14361=CARTESIAN_POINT ( 'NONE',  ( 5.177752511601999785, -76.60280117385499921, 9.912858493839999952 ) ) ;
#14365=CARTESIAN_POINT ( 'NONE',  ( 1.552784181637999916, -76.45944931795999366, -11.12081786967999975 ) ) ;
#14377=DIRECTION ( 'NONE',  ( 0.000000000000000000, 1.000000000000000000, -7.105427357601000597E-14 ) ) ;
#14378=B_SPLINE_SURFACE_WITH_KNOTS ( 'NONE', 3, 3, ( 
 ( #28525, #15250, #37974, #27651, #6393, #36804, #55998, #24408, #32076, #42126, #50408, #55702, #33243, #10841, #28817, #14365, #46866, #9957, #27938, #50117, #9661, #45693, #5232, #45986, #5512, #23522, #41533, #39430, #25845, #2844, #20841, #38267, #42710, #47735, #20560 ),
 ( #11995, #11710, #20273, #2559, #38558, #15545, #7269, #47452, #25270, #48024, #33541, #38845, #56288, #51865, #51580, #48306, #2275, #11137, #39136, #6977, #7558, #11418, #15839, #43873, #3140, #24980, #56863, #7845, #29399, #12275, #29973, #34109, #33827, #16422, #43002 ),
 ( #25557, #47159, #56574, #34406, #16132, #52152, #52435, #43577, #21129, #3422, #57147, #16711, #34693, #52723, #30264, #21422, #29113, #6689, #24698, #44738, #8715, #35564, #9016, #36164, #27295, #49765, #4289, #16998, #21992, #35266, #34978, #31717, #26136, #53008, #22587 ),
 ( #21706, #4589, #53894, #45036, #8135, #44436, #44157, #27001, #12561, #40000, #9305, #18171, #35865, #53298, #53590, #40600, #22288, #57437, #196, #30559, #3703, #54183, #58015, #12842, #45331, #49468, #13721, #3989, #17276, #4881, #22878, #8418, #17576, #48590, #39711 ) ),
 .UNSPECIFIED., .F., .F., .F.,
 ( 4, 4 ),
 ( 4, 1, 1, 1, 1, 1, 1, 1, 1, 1, 1, 1, 1, 1, 1, 1, 1, 1, 1, 1, 1, 1, 1, 1, 1, 1, 1, 1, 1, 1, 1, 1, 4 ),
 ( -0.1772706441294000235, 1.177270644128999955 ),
 ( -0.009208997693793000497, 0.005755623558620999794, 0.02072024481102999888, 0.03568486606345000478, 0.05064948731585999786, 0.06561410856827000482, 0.08057872982069000378, 0.09554335107309999686, 0.1105079723255000118, 0.1254725935778999990, 0.1404372148303000001, 0.1554018360827999767, 0.1703664573352000056, 0.1853310785876000066, 0.2002956998400000077, 0.2152603210924000088, 0.2302249423447999821, 0.2451895635972000109, 0.2601541848496000120, 0.2751188061020999887, 0.2900834273544999897, 0.3050480486068999908, 0.3200126698593000474, 0.3349772911116999929, 0.3499419123640999940, 0.3649065336164999951, 0.3798711548689999717, 0.3948357761214000283, 0.4098003973737999739, 0.4247650186261999750, 0.4397296398786000315, 0.4546942611309999771, 0.4696588823833999782 ),
 .UNSPECIFIED. ) ;
#14386=EDGE_CURVE ( 'NONE', #18069, #30361, #46222, .T. ) ;
#14388=CARTESIAN_POINT ( 'NONE',  ( 2.765208115035000080, -77.51648380221600121, -11.96450597650000169 ) ) ;
#14395=CARTESIAN_POINT ( 'NONE',  ( -9.301394811601999990, -79.17722582056299530, -7.464576829628999377 ) ) ;
#14396=CARTESIAN_POINT ( 'NONE',  ( 10.60070852584000001, -80.43093146505920288, -3.881634873714000289 ) ) ;
#14399=CARTESIAN_POINT ( 'NONE',  ( 2.976864594307000011, -77.54805815623998910, -10.81463766284999828 ) ) ;
#14414=CARTESIAN_POINT ( 'NONE',  ( 5.675825126306000001, -79.16335487410098892, 10.88946240266999865 ) ) ;
#14418=ORIENTED_EDGE ( 'NONE', *, *, #48488, .F. ) ;
#14421=CIRCLE ( 'NONE', #49336, 11.70000000000000107 ) ;
#14441=CARTESIAN_POINT ( 'NONE',  ( -1.407171709420418138, -77.61458333333330017, -10.75000000000000000 ) ) ;
#14446=CARTESIAN_POINT ( 'NONE',  ( -8.987350104473000201, -77.14201387919399622, 8.369597699504998545 ) ) ;
#14451=CARTESIAN_POINT ( 'NONE',  ( 11.21665020278000036, -78.50049515372108999, 0.06973997782872000395 ) ) ;
#14458=CARTESIAN_POINT ( 'NONE',  ( 10.24999999991999999, -82.10000000007899246, -6.817370023903000320E-10 ) ) ;
#14462=CARTESIAN_POINT ( 'NONE',  ( -9.926966510012999123, -77.52975978748899877, 6.625016102256999773 ) ) ;
#14465=CARTESIAN_POINT ( 'NONE',  ( -8.917244775899000331, -79.00895807477898813, -6.494958043606000153 ) ) ;
#14470=CARTESIAN_POINT ( 'NONE',  ( 4.774672647477999909, -79.91637558193269797, -11.01515226630999855 ) ) ;
#14472=CARTESIAN_POINT ( 'NONE',  ( -10.57894479237893748, -76.18802083340513320, -2.843887423799716263 ) ) ;
#14480=CARTESIAN_POINT ( 'NONE',  ( -10.69024338110999928, -78.73172173177698596, -3.158052726529999799 ) ) ;
#14496=CARTESIAN_POINT ( 'NONE',  ( 6.499026777884298056, -78.77679667229833171, -8.564691133015255531 ) ) ;
#14498=VERTEX_POINT ( 'NONE', #10014 ) ;
#14499=CARTESIAN_POINT ( 'NONE',  ( 2.076475668830000121, -76.11013824524211202, 10.98918251355999942 ) ) ;
#14503=CARTESIAN_POINT ( 'NONE',  ( 9.211672236691230253, -76.85627983199107405, 7.998575932842224567 ) ) ;
#14504=CARTESIAN_POINT ( 'NONE',  ( 2.697673772653688573, -77.69297794779137689, -11.67229829829229715 ) ) ;
#14505=CARTESIAN_POINT ( 'NONE',  ( -6.324515969367999979, -78.84343660893600259, -9.263833350438000380 ) ) ;
#14524=CARTESIAN_POINT ( 'NONE',  ( -6.043427764450784778, -79.48333333333329165, -10.48543666025109822 ) ) ;
#14525=CARTESIAN_POINT ( 'NONE',  ( 3.001482106993999643, -76.63078604711199660, 11.21790237008999824 ) ) ;
#14526=CARTESIAN_POINT ( 'NONE',  ( 4.627417567202060766, -77.93975844766031003, 9.702993547770001115 ) ) ;
#14527=CARTESIAN_POINT ( 'NONE',  ( -4.085659785884999451, -78.46880095406299915, 11.26159174134999930 ) ) ;
#14530=LINE ( 'NONE', #27519, #33534 ) ;
#14535=CARTESIAN_POINT ( 'NONE',  ( 9.014158510551999015, -78.19118402616200569, 6.557403976990999972 ) ) ;
#14537=CARTESIAN_POINT ( 'NONE',  ( -1.784822011179000079, -80.34680229102650628, 10.88032703863999906 ) ) ;
#14542=CARTESIAN_POINT ( 'NONE',  ( 0.1392748842281999744, -77.07232906639299586, 11.21600254538999941 ) ) ;
#14546=CARTESIAN_POINT ( 'NONE',  ( -10.31401527466070256, -76.75508539453620926, 3.823154250450220282 ) ) ;
#14554=CARTESIAN_POINT ( 'NONE',  ( 0.1398360057836000037, -77.15060249292598371, 11.26119045437999944 ) ) ;
#14564=DIRECTION ( 'NONE',  ( 1.000000000000000000, 0.000000000000000000, 0.000000000000000000 ) ) ;
#14565=CARTESIAN_POINT ( 'NONE',  ( 2.301467643382999917, -78.53268586533900475, -10.90676452780999917 ) ) ;
#14568=ORIENTED_EDGE ( 'NONE', *, *, #10939, .T. ) ;
#14585=CARTESIAN_POINT ( 'NONE',  ( 0.000000000000000000, -92.79999999999999716, 0.000000000000000000 ) ) ;
#14597=CARTESIAN_POINT ( 'NONE',  ( -7.960542989054001595, -80.70355283024726134, 7.971132368775000643 ) ) ;
#14603=CARTESIAN_POINT ( 'NONE',  ( -9.596002108778193929, -78.34791666666664867, 7.374560639698937159 ) ) ;
#14615=CARTESIAN_POINT ( 'NONE',  ( -0.01336421990532181761, -79.47521759444254030, 10.74992168017122651 ) ) ;
#14633=CARTESIAN_POINT ( 'NONE',  ( -3.970056213021999625, -79.10344746201099042, 11.35542513096999961 ) ) ;
#14636=VERTEX_POINT ( 'NONE', #32277 ) ;
#14637=CARTESIAN_POINT ( 'NONE',  ( 4.881373948557000020, -78.28194079526799953, -10.89071580847000220 ) ) ;
#14639=ORIENTED_EDGE ( 'NONE', *, *, #17980, .F. ) ;
#14650=CARTESIAN_POINT ( 'NONE',  ( 0.9597843051886902899, -79.79999999999998295, -11.74187349997137630 ) ) ;
#14651=CARTESIAN_POINT ( 'NONE',  ( -10.75000000000000000, -80.09999999999999432, -1.711887504597999906E-14 ) ) ;
#14653=CARTESIAN_POINT ( 'NONE',  ( -11.08400893143999966, -76.27673592799600044, -1.489506537590000068 ) ) ;
#14661=FACE_OUTER_BOUND ( 'NONE', #56770, .T. ) ;
#14668=CARTESIAN_POINT ( 'NONE',  ( -9.596002108778193929, -79.34791666666664867, 7.374560639698937159 ) ) ;
#14684=CARTESIAN_POINT ( 'NONE',  ( -11.04073130536000136, -80.15336828462439200, -1.710558420931999946 ) ) ;
#14687=CARTESIAN_POINT ( 'NONE',  ( 6.433795189870999742, -77.57529449924099652, -9.188274595716000803 ) ) ;
#14692=CARTESIAN_POINT ( 'NONE',  ( 8.991649895478447618, -80.99999999999998579, -6.337868273171067379 ) ) ;
#14696=CARTESIAN_POINT ( 'NONE',  ( -7.960542989054001595, -80.63576427697100257, 7.971132368775000643 ) ) ;
#14697=DIRECTION ( 'NONE',  ( 0.000000000000000000, 0.000000000000000000, -1.000000000000000000 ) ) ;
#14705=CARTESIAN_POINT ( 'NONE',  ( -5.342744711435999605, -77.84767930019499715, -10.92875150845999954 ) ) ;
#14708=ORIENTED_EDGE ( 'NONE', *, *, #40880, .F. ) ;
#14722=CARTESIAN_POINT ( 'NONE',  ( -11.68767212001979061, -78.82083333333331154, -3.140974612311365988 ) ) ;
#14732=CARTESIAN_POINT ( 'NONE',  ( -1.984586691443999795, -76.02233504275700682, 11.75553522549000007 ) ) ;
#14738=CARTESIAN_POINT ( 'NONE',  ( -11.04065564777999953, -79.23587641477011800, 1.980412446595999798 ) ) ;
#14746=CARTESIAN_POINT ( 'NONE',  ( -8.196454039252000001, -78.57433465545000217, -8.832548491656998735 ) ) ;
#14754=CARTESIAN_POINT ( 'NONE',  ( -8.876652416960000735, -79.81871893549168817, -8.305429993361000740 ) ) ;
#14760=LINE ( 'NONE', #32757, #4414 ) ;
#14765=LINE ( 'NONE', #19144, #7004 ) ;
#14767=CARTESIAN_POINT ( 'NONE',  ( 6.128871534568974155, -79.71851631894477919, -10.04897160984813453 ) ) ;
#14770=DIRECTION ( 'NONE',  ( 0.000000000000000000, 1.000000000000000000, 0.000000000000000000 ) ) ;
#14771=EDGE_CURVE ( 'NONE', #18221, #15288, #18265, .T. ) ;
#14777=CIRCLE ( 'NONE', #22326, 9.599999999999999645 ) ;
#14784=CARTESIAN_POINT ( 'NONE',  ( 5.997500730681496250, -78.77227202905815773, -8.921341173856349727 ) ) ;
#14792=CARTESIAN_POINT ( 'NONE',  ( 12.12015523194605571, -76.29028875741708760, -1.390668883284736923 ) ) ;
#14793=CARTESIAN_POINT ( 'NONE',  ( -9.964686285863574966, -77.50307273982538447, 6.650189363608897786 ) ) ;
#14794=CARTESIAN_POINT ( 'NONE',  ( 9.453938376997999882, -79.06132735295099678, 6.036651369377000087 ) ) ;
#14804=CARTESIAN_POINT ( 'NONE',  ( -6.043427764450784778, -77.48333333333332007, -10.48543666025109822 ) ) ;
#14805=DIRECTION ( 'NONE',  ( 0.000000000000000000, 0.000000000000000000, -1.000000000000000000 ) ) ;
#14815=CARTESIAN_POINT ( 'NONE',  ( 7.103732877834134207, -77.91783737943933374, 8.098743610684461913 ) ) ;
#14816=CARTESIAN_POINT ( 'NONE',  ( -7.615853692923001184, -78.49593026948699048, 9.247423260715999405 ) ) ;
#14818=CARTESIAN_POINT ( 'NONE',  ( 10.40652105080773815, -78.87097662156874378, 2.787377815128531999 ) ) ;
#14823=CARTESIAN_POINT ( 'NONE',  ( -10.00926467875000014, -76.92433028348600033, 4.638537167971000130 ) ) ;
#14824=CARTESIAN_POINT ( 'NONE',  ( -10.85634995915000012, -76.18870722365406323, -5.741293403527000017 ) ) ;
#14825=CARTESIAN_POINT ( 'NONE',  ( -3.078559409956000081, -80.49385671464260383, -10.70699195275999926 ) ) ;
#14830=CARTESIAN_POINT ( 'NONE',  ( -1.407065915474770446, -80.48551767968157833, 10.74861335954481056 ) ) ;
#14832=CARTESIAN_POINT ( 'NONE',  ( -10.86658628928999981, -76.78604516064498853, -2.781249891074999869 ) ) ;
#14840=AXIS2_PLACEMENT_3D ( 'NONE', #823, #50982, #46855 ) ;
#14847=CARTESIAN_POINT ( 'NONE',  ( 1.570796326794909881, -79.43541666666665435, -11.99999999999999822 ) ) ;
#14850=CARTESIAN_POINT ( 'NONE',  ( -7.482244971425966895, -80.16420082495498889, -7.718414027147809442 ) ) ;
#14855=CARTESIAN_POINT ( 'NONE',  ( -9.643902624173000149, -79.49921224881200033, -5.356946570292000054 ) ) ;
#14873=CARTESIAN_POINT ( 'NONE',  ( -10.98749645531777652, -76.93354319426246946, -4.929334125398809441 ) ) ;
#14881=CARTESIAN_POINT ( 'NONE',  ( 6.043427764450763462, -76.73333333333330586, 10.48543666025111065 ) ) ;
#14887=CARTESIAN_POINT ( 'NONE',  ( 3.140974612311327796, -76.65416666666669698, 11.68767212001979594 ) ) ;
#14888=CARTESIAN_POINT ( 'NONE',  ( -8.547594633831460342, -76.65220310981916896, -6.557508948702818863 ) ) ;
#14894=CARTESIAN_POINT ( 'NONE',  ( 6.226899213932999722, -78.49568698277398937, -9.208165984944999494 ) ) ;
#14901=ADVANCED_FACE ( 'NONE', ( #54851 ), #52800, .F. ) ;
#14904=CARTESIAN_POINT ( 'NONE',  ( 4.287079134832745275, -79.44247393178839900, 9.901961492083930949 ) ) ;
#14923=CARTESIAN_POINT ( 'NONE',  ( 7.313768098873999257, -79.02375777975099425, 9.313141831727000053 ) ) ;
#14924=CARTESIAN_POINT ( 'NONE',  ( 0.000000000000000000, -87.59999999999999432, 0.000000000000000000 ) ) ;
#14926=ORIENTED_EDGE ( 'NONE', *, *, #53604, .F. ) ;
#14928=CARTESIAN_POINT ( 'NONE',  ( 11.93224739473999918, -77.87500106391100019, 0.2386934378577999782 ) ) ;
#14932=EDGE_CURVE ( 'NONE', #55147, #12394, #45285, .T. ) ;
#14940=CARTESIAN_POINT ( 'NONE',  ( 9.393203674808285442, -80.70833333333332860, -5.413904038987152667 ) ) ;
#14942=CARTESIAN_POINT ( 'NONE',  ( 3.630949683904999947, -79.79999999999999716, -11.17491406647000041 ) ) ;
#14944=CARTESIAN_POINT ( 'NONE',  ( -10.71797595155061877, -80.09332378991105372, 0.9698581247420646756 ) ) ;
#14948=CARTESIAN_POINT ( 'NONE',  ( -7.695020077040999773, -76.20149010202899831, 8.115451295621999961 ) ) ;
#14959=DIRECTION ( 'NONE',  ( -1.000000000000000000, 0.000000000000000000, 0.000000000000000000 ) ) ;
#14961=CARTESIAN_POINT ( 'NONE',  ( -9.797074649825203707, -78.06619525258034287, 4.439059621284440205 ) ) ;
#14979=CARTESIAN_POINT ( 'NONE',  ( -11.28597752728000003, -80.71071295308820481, -0.2623390868082999816 ) ) ;
#14982=CARTESIAN_POINT ( 'NONE',  ( -8.728447447808001414, -76.84899201919300538, 6.810956705545000212 ) ) ;
#14992=CARTESIAN_POINT ( 'NONE',  ( 7.496935112050000072, -80.51537353295650234, 8.408636027568000770 ) ) ;
#15001=CARTESIAN_POINT ( 'NONE',  ( 4.975516581814000361, -78.41739492409399759, -11.10075516933000017 ) ) ;
#15010=CARTESIAN_POINT ( 'NONE',  ( 1.407249749486563895, -77.73544497621409732, -10.74983756269776514 ) ) ;
#15021=CARTESIAN_POINT ( 'NONE',  ( -11.14643061761961818, -76.74479870980059104, 0.7341212784377569855 ) ) ;
#15033=CARTESIAN_POINT ( 'NONE',  ( 12.24159337356999977, -76.37751877473299089, -0.9828625608234000666 ) ) ;
#15034=B_SPLINE_CURVE_WITH_KNOTS ( 'NONE', 3,
 ( #5963, #38126, #6549, #45851, #24267, #41692, #54975, #55265, #51732, #23966, #1270, #14524, #33404, #41985, #19261, #56150, #37839, #42574 ),
 .UNSPECIFIED., .F., .F.,
 ( 4, 2, 2, 2, 2, 2, 2, 2, 4 ),
 ( 0.000000000000000000, 0.1250000000000000000, 0.2500000000000000000, 0.3750000000000000000, 0.5000000000000000000, 0.6250000000000000000, 0.7500000000000000000, 0.8750000000000000000, 1.000000000000000000 ),
 .UNSPECIFIED. ) ;
#15035=LINE ( 'NONE', #9741, #44974 ) ;
#15038=CARTESIAN_POINT ( 'NONE',  ( 0.000000000000000000, -75.15999999999999659, 0.000000000000000000 ) ) ;
#15047=CARTESIAN_POINT ( 'NONE',  ( 7.527227981725999939, -78.33017081663599868, 9.409389490551998136 ) ) ;
#15051=CARTESIAN_POINT ( 'NONE',  ( 6.695505957611000092, -79.34904856920998384, 8.622387486181999350 ) ) ;
#15055=CARTESIAN_POINT ( 'NONE',  ( -12.00019890019965096, -76.39977373798492977, -1.177339121803222359E-06 ) ) ;
#15056=CARTESIAN_POINT ( 'NONE',  ( 9.393203674808260573, -77.29166666666665719, 5.413904038987188194 ) ) ;
#15063=CARTESIAN_POINT ( 'NONE',  ( -10.07641688825555271, -76.38559964190847040, -4.852212949701282696 ) ) ;
#15064=CARTESIAN_POINT ( 'NONE',  ( -5.422116380438207983, -79.63706600996927421, -10.51876813104020059 ) ) ;
#15065=CARTESIAN_POINT ( 'NONE',  ( 9.599999999916001059, -90.40000000008399184, -6.531555804621000072E-10 ) ) ;
#15069=CARTESIAN_POINT ( 'NONE',  ( -9.066922875887595268, -78.90000278671779199, -6.603977477736625801 ) ) ;
#15079=CARTESIAN_POINT ( 'NONE',  ( 2.853743189566999534E-14, -82.05000000008600125, 0.000000000000000000 ) ) ;
#15080=CARTESIAN_POINT ( 'NONE',  ( 8.845698630191822787, -78.80205931604734815, -6.110774902956666033 ) ) ;
#15081=AXIS2_PLACEMENT_3D ( 'NONE', #53249, #12800, #58266 ) ;
#15088=CARTESIAN_POINT ( 'NONE',  ( 11.84749940521009393, -76.81854709368607814, 2.910134059890192582 ) ) ;
#15090=CARTESIAN_POINT ( 'NONE',  ( 11.88398914487867941, -78.28982288711439708, -1.513536703370712999 ) ) ;
#15091=CARTESIAN_POINT ( 'NONE',  ( 3.371435477143000181, -79.41539981197399811, -10.69820234502000034 ) ) ;
#15092=VERTEX_POINT ( 'NONE', #48615 ) ;
#15111=CARTESIAN_POINT ( 'NONE',  ( -0.3512719843520540897, -77.97766118670328694, 10.74453117849748374 ) ) ;
#15112=CARTESIAN_POINT ( 'NONE',  ( -9.690626710582000314, -78.11611985355399668, -7.043281791253000357 ) ) ;
#15120=CARTESIAN_POINT ( 'NONE',  ( 3.831242997621999713, -77.30563908551199859, 10.34520717408000046 ) ) ;
#15121=CARTESIAN_POINT ( 'NONE',  ( 11.13784153760999907, -76.43460365348362018, 5.174080857020999957 ) ) ;
#15122=CARTESIAN_POINT ( 'NONE',  ( -12.00000000000000000, -78.29999999999999716, 0.000000000000000000 ) ) ;
#15128=CARTESIAN_POINT ( 'NONE',  ( -8.728447447808001414, -76.71341491264000467, 6.810956705545000212 ) ) ;
#15133=CARTESIAN_POINT ( 'NONE',  ( -5.177348173361999706, -76.16656866488499134, -10.99455251688000068 ) ) ;
#15140=CARTESIAN_POINT ( 'NONE',  ( 2.988858019399999844, -77.42296592294499646, -10.85820852157999994 ) ) ;
#15149=ORIENTED_EDGE ( 'NONE', *, *, #17014, .F. ) ;
#15150=B_SPLINE_CURVE_WITH_KNOTS ( 'NONE', 3,
 ( #26259, #13559, #58143, #48999, #3829, #21829, #8259, #39834, #8546, #9146, #57555, #13263, #31253, #21254, #53136, #48715, #16837, #17710, #44272, #49295, #17116, #18003, #7969, #35993, #31551, #44865, #57847, #54018, #57273, #23, #25966, #43992, #12964, #21545, #22420, #35696, #49598, #34819, #35102, #30962, #27130, #45168, #52847, #39260, #17406, #12684, #26538, #39550, #12400, #3543, #44565, #4119, #22120, #40130, #53724, #8846, #26837, #4419, #22717, #50182, #19171, #10316, #15021, #33015, #19460 ),
 .UNSPECIFIED., .F., .F.,
 ( 4, 1, 1, 1, 1, 1, 1, 1, 1, 1, 1, 1, 1, 1, 1, 1, 1, 1, 1, 1, 1, 1, 1, 1, 1, 1, 1, 1, 1, 1, 1, 1, 1, 1, 1, 1, 1, 1, 1, 1, 1, 1, 1, 1, 1, 1, 1, 1, 1, 1, 1, 1, 1, 1, 1, 1, 1, 1, 1, 1, 1, 1, 4 ),
 ( 0.000000000000000000, 0.01249977652363656183, 0.02874978397244884118, 0.04499979142126112053, 0.06124979887007339641, 0.07749980631888567228, 0.09374981376769794816, 0.1099998212165102240, 0.1262498286653224999, 0.1424998361141347758, 0.1587498435629470794, 0.1749998510117593276, 0.1912498584605716312, 0.2074998659093838793, 0.2237498733581961829, 0.2399998808070084588, 0.2562498882558207347, 0.2724998957046330661, 0.2887499031534452865, 0.3049999106022575623, 0.3212499180510698382, 0.3374999254998821696, 0.3537499329486944455, 0.3699999403975066659, 0.3862499478463189417, 0.4024999552951312731, 0.4187499627439435490, 0.4349999701927558249, 0.4512499776415680453, 0.4674999850903803766, 0.4837499925391926525, 0.4999999999880049284, 0.5162500074368171488, 0.5325000148856294802, 0.5487500223344417005, 0.5650000297832540319, 0.5812500372320663633, 0.5975000446808785837, 0.6137500521296909151, 0.6300000595785031354, 0.6462500670273154668, 0.6625000744761276872, 0.6787500819249399076, 0.6950000893737522389, 0.7112500968225645703, 0.7275001042713769017, 0.7437501117201891221, 0.7600001191690013425, 0.7762501266178136738, 0.7925001340666258942, 0.8087501415154382256, 0.8250001489642504460, 0.8412501564130627774, 0.8575001638618751088, 0.8737501713106873291, 0.8900001787594996605, 0.9062501862083118809, 0.9225001936571242123, 0.9387502011059364326, 0.9550002085547486530, 0.9712502160035609844, 0.9875002234523733158, 1.000000000000000000 ),
 .UNSPECIFIED. ) ;
#15152=CARTESIAN_POINT ( 'NONE',  ( 8.591781367357000931, -78.69610392334999460, 7.101823234627000048 ) ) ;
#15154=ORIENTED_EDGE ( 'NONE', *, *, #23496, .T. ) ;
#15199=CARTESIAN_POINT ( 'NONE',  ( -9.799999999999998934, -92.13603921945998820, 1.133246274598000030E-12 ) ) ;
#15204=CARTESIAN_POINT ( 'NONE',  ( -2.513426006153157033, -79.49377681576562793, 10.45203454596306081 ) ) ;
#15213=CARTESIAN_POINT ( 'NONE',  ( -11.69999999991999928, -75.99999999992400035, -2.424604595008000056E-09 ) ) ;
#15216=CARTESIAN_POINT ( 'NONE',  ( 5.841136755832899929, -80.27119191073492743, -9.025644075688319390 ) ) ;
#15218=CARTESIAN_POINT ( 'NONE',  ( -7.595496139713672434, -77.16257047061313301, -7.607272242958681652 ) ) ;
#15223=VERTEX_POINT ( 'NONE', #53784 ) ;
#15224=CARTESIAN_POINT ( 'NONE',  ( -11.95950202284999975, -79.19309835455399593, 1.295167635372999948 ) ) ;
#15228=CARTESIAN_POINT ( 'NONE',  ( -6.752419751440000617, -78.20055284899699188, -9.840748444448999876 ) ) ;
#15236=ORIENTED_EDGE ( 'NONE', *, *, #15522, .T. ) ;
#15237=AXIS2_PLACEMENT_3D ( 'NONE', #31095, #451, #40271 ) ;
#15243=CARTESIAN_POINT ( 'NONE',  ( -0.8507363746134872784, -79.80000000000001137, -11.77153046305032902 ) ) ;
#15246=CARTESIAN_POINT ( 'NONE',  ( -10.07624512687999996, -76.23402931670899818, -4.852130239470000106 ) ) ;
#15249=B_SPLINE_CURVE_WITH_KNOTS ( 'NONE', 3,
 ( #18042, #22752, #31591, #45498, #49634, #9181, #27166, #5044, #23043, #41058, #36620, #23913, #33639, #11228, #15056, #46379, #15934, #42230 ),
 .UNSPECIFIED., .F., .F.,
 ( 4, 2, 2, 2, 2, 2, 2, 2, 4 ),
 ( 0.000000000000000000, 0.1250000000000000000, 0.2500000000000000000, 0.3750000000000000000, 0.5000000000000000000, 0.6250000000000000000, 0.7500000000000000000, 0.8750000000000000000, 1.000000000000000000 ),
 .UNSPECIFIED. ) ;
#15250=CARTESIAN_POINT ( 'NONE',  ( -10.71544265974000076, -76.80223585847799939, 2.915930582825000172 ) ) ;
#15260=CARTESIAN_POINT ( 'NONE',  ( 7.475611960616999951, -79.75467010736198858, -9.493926176044999110 ) ) ;
#15261=AXIS2_PLACEMENT_3D ( 'NONE', #36207, #23499, #50388 ) ;
#15262=CARTESIAN_POINT ( 'NONE',  ( 11.37395959471070483, -76.22187500001194849, 3.693278803254645748 ) ) ;
#15279=CARTESIAN_POINT ( 'NONE',  ( -3.071993112688999883, -80.60579489507729534, 10.86300919910000040 ) ) ;
#15282=CARTESIAN_POINT ( 'NONE',  ( -9.457500717944000712, -78.44685747529899800, -6.031068363571000290 ) ) ;
#15288=VERTEX_POINT ( 'NONE', #5925 ) ;
#15291=CARTESIAN_POINT ( 'NONE',  ( -8.418594644163000851, -80.75615502098555964, -7.485750452785000064 ) ) ;
#15300=CARTESIAN_POINT ( 'NONE',  ( 7.599120132820000428, -78.58017081663599868, 9.499258065358000991 ) ) ;
#15304=EDGE_LOOP ( 'NONE', ( #35395, #29957, #40225, #1457 ) ) ;
#15309=CARTESIAN_POINT ( 'NONE',  ( 9.393383141732488895, -77.80837651054207527, -5.413844486429424840 ) ) ;
#15313=CARTESIAN_POINT ( 'NONE',  ( -10.90022919700999893, -78.56903125995000892, 0.6003077901278000006 ) ) ;
#15328=CARTESIAN_POINT ( 'NONE',  ( 10.47020627418439531, -77.72916666666667140, -2.813789756862242974 ) ) ;
#15329=EDGE_CURVE ( 'NONE', #15756, #45004, #12293, .T. ) ;
#15334=CARTESIAN_POINT ( 'NONE',  ( -1.925872869407999843, -76.74636341947798712, -12.12904120624999926 ) ) ;
#15338=CARTESIAN_POINT ( 'NONE',  ( 10.54265532893000312, -78.52773149672268005, 3.830212845596999927 ) ) ;
#15346=CARTESIAN_POINT ( 'NONE',  ( -10.67791114319000023, -78.54720534002599663, -5.583725037239000599 ) ) ;
#15352=CARTESIAN_POINT ( 'NONE',  ( -10.58864275599752958, -79.58633413285787128, 1.856070104963200906 ) ) ;
#15362=FACE_OUTER_BOUND ( 'NONE', #36275, .T. ) ;
#15364=CARTESIAN_POINT ( 'NONE',  ( -11.08513710546999853, -79.26246662722100211, 1.988391287278999942 ) ) ;
#15366=CARTESIAN_POINT ( 'NONE',  ( 8.899186938124000079, -76.04999999999999716, -6.465637775218000094 ) ) ;
#15367=CARTESIAN_POINT ( 'NONE',  ( 11.83165817387121876, -79.30168238477698139, 0.2954418266251981340 ) ) ;
#15382=CARTESIAN_POINT ( 'NONE',  ( 9.994252366402587739, -78.82006649457892422, -3.959790582201482501 ) ) ;
#15389=CARTESIAN_POINT ( 'NONE',  ( -11.74114114509063533, -78.53398672592838636, 2.380251238623568799 ) ) ;
#15391=CARTESIAN_POINT ( 'NONE',  ( 5.622824352109999424, -80.06846743556140211, -9.705769245306999693 ) ) ;
#15397=CARTESIAN_POINT ( 'NONE',  ( -10.58742881249942869, -77.82311968649129597, 3.705126192729017109 ) ) ;
#15400=CIRCLE ( 'NONE', #45594, 9.700000000000001066 ) ;
#15413=CARTESIAN_POINT ( 'NONE',  ( 0.4922963458217056165, -77.97152273167989733, 10.74989978380444811 ) ) ;
#15414=CARTESIAN_POINT ( 'NONE',  ( 3.249499231398999655, -78.71296479287700265, -11.53069031867000049 ) ) ;
#15422=CARTESIAN_POINT ( 'NONE',  ( 10.83471462526000018, -77.22393005650599207, 2.076220934837999632 ) ) ;
#15423=CARTESIAN_POINT ( 'NONE',  ( 4.297951556683999641, -76.80344829822820429, -11.50435740523999861 ) ) ;
#15424=CARTESIAN_POINT ( 'NONE',  ( -6.043427764450786555, -78.38333333333332575, -10.48543666025110177 ) ) ;
#15429=CARTESIAN_POINT ( 'NONE',  ( -6.884807209879999057, -78.40630526502499720, -8.855368954042999619 ) ) ;
#15439=ADVANCED_FACE ( 'NONE', ( #26467 ), #31476, .T. ) ;
#15442=CARTESIAN_POINT ( 'NONE',  ( 11.23689443680000011, -77.53191129495199618, 0.7524413429202000403 ) ) ;
#15456=CARTESIAN_POINT ( 'NONE',  ( 10.47694508628999976, -78.66886758034799243, 3.806339902057000124 ) ) ;
#15469=CARTESIAN_POINT ( 'NONE',  ( 5.622824352109999424, -79.86510177573269686, -9.705769245306999693 ) ) ;
#15474=EDGE_CURVE ( 'NONE', #47432, #42525, #47566, .T. ) ;
#15479=CARTESIAN_POINT ( 'NONE',  ( -8.012523733904361123, -77.36708638852499575, -8.990154430768210858 ) ) ;
#15490=CARTESIAN_POINT ( 'NONE',  ( 0.000000000000000000, -92.13603921945998820, 0.000000000000000000 ) ) ;
#15493=CARTESIAN_POINT ( 'NONE',  ( -11.70000000000000107, -80.79999999999999716, 0.000000000000000000 ) ) ;
#15494=VERTEX_POINT ( 'NONE', #19095 ) ;
#15497=CARTESIAN_POINT ( 'NONE',  ( 0.000000000000000000, -81.00000000000000000, 0.000000000000000000 ) ) ;
#15501=CARTESIAN_POINT ( 'NONE',  ( -0.02668022986331678933, -79.47531791158665726, 10.74989935270009589 ) ) ;
#15514=CARTESIAN_POINT ( 'NONE',  ( 7.608898304480751662, -80.28757492195111922, -7.593877026215479553 ) ) ;
#15515=CARTESIAN_POINT ( 'NONE',  ( -10.75000000000000000, -77.10000000000000853, 0.000000000000000000 ) ) ;
#15517=ORIENTED_EDGE ( 'NONE', *, *, #57139, .T. ) ;
#15519=CARTESIAN_POINT ( 'NONE',  ( 11.43764105185000091, -79.83449565003729731, 2.691257544168000226 ) ) ;
#15522=EDGE_CURVE ( 'NONE', #8076, #8174, #33724, .T. ) ;
#15525=CARTESIAN_POINT ( 'NONE',  ( 11.76923221829999910, -77.38667338628398795, 1.980068107414000300 ) ) ;
#15529=ORIENTED_EDGE ( 'NONE', *, *, #11263, .F. ) ;
#15538=CARTESIAN_POINT ( 'NONE',  ( -10.44136617523937360, -79.79999999999998295, -5.814006440372521567 ) ) ;
#15541=CARTESIAN_POINT ( 'NONE',  ( -5.279550234765999939, -76.41977030724000031, -9.859017853534000508 ) ) ;
#15542=CARTESIAN_POINT ( 'NONE',  ( -10.07979664880000037, -76.57175206120300004, 3.736335038366999761 ) ) ;
#15545=CARTESIAN_POINT ( 'NONE',  ( -1.650172555132999985, -76.77799580226398746, 10.99074904627999949 ) ) ;
#15555=CARTESIAN_POINT ( 'NONE',  ( -11.20868100329999884, -79.54611832227699608, 4.514961651145999788 ) ) ;
#15557=CARTESIAN_POINT ( 'NONE',  ( 11.80338905328919985, -76.21406250001351168, 1.871110305591846101 ) ) ;
#15566=CARTESIAN_POINT ( 'NONE',  ( 10.75000000000000000, -77.25000000000000000, 0.000000000000000000 ) ) ;
#15571=ORIENTED_EDGE ( 'NONE', *, *, #44348, .F. ) ;
#15573=CARTESIAN_POINT ( 'NONE',  ( -6.997899816120000338, -80.78065832509547306, -8.858414569421000806 ) ) ;
#15577=CARTESIAN_POINT ( 'NONE',  ( 0.5473670387515998659, -77.03056763920500316, -11.20350390113000039 ) ) ;
#15594=CARTESIAN_POINT ( 'NONE',  ( 10.68616709762000028, -77.53559594867499527, -6.049920594266999352 ) ) ;
#15601=CARTESIAN_POINT ( 'NONE',  ( 10.75000000000000000, -77.85000000000000853, 0.000000000000000000 ) ) ;
#15605=CARTESIAN_POINT ( 'NONE',  ( -5.250095168255000111, -79.65848498002199563, -9.571408815458999797 ) ) ;
#15621=CARTESIAN_POINT ( 'NONE',  ( -11.80208112487999905, -77.08840224925098994, -3.396125071686999952 ) ) ;
#15625=CARTESIAN_POINT ( 'NONE',  ( -9.805641529082999241, -79.29034910077353970, -5.446788484474000214 ) ) ;
#15630=CARTESIAN_POINT ( 'NONE',  ( 3.113304451009999863, -78.39783470746900207, -10.55022916317000181 ) ) ;
#15633=CARTESIAN_POINT ( 'NONE',  ( -0.8050603620646999969, -78.56086622188500712, -12.13813858862000217 ) ) ;
#15637=CARTESIAN_POINT ( 'NONE',  ( 10.63911585229000067, -79.29457588320700268, 2.446340097336999975 ) ) ;
#15650=CARTESIAN_POINT ( 'NONE',  ( -7.438698978239999704, -79.34417565622699442, -8.455750828251000328 ) ) ;
#15652=CARTESIAN_POINT ( 'NONE',  ( -3.301984850800046001, -78.94713398100178381, 11.36385870249712582 ) ) ;
#15654=CARTESIAN_POINT ( 'NONE',  ( -9.599999999999999645, -92.13603921945998820, 0.000000000000000000 ) ) ;
#15659=CARTESIAN_POINT ( 'NONE',  ( 12.00000000000000000, -76.64999999999999147, 0.000000000000000000 ) ) ;
#15662=CARTESIAN_POINT ( 'NONE',  ( 2.787230247158716256, -78.45418832451430546, 10.40622211214603787 ) ) ;
#15666=CARTESIAN_POINT ( 'NONE',  ( -3.756378708322000382, -77.15821184318100734, 11.89142995536000136 ) ) ;
#15667=CARTESIAN_POINT ( 'NONE',  ( 4.118279509176275610, -78.75630550986022627, -9.929848109398376366 ) ) ;
#15678=CARTESIAN_POINT ( 'NONE',  ( -1.639962962630000076, -78.72057076119999408, 11.09633417262999977 ) ) ;
#15685=CARTESIAN_POINT ( 'NONE',  ( -9.998919412391977346, -77.38733819846200390, -5.083622679572695979 ) ) ;
#15687=EDGE_CURVE ( 'NONE', #2822, #35616, #36231, .T. ) ;
#15688=FACE_OUTER_BOUND ( 'NONE', #13897, .T. ) ;
#15695=CARTESIAN_POINT ( 'NONE',  ( 2.377756013412999803, -79.29083355210798345, -11.79209151100000064 ) ) ;
#15698=VERTEX_POINT ( 'NONE', #53699 ) ;
#15701=CARTESIAN_POINT ( 'NONE',  ( 2.813892236037239591, -79.24597810272209131, -10.47065658903501451 ) ) ;
#15702=CARTESIAN_POINT ( 'NONE',  ( -3.545645331619000196, -77.53280483666000578, 11.44309676683000099 ) ) ;
#15704=CARTESIAN_POINT ( 'NONE',  ( -5.413816992568016850, -79.01682948708119625, 9.393189368892933544 ) ) ;
#15706=CARTESIAN_POINT ( 'NONE',  ( 8.138661153347824140, -80.90697426621636623, 7.022889926100115865 ) ) ;
#15709=CARTESIAN_POINT ( 'NONE',  ( -11.03167625133000129, -77.95931131755500587, -0.06207630174703999970 ) ) ;
#15711=CARTESIAN_POINT ( 'NONE',  ( 10.74691056845999881, -80.79039695949025202, 1.883480763652999990 ) ) ;
#15717=CARTESIAN_POINT ( 'NONE',  ( -2.185791986076000004, -77.87549888071799842, -11.00183730042999919 ) ) ;
#15721=CARTESIAN_POINT ( 'NONE',  ( 3.242959734088999735, -77.22308533742300085, -11.71178937074000004 ) ) ;
#15731=DIRECTION ( 'NONE',  ( 0.000000000000000000, 0.000000000000000000, -1.000000000000000000 ) ) ;
#15744=B_SPLINE_CURVE_WITH_KNOTS ( 'NONE', 3,
 ( #2434, #20721, #38431, #29562, #2725, #38720, #30344, #22377, #53090, #3784, #44820, #17660, #48669, #58396, #31209, #17958, #35647, #53675 ),
 .UNSPECIFIED., .F., .F.,
 ( 4, 2, 2, 2, 2, 2, 2, 2, 4 ),
 ( 0.000000000000000000, 0.1250000000000000000, 0.2499999999999999722, 0.3750000000000000000, 0.5000000000000000000, 0.6250000000000000000, 0.7500000000000000000, 0.8750000000000000000, 1.000000000000000000 ),
 .UNSPECIFIED. ) ;
#15754=CARTESIAN_POINT ( 'NONE',  ( 2.407803015296000382, -80.05575617674540467, 10.73324203768999929 ) ) ;
#15755=EDGE_LOOP ( 'NONE', ( #4850, #2263, #10522, #13916 ) ) ;
#15756=VERTEX_POINT ( 'NONE', #22396 ) ;
#15762=CARTESIAN_POINT ( 'NONE',  ( 8.596418555780450887, -76.69791666666668561, -6.606377239730321982 ) ) ;
#15764=CARTESIAN_POINT ( 'NONE',  ( -7.223234266881707555, -77.37379502737748282, -9.635782272404652460 ) ) ;
#15773=CARTESIAN_POINT ( 'NONE',  ( 6.606800074109491661, -76.77723522011874024, -8.596815025920347964 ) ) ;
#15794=CARTESIAN_POINT ( 'NONE',  ( -0.003822974957334815405, -79.47514570661689959, 10.74992904790657455 ) ) ;
#15799=CARTESIAN_POINT ( 'NONE',  ( 8.993546968190999635, -77.34198448012199378, -6.388884668894999841 ) ) ;
#15805=CARTESIAN_POINT ( 'NONE',  ( 7.807646140253542200, -80.28969248854734531, -7.390132470684190658 ) ) ;
#15809=CARTESIAN_POINT ( 'NONE',  ( -7.858171174022000827, -79.06554253958299228, 9.108036400545000077 ) ) ;
#15814=CARTESIAN_POINT ( 'NONE',  ( -11.44451898095999987, -78.14629421814900923, -3.385038809382000302 ) ) ;
#15815=AXIS2_PLACEMENT_3D ( 'NONE', #14022, #13138, #32020 ) ;
#15830=CARTESIAN_POINT ( 'NONE',  ( -2.414913865112868763, -79.79999999999999716, -11.57229497112463612 ) ) ;
#15832=CARTESIAN_POINT ( 'NONE',  ( -10.58481073984209786, -80.08630942833664790, 1.876888235204818622 ) ) ;
#15835=CARTESIAN_POINT ( 'NONE',  ( -7.695020077040999773, -76.33706720858099004, 8.115451295621999961 ) ) ;
#15839=CARTESIAN_POINT ( 'NONE',  ( -9.770426151684000970, -76.35160278844999482, 5.297017541237999616 ) ) ;
#15846=CARTESIAN_POINT ( 'NONE',  ( -5.021054719342000539, -79.98639431301229763, 10.71058697011000049 ) ) ;
#15885=EDGE_LOOP ( 'NONE', ( #55678, #42696, #2366, #17588 ) ) ;
#15886=CARTESIAN_POINT ( 'NONE',  ( 12.09396573961999799, -77.56272526409898660, -2.128801122353999986 ) ) ;
#15895=CARTESIAN_POINT ( 'NONE',  ( 10.85828250482999913, -79.33164886400000171, 1.128302723381999995 ) ) ;
#15905=CARTESIAN_POINT ( 'NONE',  ( 10.18066396183999878, -78.44417834570113257, 6.314281093748000728 ) ) ;
#15906=CYLINDRICAL_SURFACE ( 'NONE', #39727, 10.75000000000000000 ) ;
#15913=CARTESIAN_POINT ( 'NONE',  ( -7.650089724727000551, -76.63759212789700825, -9.607224057717001386 ) ) ;
#15924=CARTESIAN_POINT ( 'NONE',  ( -7.733454931756999606, -78.37096101391799152, 9.390218602554998739 ) ) ;
#15929=CARTESIAN_POINT ( 'NONE',  ( 10.30613478042999986, -78.74984902316998614, -3.599856929194000354 ) ) ;
#15930=CARTESIAN_POINT ( 'NONE',  ( -10.55305693674421619, -79.58487289164341405, 2.047928793955265281 ) ) ;
#15934=CARTESIAN_POINT ( 'NONE',  ( 10.74999999999999645, -77.26041666666667140, 1.407171709420451666 ) ) ;
#15938=CARTESIAN_POINT ( 'NONE',  ( -12.00000000000000000, -77.89999999999999147, -2.795183092923000262E-14 ) ) ;
#15941=CARTESIAN_POINT ( 'NONE',  ( 2.188076007269000200, -78.63603073817900224, 11.04745617521000156 ) ) ;
#15942=CARTESIAN_POINT ( 'NONE',  ( -10.15970891481431515, -76.81842413191742480, 4.240029984634371196 ) ) ;
#15944=CARTESIAN_POINT ( 'NONE',  ( -11.10694245833507310, -79.07649623643344228, -3.897797401036807496 ) ) ;
#15951=CARTESIAN_POINT ( 'NONE',  ( 9.559505855103624938, -76.07072051956410519, -5.521514537851864191 ) ) ;
#15952=DIRECTION ( 'NONE',  ( 0.000000000000000000, 1.000000000000000000, 0.000000000000000000 ) ) ;
#15956=CARTESIAN_POINT ( 'NONE',  ( -6.169654037346999687, -76.24235318827498986, 10.97285421267000061 ) ) ;
#15957=CARTESIAN_POINT ( 'NONE',  ( 0.1192520569309659245, -78.72596489933566488, -10.74939088699284362 ) ) ;
#15965=CARTESIAN_POINT ( 'NONE',  ( -6.606081245964748661, -79.67294187189699528, -8.595967819608736349 ) ) ;
#15968=CARTESIAN_POINT ( 'NONE',  ( -6.324515969367999979, -78.91122516221300032, -9.263833350438000380 ) ) ;
#15976=AXIS2_PLACEMENT_3D ( 'NONE', #17230, #3942, #18124 ) ;
#15977=LINE ( 'NONE', #42559, #58331 ) ;
#15987=B_SPLINE_CURVE_WITH_KNOTS ( 'NONE', 3,
 ( #50959, #10510, #3390, #42970, #34374, #33795, #20242, #12527, #20530, #21386 ),
 .UNSPECIFIED., .F., .F.,
 ( 4, 2, 2, 2, 4 ),
 ( 0.000000000000000000, 0.2500000000000001110, 0.5000000000000001110, 0.7500000000000001110, 1.000000000000000000 ),
 .UNSPECIFIED. ) ;
#15994=CARTESIAN_POINT ( 'NONE',  ( -9.393470487601941699, -79.14183230196326235, -5.414092425894560634 ) ) ;
#15996=CARTESIAN_POINT ( 'NONE',  ( -6.777984382448000389, -78.07546061570199925, -9.878005474088999094 ) ) ;
#16000=CARTESIAN_POINT ( 'NONE',  ( 10.41713664689605245, -80.87023554807993264, 2.654027955184751431 ) ) ;
#16003=CARTESIAN_POINT ( 'NONE',  ( 8.061453700986000115, -77.76865691654299440, 7.530916186516999566 ) ) ;
#16004=CARTESIAN_POINT ( 'NONE',  ( 8.039723150245000838, -80.33398629742849550, 7.069263470143000383 ) ) ;
#16010=CARTESIAN_POINT ( 'NONE',  ( 1.407384697719938904, -80.46469927918771248, 10.68108411319174245 ) ) ;
#16011=CARTESIAN_POINT ( 'NONE',  ( 0.5473670387515998659, -76.89499053265299722, -11.20350390113000039 ) ) ;
#16043=CARTESIAN_POINT ( 'NONE',  ( -10.50414906643726987, -81.00000000000000000, -2.423834968728446615 ) ) ;
#16044=CARTESIAN_POINT ( 'NONE',  ( 7.307192483546000261, -76.75676689867499647, -8.110505779365999146 ) ) ;
#16054=FACE_OUTER_BOUND ( 'NONE', #20546, .T. ) ;
#16058=CARTESIAN_POINT ( 'NONE',  ( -5.413904038987160661, -76.58333333333330017, -9.393203674808278336 ) ) ;
#16059=CARTESIAN_POINT ( 'NONE',  ( -9.596002108778193929, -76.84791666666663446, 7.374560639698937159 ) ) ;
#16090=DIRECTION ( 'NONE',  ( -1.000000000000000000, 0.000000000000000000, 0.000000000000000000 ) ) ;
#16092=ADVANCED_FACE ( 'NONE', ( #55151 ), #53571, .F. ) ;
#16096=CARTESIAN_POINT ( 'NONE',  ( -9.149418163674001292, -76.68831224807900071, -6.163594735446999984 ) ) ;
#16102=CARTESIAN_POINT ( 'NONE',  ( 5.994180301456028204, -80.27253328818157740, -8.923361141312334155 ) ) ;
#16106=CARTESIAN_POINT ( 'NONE',  ( -0.9103933733443999587, -79.61728894252300393, -11.99492895764000089 ) ) ;
#16108=CARTESIAN_POINT ( 'NONE',  ( 10.16136252780999882, -79.60888520700200388, 4.855993836148999598 ) ) ;
#16109=ORIENTED_EDGE ( 'NONE', *, *, #38593, .F. ) ;
#16118=ORIENTED_EDGE ( 'NONE', *, *, #47396, .T. ) ;
#16125=CARTESIAN_POINT ( 'NONE',  ( -10.54604950822804454, -80.08464066063081077, 2.090755568749749216 ) ) ;
#16129=CARTESIAN_POINT ( 'NONE',  ( 7.778176538613999824, -76.58788662847199191, -8.035785801754000701 ) ) ;
#16132=CARTESIAN_POINT ( 'NONE',  ( -4.924589481749999997, -76.87080480866698906, 9.835153137904999454 ) ) ;
#16140=CARTESIAN_POINT ( 'NONE',  ( -9.963109346188520732, -78.06943961487655770, 4.037170563993010219 ) ) ;
#16147=CARTESIAN_POINT ( 'NONE',  ( -6.745911349169843696, -79.22231418035541139, 9.981325353439961745 ) ) ;
#16159=CARTESIAN_POINT ( 'NONE',  ( 7.496935112050000072, -80.56705559776401060, 8.408636027568000770 ) ) ;
#16166=CARTESIAN_POINT ( 'NONE',  ( 6.436424241555000592, -79.92391735373439587, 8.610165096135999008 ) ) ;
#16176=EDGE_LOOP ( 'NONE', ( #11742, #54875, #24003, #45381, #4263 ) ) ;
#16177=CARTESIAN_POINT ( 'NONE',  ( 8.821626479137000487, -79.00077142985099954, 8.208219718620000549 ) ) ;
#16179=ORIENTED_EDGE ( 'NONE', *, *, #57168, .T. ) ;
#16198=CARTESIAN_POINT ( 'NONE',  ( -3.201374924283697521, -80.74789697147706136, 10.74410602307857765 ) ) ;
#16199=CARTESIAN_POINT ( 'NONE',  ( -3.085175050843000477, -78.25427313773511173, -11.57574012064000435 ) ) ;
#16209=CARTESIAN_POINT ( 'NONE',  ( 12.00000000000000888, -78.03958333333333997, -1.570796326794872577 ) ) ;
#16210=ORIENTED_EDGE ( 'NONE', *, *, #38865, .F. ) ;
#16214=CARTESIAN_POINT ( 'NONE',  ( 11.99999999999999822, -78.65670863885249275, 1.011638905658234666 ) ) ;
#16216=CARTESIAN_POINT ( 'NONE',  ( 3.985687926398000069, -78.28957306764699808, 11.49333817212000142 ) ) ;
#16221=CARTESIAN_POINT ( 'NONE',  ( -10.22017084124837005, -79.57491545742729500, 3.338102352714737986 ) ) ;
#16224=CARTESIAN_POINT ( 'NONE',  ( 5.224348721355000613, -79.41921447277900370, -10.97639677120000101 ) ) ;
#16231=CARTESIAN_POINT ( 'NONE',  ( 12.00000000000000000, -78.14999999999999147, 0.000000000000000000 ) ) ;
#16236=CARTESIAN_POINT ( 'NONE',  ( 11.17338741157130322, -79.27293521690316425, -3.903988906372769296 ) ) ;
#16253=CARTESIAN_POINT ( 'NONE',  ( -12.46551533733999939, -76.25659160047199236, 0.3559871039980000429 ) ) ;
#16254=CARTESIAN_POINT ( 'NONE',  ( 5.898677060894324420, -78.77139060450180352, -8.987420904564112689 ) ) ;
#16261=CARTESIAN_POINT ( 'NONE',  ( -10.75037226435630267, -79.61044805530501378, -1.407100289909882118 ) ) ;
#16264=CARTESIAN_POINT ( 'NONE',  ( -8.982117338527000783, -79.78278813827100180, 6.718606902359000266 ) ) ;
#16273=AXIS2_PLACEMENT_3D ( 'NONE', #29263, #30128, #25425 ) ;
#16274=CARTESIAN_POINT ( 'NONE',  ( -9.524907056233788083, -77.30562916945632423, 5.924335788417241844 ) ) ;
#16276=DIRECTION ( 'NONE',  ( -1.000000000000000000, 0.000000000000000000, 0.000000000000000000 ) ) ;
#16277=CARTESIAN_POINT ( 'NONE',  ( 1.407171709420391936, -80.86458333333331439, 10.75000000000000178 ) ) ;
#16282=CARTESIAN_POINT ( 'NONE',  ( 10.75000000000000000, -79.35000000000000853, 0.000000000000000000 ) ) ;
#16287=DIRECTION ( 'NONE',  ( 0.000000000000000000, 1.000000000000000000, 0.000000000000000000 ) ) ;
#16292=CARTESIAN_POINT ( 'NONE',  ( 11.20799393363000007, -77.84482669931600185, 4.230477091134000389 ) ) ;
#16299=CARTESIAN_POINT ( 'NONE',  ( -10.62516247904072486, -76.58790361868092589, 1.636441214579218650 ) ) ;
#16300=CARTESIAN_POINT ( 'NONE',  ( -0.9257816722924000485, -78.40834718399401027, 10.87742130684000053 ) ) ;
#16311=CARTESIAN_POINT ( 'NONE',  ( 11.37390407689999883, -76.35523235640999928, 4.280169657041000164 ) ) ;
#16314=EDGE_LOOP ( 'NONE', ( #40350, #54490, #22645, #42104 ) ) ;
#16315=CARTESIAN_POINT ( 'NONE',  ( -8.329953570067999635, -79.76670276584599151, -7.407190701775999919 ) ) ;
#16321=FACE_OUTER_BOUND ( 'NONE', #33374, .T. ) ;
#16328=CIRCLE ( 'NONE', #23856, 0.2000000000000005107 ) ;
#16337=CARTESIAN_POINT ( 'NONE',  ( -7.753620043410437646, -81.00000000000002842, -7.606346643182852141 ) ) ;
#16339=CARTESIAN_POINT ( 'NONE',  ( 10.06402303786000196, -77.79174793274400201, -4.229752508564000202 ) ) ;
#16343=CARTESIAN_POINT ( 'NONE',  ( 8.203824050184531202, -76.29609375003914806, -7.004042987541993170 ) ) ;
#16344=EDGE_LOOP ( 'NONE', ( #36208, #21694, #44775, #55376 ) ) ;
#16352=CARTESIAN_POINT ( 'NONE',  ( -10.75000000000000000, -76.51041666666665719, -1.407171709420429018 ) ) ;
#16358=CARTESIAN_POINT ( 'NONE',  ( -3.085175050843000477, -78.30595559095398528, -11.57574012064000080 ) ) ;
#16364=CARTESIAN_POINT ( 'NONE',  ( -10.21813353151999948, -76.78887615466000227, 4.735332084273999875 ) ) ;
#16381=CARTESIAN_POINT ( 'NONE',  ( -2.295071999339000079, -77.60036594554799194, 10.90812747857000176 ) ) ;
#16382=EDGE_CURVE ( 'NONE', #24385, #10331, #10849, .T. ) ;
#16388=CARTESIAN_POINT ( 'NONE',  ( 6.639710140890153767, -80.27824733682197689, -8.457367011817090940 ) ) ;
#16389=CARTESIAN_POINT ( 'NONE',  ( 10.27001848845763021, -79.87467406915122581, 3.283795101429460850 ) ) ;
#16391=CARTESIAN_POINT ( 'NONE',  ( -10.65106809510000119, -78.95984906387799640, 5.591232889670999739 ) ) ;
#16407=ORIENTED_EDGE ( 'NONE', *, *, #28903, .T. ) ;
#16413=CARTESIAN_POINT ( 'NONE',  ( 9.964806208336344895, -79.79999999999999716, 6.397882358273444758 ) ) ;
#16415=CARTESIAN_POINT ( 'NONE',  ( -6.940450258154920782, -80.03122518745470870, 8.209008405819576026 ) ) ;
#16419=CARTESIAN_POINT ( 'NONE',  ( 10.97835188747000146, -76.06862311939200083, -2.133021021907000048 ) ) ;
#16422=CARTESIAN_POINT ( 'NONE',  ( 8.280908091976000307, -76.08406207389899123, -7.227859519978000691 ) ) ;
#16426=DIRECTION ( 'NONE',  ( -1.000000000000000000, 0.000000000000000000, 0.000000000000000000 ) ) ;
#16429=CARTESIAN_POINT ( 'NONE',  ( -4.484732399288205329, -78.00924820851443542, 9.770240355338039251 ) ) ;
#16446=CARTESIAN_POINT ( 'NONE',  ( 1.328862289696999932, -80.11559030770953882, 11.18676134159000135 ) ) ;
#16454=CARTESIAN_POINT ( 'NONE',  ( 2.194504958346340739, -79.95907396938338252, 10.52387239888080828 ) ) ;
#16457=CARTESIAN_POINT ( 'NONE',  ( 8.660139315840918783, -77.29964975416137918, -6.376535095569426659 ) ) ;
#16465=CARTESIAN_POINT ( 'NONE',  ( 1.644133925033999910, -79.05503006069899641, 11.70364056775000172 ) ) ;
#16467=ORIENTED_EDGE ( 'NONE', *, *, #3026, .T. ) ;
#16502=CARTESIAN_POINT ( 'NONE',  ( -9.840265838668001308, -77.99115059798600669, -7.152041583326999685 ) ) ;
#16506=CARTESIAN_POINT ( 'NONE',  ( 10.75000000000000000, -80.34999999999999432, 0.000000000000000000 ) ) ;
#16508=CARTESIAN_POINT ( 'NONE',  ( -10.71852045160081168, -79.59351931985985118, 0.8923418771536563154 ) ) ;
#16509=EDGE_LOOP ( 'NONE', ( #7957, #31040, #48631, #41663, #47499, #29517 ) ) ;
#16510=CARTESIAN_POINT ( 'NONE',  ( -11.85739648576925553, -78.88587530551917837, 2.129864859879341932 ) ) ;
#16511=CARTESIAN_POINT ( 'NONE',  ( -2.849897923499999930, -79.08515109989099301, 11.69915687793999837 ) ) ;
#16524=CARTESIAN_POINT ( 'NONE',  ( 5.633582509268093119, -78.88484845060878570, 10.33564305875573730 ) ) ;
#16532=CARTESIAN_POINT ( 'NONE',  ( -11.59999999999999964, -87.70000000000000284, 0.000000000000000000 ) ) ;
#16534=CARTESIAN_POINT ( 'NONE',  ( 0.7035754441837855921, -78.46981644582842819, 10.74957883124878499 ) ) ;
#16538=CARTESIAN_POINT ( 'NONE',  ( -9.212468050143000298, -77.26692164589900358, 8.579241990457999734 ) ) ;
#16539=CARTESIAN_POINT ( 'NONE',  ( 4.117740896665462280, -78.75630124736080973, -9.930072027249686073 ) ) ;
#16547=CARTESIAN_POINT ( 'NONE',  ( 10.75000000000000000, -78.75000000000000000, 0.000000000000000000 ) ) ;
#16549=CARTESIAN_POINT ( 'NONE',  ( -10.75729140709000120, -78.92454102948499894, -3.177859684493999914 ) ) ;
#16553=ORIENTED_EDGE ( 'NONE', *, *, #45383, .F. ) ;
#16560=CARTESIAN_POINT ( 'NONE',  ( -10.75000000000000000, -78.00000000000000000, 2.252154972635999871E-14 ) ) ;
#16569=CARTESIAN_POINT ( 'NONE',  ( 0.000000000000000000, -90.35000000009100063, 0.000000000000000000 ) ) ;
#16574=CARTESIAN_POINT ( 'NONE',  ( 9.148490208346998998, -77.87195601473999318, 7.734416031130999514 ) ) ;
#16580=CARTESIAN_POINT ( 'NONE',  ( -10.64192559734432031, -76.58874692010783747, 1.522398744522916125 ) ) ;
#16586=CARTESIAN_POINT ( 'NONE',  ( 1.173088849732999872, -79.19397159786899465, 12.21509120978000063 ) ) ;
#16590=CARTESIAN_POINT ( 'NONE',  ( -2.309466437479000156, -77.72539668997998774, 10.97654204954999990 ) ) ;
#16594=CARTESIAN_POINT ( 'NONE',  ( -2.601777299206000205, -76.33297644249898894, 12.11064771572999987 ) ) ;
#16597=EDGE_LOOP ( 'NONE', ( #305, #55136, #29590, #41162 ) ) ;
#16598=CARTESIAN_POINT ( 'NONE',  ( 8.589798209762999903, -78.33715855134300909, -6.922213596449000583 ) ) ;
#16607=EDGE_CURVE ( 'NONE', #40109, #15092, #15744, .T. ) ;
#16616=ORIENTED_EDGE ( 'NONE', *, *, #46750, .F. ) ;
#16625=CARTESIAN_POINT ( 'NONE',  ( -11.20683111097000051, -79.70168371772200544, -0.4743912329535999728 ) ) ;
#16636=CARTESIAN_POINT ( 'NONE',  ( -1.407171709420418138, -76.61458333333330017, -10.75000000000000000 ) ) ;
#16642=ADVANCED_FACE ( 'NONE', ( #25771 ), #16781, .F. ) ;
#16643=CARTESIAN_POINT ( 'NONE',  ( -3.189212937810000259, -76.47126873785200019, 10.79536088457000176 ) ) ;
#16644=CARTESIAN_POINT ( 'NONE',  ( 11.20799393363000007, -77.98040380586900255, 4.230477091134000389 ) ) ;
#16646=VECTOR ( 'NONE', #34208, 1000.000000000000000 ) ;
#16650=( LENGTH_UNIT ( ) NAMED_UNIT ( * ) SI_UNIT ( .MILLI., .METRE. ) );
#16652=CARTESIAN_POINT ( 'NONE',  ( -7.880862184694999328, -76.76163981165899486, 7.737503720428000165 ) ) ;
#16663=CARTESIAN_POINT ( 'NONE',  ( -10.93308570624999909, -78.21625547246898691, -2.507139558745000052 ) ) ;
#16673=CARTESIAN_POINT ( 'NONE',  ( -5.715586620248999772, -77.79102034656098397, -9.570092484259999921 ) ) ;
#16679=CARTESIAN_POINT ( 'NONE',  ( 2.419489426094433515, -80.24335428146707727, -10.47420677764779029 ) ) ;
#16682=CARTESIAN_POINT ( 'NONE',  ( 11.77452260639999970, -79.75674588647899554, 1.259536412044000020 ) ) ;
#16684=CARTESIAN_POINT ( 'NONE',  ( 10.94267788024999888, -79.55441252099899430, -2.663036869319000299 ) ) ;
#16705=CARTESIAN_POINT ( 'NONE',  ( -10.21718853249328518, -80.07487106893638895, 3.342320372008775742 ) ) ;
#16708=CARTESIAN_POINT ( 'NONE',  ( -4.800187936532999800, -76.24419671331600057, 10.10109298474000106 ) ) ;
#16711=CARTESIAN_POINT ( 'NONE',  ( 10.83817488108000227, -76.69523121474300353, -1.875052409207000004 ) ) ;
#16723=CARTESIAN_POINT ( 'NONE',  ( -1.812920252538464227, -79.18700244415332179, 11.90997463893260644 ) ) ;
#16731=DIRECTION ( 'NONE',  ( 0.000000000000000000, -0.7071067811866525998, -0.7071067811864425456 ) ) ;
#16745=CARTESIAN_POINT ( 'NONE',  ( 10.34512087479159526, -77.32797947898937707, -2.955462300682764276 ) ) ;
#16755=B_SPLINE_CURVE_WITH_KNOTS ( 'NONE', 3,
 ( #31412, #13708, #52997, #48578, #49151, #57422, #22273, #31703, #183, #34966 ),
 .UNSPECIFIED., .F., .F.,
 ( 4, 2, 2, 2, 4 ),
 ( 0.000000000000000000, 0.2500000000000000000, 0.5000000000000001110, 0.7500000000000001110, 1.000000000000000000 ),
 .UNSPECIFIED. ) ;
#16756=CARTESIAN_POINT ( 'NONE',  ( -8.196454039252000001, -78.75660759103701025, -8.832548491656998735 ) ) ;
#16758=ORIENTED_EDGE ( 'NONE', *, *, #11850, .T. ) ;
#16767=ORIENTED_EDGE ( 'NONE', *, *, #45244, .F. ) ;
#16775=CARTESIAN_POINT ( 'NONE',  ( -11.74098051674999965, -78.63408355366797764, 2.380218674853999961 ) ) ;
#16781=CONICAL_SURFACE ( 'NONE', #49800, 9.649999999844000698, 0.7853981633972997312 ) ;
#16783=CARTESIAN_POINT ( 'NONE',  ( 12.24159337356999977, -76.24194166818098495, -0.9828625608234000666 ) ) ;
#16793=CARTESIAN_POINT ( 'NONE',  ( 11.71313121114000033, -78.66938348357999189, -3.284064838691000077 ) ) ;
#16798=CARTESIAN_POINT ( 'NONE',  ( -8.925400722459096770, -79.55299714917772747, 5.991630607438681366 ) ) ;
#16801=CARTESIAN_POINT ( 'NONE',  ( 11.95103999880999979, -79.43138830090799729, -1.471358499936000097 ) ) ;
#16804=CARTESIAN_POINT ( 'NONE',  ( -9.599999999916001059, -87.30000000008399752, 6.531558194539000517E-10 ) ) ;
#16829=CARTESIAN_POINT ( 'NONE',  ( 9.552063159248998403, -76.95329815165599996, -8.017142583401000167 ) ) ;
#16830=CARTESIAN_POINT ( 'NONE',  ( 2.679031828523773306, -78.74517864561535418, -10.41213411323704463 ) ) ;
#16837=CARTESIAN_POINT ( 'NONE',  ( 11.19952915612999789, -77.99557525653385426, -0.6234238306063999424 ) ) ;
#16840=ADVANCED_FACE ( 'NONE', ( #1543 ), #54395, .F. ) ;
#16843=ORIENTED_EDGE ( 'NONE', *, *, #2878, .F. ) ;
#16857=CARTESIAN_POINT ( 'NONE',  ( -2.813789756862251856, -79.60416666666667140, -10.47020627418439709 ) ) ;
#16864=CARTESIAN_POINT ( 'NONE',  ( -11.61454496413000115, -77.54640422965499624, 2.935712811417999557 ) ) ;
#16878=CARTESIAN_POINT ( 'NONE',  ( -5.709495105464999831, -79.91307963075219334, -10.86213658064000143 ) ) ;
#16881=CARTESIAN_POINT ( 'NONE',  ( -5.859445663532000914, -77.75263303298099515, 9.564779511708000115 ) ) ;
#16884=CARTESIAN_POINT ( 'NONE',  ( -6.650186219591999404, -76.86123477876799370, 10.45045725565999994 ) ) ;
#16888=CARTESIAN_POINT ( 'NONE',  ( 5.948804865077000237, -80.03906619586439319, 9.426875752653000262 ) ) ;
#16895=CARTESIAN_POINT ( 'NONE',  ( 3.030935459916999974, -79.18144108438299611, 11.73679554811000081 ) ) ;
#16908=CARTESIAN_POINT ( 'NONE',  ( -10.34074641381923065, -80.99999999999998579, -3.089209180937224630 ) ) ;
#16909=CARTESIAN_POINT ( 'NONE',  ( 5.013494814495999208, -77.41043913071800375, 9.697434492446999954 ) ) ;
#16914=CARTESIAN_POINT ( 'NONE',  ( -11.06493808903000087, -79.21142954368899325, -1.839906431680000010 ) ) ;
#16929=CARTESIAN_POINT ( 'NONE',  ( 12.08450773144999957, -79.26983947277899745, 1.677439557700999950 ) ) ;
#16931=CARTESIAN_POINT ( 'NONE',  ( 11.95248949435000085, -78.95705916112399336, 0.8087524912306001124 ) ) ;
#16939=CARTESIAN_POINT ( 'NONE',  ( 0.2638252682410999750, -78.51802014218399961, -11.14383981435000059 ) ) ;
#16947=CARTESIAN_POINT ( 'NONE',  ( -10.05535668103000191, -78.16178278646499678, 4.970705447719999448 ) ) ;
#16957=CARTESIAN_POINT ( 'NONE',  ( -11.14677829112999952, -77.70931131755500587, -0.06272399197938000048 ) ) ;
#16963=CARTESIAN_POINT ( 'NONE',  ( -2.085031794558877660, -80.20968772933238711, -10.54572087693944837 ) ) ;
#16965=CARTESIAN_POINT ( 'NONE',  ( 11.15695051371543833, -79.60814770476476099, 1.159337827475353189 ) ) ;
#16966=CARTESIAN_POINT ( 'NONE',  ( -12.02912753549999891, -79.56554297241000029, 0.08506824670321999626 ) ) ;
#16967=EDGE_CURVE ( 'NONE', #31041, #5144, #55163, .T. ) ;
#16969=CARTESIAN_POINT ( 'NONE',  ( 3.646964122112999807, -80.17176962903970150, 10.50067842184000000 ) ) ;
#16979=CARTESIAN_POINT ( 'NONE',  ( 5.708176239699000121, -78.24219514392800079, -9.305495801267001710 ) ) ;
#16987=ORIENTED_EDGE ( 'NONE', *, *, #4965, .T. ) ;
#16988=VERTEX_POINT ( 'NONE', #20411 ) ;
#16990=CARTESIAN_POINT ( 'NONE',  ( -1.887341892627375062, -79.79999999999998295, 11.86718873371815519 ) ) ;
#16991=CARTESIAN_POINT ( 'NONE',  ( -6.927833380277669484, -80.03110721467722044, 8.219656879950077766 ) ) ;
#16992=AXIS2_PLACEMENT_3D ( 'NONE', #28845, #10874, #42740 ) ;
#16998=CARTESIAN_POINT ( 'NONE',  ( 5.292034929522999143, -76.29392014291700264, 9.642417924923000427 ) ) ;
#17001=DIRECTION ( 'NONE',  ( 0.000000000000000000, -1.000000000000000000, 0.000000000000000000 ) ) ;
#17009=CARTESIAN_POINT ( 'NONE',  ( -12.00000000000000711, -79.29293765275959061, 1.064976873965741921 ) ) ;
#17011=CIRCLE ( 'NONE', #55705, 9.760776772971999193 ) ;
#17014=EDGE_CURVE ( 'NONE', #47018, #17785, #15977, .T. ) ;
#17018=ORIENTED_EDGE ( 'NONE', *, *, #31581, .F. ) ;
#17022=CARTESIAN_POINT ( 'NONE',  ( 12.00000000000000000, -79.14999999999999147, 0.000000000000000000 ) ) ;
#17025=CARTESIAN_POINT ( 'NONE',  ( 1.830902252650064010, -79.96174285384452673, 10.59271595565334678 ) ) ;
#17028=CARTESIAN_POINT ( 'NONE',  ( 10.75000000000000000, -77.35000000000000853, 0.000000000000000000 ) ) ;
#17037=EDGE_CURVE ( 'NONE', #8440, #45906, #12188, .T. ) ;
#17038=CARTESIAN_POINT ( 'NONE',  ( 1.747513281931999840, -77.39552404313198508, -11.88039736288000014 ) ) ;
#17045=EDGE_CURVE ( 'NONE', #38125, #56550, #37593, .T. ) ;
#17063=CARTESIAN_POINT ( 'NONE',  ( -1.984586691443999795, -75.88675793620500087, 11.75553522549000007 ) ) ;
#17072=CARTESIAN_POINT ( 'NONE',  ( 3.030935459916999974, -78.72825989114500089, 11.73679554811000081 ) ) ;
#17077=CARTESIAN_POINT ( 'NONE',  ( -6.271985153401672619, -79.52459541282148336, 8.730686292822458228 ) ) ;
#17081=CARTESIAN_POINT ( 'NONE',  ( -6.597056085936999992, -79.17951179515100080, 10.21048365676999836 ) ) ;
#17106=CARTESIAN_POINT ( 'NONE',  ( 6.764901149608999908, -77.36370303413399085, -9.901050649137001614 ) ) ;
#17108=CARTESIAN_POINT ( 'NONE',  ( 0.000000000000000000, -75.15999999999999659, 0.000000000000000000 ) ) ;
#17116=CARTESIAN_POINT ( 'NONE',  ( 1.633411169670999863, -77.88662988452688296, -11.09730050697999992 ) ) ;
#17119=CARTESIAN_POINT ( 'NONE',  ( -5.268979267983999293, -78.81559565747798501, 9.902321347348999936 ) ) ;
#17123=ORIENTED_EDGE ( 'NONE', *, *, #14195, .F. ) ;
#17128=CARTESIAN_POINT ( 'NONE',  ( 11.08610830971117522, -77.08773842544198374, -1.708745595551396157 ) ) ;
#17138=CARTESIAN_POINT ( 'NONE',  ( -7.858171174022000827, -79.08164813617541711, 9.108036400545000077 ) ) ;
#17144=CARTESIAN_POINT ( 'NONE',  ( 10.69384760718000038, -78.21110719282100376, -5.399785902169999652 ) ) ;
#17147=CARTESIAN_POINT ( 'NONE',  ( -11.79984144923200340, -76.38290029571203377, 2.513141340760493669 ) ) ;
#17158=B_SPLINE_CURVE_WITH_KNOTS ( 'NONE', 3,
 ( #34264, #38123, #12134, #7702, #33399, #43731, #29546, #25127, #51727, #3283, #21276, #47015, #6833, #24844, #2133, #20136, #38415, #56146, #11279, #15695, #29257, #42859, #56434, #20705, #32375, #44012, #17138, #8566, #30981, #49020, #57574, #22140 ),
 .UNSPECIFIED., .F., .F.,
 ( 4, 1, 1, 1, 1, 1, 1, 1, 1, 1, 1, 1, 1, 1, 1, 1, 1, 1, 1, 1, 1, 1, 1, 1, 1, 1, 1, 1, 1, 4 ),
 ( 0.000000000000000000, 0.001396860765158759038, 0.03786267284115284182, 0.07432848491735072338, 0.1107942969933448096, 0.1472601090695426773, 0.1837259211455369856, 0.2201917332217348533, 0.2566575452977291616, 0.2931233573739268072, 0.3295891694499208935, 0.3660549815259152018, 0.4025207936021130695, 0.4389866056781073778, 0.4754524177543050234, 0.5119182298302993317, 0.5483840419064972549, 0.5848498539824913411, 0.6213156660586891533, 0.6577814781346832396, 0.6942472902108811628, 0.7307131022868754711, 0.7671789143630732832, 0.8036447264390675915, 0.8401105385152655147, 0.8765763505912593789, 0.9130421626674571911, 0.9495079747434516104, 0.9859737868196494226, 1.000000000000000000 ),
 .UNSPECIFIED. ) ;
#17161=CARTESIAN_POINT ( 'NONE',  ( -1.051549137210000096, -76.55937287232799804, -12.34225577480999902 ) ) ;
#17165=CARTESIAN_POINT ( 'NONE',  ( -8.926133614190998600, -79.65775739383899179, 6.676731181684000482 ) ) ;
#17168=B_SPLINE_CURVE_WITH_KNOTS ( 'NONE', 3,
 ( #58317, #17879, #13430, #54188, #13726, #31723, #30562, #14887, #5744, #19045, #37036, #23460, #55050, #23752, #41473, #32592, #45631, #37618 ),
 .UNSPECIFIED., .F., .F.,
 ( 4, 2, 2, 2, 2, 2, 2, 2, 4 ),
 ( 0.000000000000000000, 0.1249999999999999722, 0.2499999999999999445, 0.3749999999999998890, 0.4999999999999998890, 0.6249999999999998890, 0.7499999999999997780, 0.8749999999999998890, 1.000000000000000000 ),
 .UNSPECIFIED. ) ;
#17170=CARTESIAN_POINT ( 'NONE',  ( 1.125737367536490563, -76.36666666666664582, 10.74999999999998757 ) ) ;
#17173=CARTESIAN_POINT ( 'NONE',  ( 2.284509925729999669, -78.18669951884498914, 12.06552085823000020 ) ) ;
#17176=CARTESIAN_POINT ( 'NONE',  ( 0.000000000000000000, -82.00000000000000000, 0.000000000000000000 ) ) ;
#17180=CARTESIAN_POINT ( 'NONE',  ( 10.74994633437535541, -78.84663129478072108, -0.4671562791492399058 ) ) ;
#17184=CARTESIAN_POINT ( 'NONE',  ( -3.427405331535606781, -81.00000000000000000, -10.36637788387490922 ) ) ;
#17185=CARTESIAN_POINT ( 'NONE',  ( -9.889498855898999352, -78.10460208417299555, 4.888716273084000363 ) ) ;
#17189=CARTESIAN_POINT ( 'NONE',  ( -10.39759693597000023, -79.79670861399999637, -4.208097972746998927 ) ) ;
#17197=EDGE_CURVE ( 'NONE', #47139, #54085, #29085, .T. ) ;
#17205=ORIENTED_EDGE ( 'NONE', *, *, #5130, .F. ) ;
#17206=CARTESIAN_POINT ( 'NONE',  ( 11.20573829663000076, -79.79121893549199740, 4.825001155745000325 ) ) ;
#17208=CARTESIAN_POINT ( 'NONE',  ( -1.360213228908000005, -77.81762791332599249, -11.90234785270000017 ) ) ;
#17214=LINE ( 'NONE', #30498, #26698 ) ;
#17215=CARTESIAN_POINT ( 'NONE',  ( -9.398554024959999253, -78.43631111317900206, -5.993477931829000127 ) ) ;
#17219=CARTESIAN_POINT ( 'NONE',  ( 3.113304451009999863, -78.39783470746900207, -10.55022916317000181 ) ) ;
#17224=CARTESIAN_POINT ( 'NONE',  ( -6.884807209879999057, -78.27072815847299125, -8.855368954042999619 ) ) ;
#17230=CARTESIAN_POINT ( 'NONE',  ( 2.854661674668000058E-14, -82.00000000000000000, 0.000000000000000000 ) ) ;
#17235=CARTESIAN_POINT ( 'NONE',  ( -11.18527010467000160, -78.26729255600099577, 1.312896411821999898 ) ) ;
#17241=CARTESIAN_POINT ( 'NONE',  ( 3.041187196987005681, -80.24796802560094022, -10.31335799952287502 ) ) ;
#17247=CARTESIAN_POINT ( 'NONE',  ( -3.970056213021999625, -78.90008180218299572, 11.35542513096999961 ) ) ;
#17248=CARTESIAN_POINT ( 'NONE',  ( 5.645478026989999343, -79.99019400902760424, -9.744872608167998607 ) ) ;
#17249=CARTESIAN_POINT ( 'NONE',  ( -9.392738704232332481, -77.55834533578540402, 5.413616812572119130 ) ) ;
#17254=ORIENTED_EDGE ( 'NONE', *, *, #17538, .F. ) ;
#17255=DIRECTION ( 'NONE',  ( -1.000000000000000000, 0.000000000000000000, 0.000000000000000000 ) ) ;
#17257=CARTESIAN_POINT ( 'NONE',  ( 3.413317904202999742, -78.92310371897299603, 10.36940822202999790 ) ) ;
#17258=CARTESIAN_POINT ( 'NONE',  ( -6.043427764450786555, -76.38333333329933339, -10.48543666025110177 ) ) ;
#17276=CARTESIAN_POINT ( 'NONE',  ( 7.936766385091000409, -76.33656526534099385, 7.448366782227999749 ) ) ;
#17284=CARTESIAN_POINT ( 'NONE',  ( -0.8698067890798458768, -80.98156680119757311, 10.71467698395598767 ) ) ;
#17285=CARTESIAN_POINT ( 'NONE',  ( 1.618170588614999961, -80.47036452348720559, -11.14857479085000058 ) ) ;
#17291=EDGE_CURVE ( 'NONE', #29449, #185, #2719, .T. ) ;
#17301=CARTESIAN_POINT ( 'NONE',  ( -4.454457568640999732, -80.65734865577489643, 10.34731867136000005 ) ) ;
#17308=CARTESIAN_POINT ( 'NONE',  ( 1.773208520488963824, -79.96215963365355606, 10.60254057701149577 ) ) ;
#17311=CARTESIAN_POINT ( 'NONE',  ( -4.643650396336004960, -77.18947228263908755, -9.695312717224595644 ) ) ;
#17321=CARTESIAN_POINT ( 'NONE',  ( -7.278283919121999901, -77.68490340765200131, 9.747261860606000639 ) ) ;
#17336=CARTESIAN_POINT ( 'NONE',  ( -1.814796094202807186, -80.23779093740807866, 11.06304992301285672 ) ) ;
#17338=CARTESIAN_POINT ( 'NONE',  ( -1.360213228908000227, -77.76594546010713316, -11.90234785270000195 ) ) ;
#17346=B_SPLINE_CURVE_WITH_KNOTS ( 'NONE', 3,
 ( #9933, #4630, #27912, #58353, #45962, #17915, #31760, #31166, #35604, #22032 ),
 .UNSPECIFIED., .F., .F.,
 ( 4, 2, 2, 2, 4 ),
 ( 0.5000000051225159670, 0.6250000038418869197, 0.7500000025612578725, 0.8750000012806289362, 1.000000000000000000 ),
 .UNSPECIFIED. ) ;
#17360=CARTESIAN_POINT ( 'NONE',  ( -10.87089293717000160, -77.01929369090099442, 0.9996073426339999735 ) ) ;
#17361=CARTESIAN_POINT ( 'NONE',  ( 6.544501642745999881, -77.61134018205299867, -10.25436633016999899 ) ) ;
#17366=CARTESIAN_POINT ( 'NONE',  ( -3.728013830608571055, -79.50331027668923412, 10.08280175580265059 ) ) ;
#17369=CARTESIAN_POINT ( 'NONE',  ( -11.50904265702000018, -79.23277905684599887, 3.913699539746000156 ) ) ;
#17370=CARTESIAN_POINT ( 'NONE',  ( -7.325508896758000432, -80.57304051666800149, 8.435678689013998977 ) ) ;
#17372=CARTESIAN_POINT ( 'NONE',  ( 0.9463392500275673580, -79.76874999999999716, 11.99969609698326778 ) ) ;
#17395=ORIENTED_EDGE ( 'NONE', *, *, #54871, .T. ) ;
#17396=CARTESIAN_POINT ( 'NONE',  ( 9.461695017160998589, -76.88557108724299383, -7.941295693778001485 ) ) ;
#17406=CARTESIAN_POINT ( 'NONE',  ( -10.96060824219999930, -77.23295765248289513, 2.383941600041999731 ) ) ;
#17409=CARTESIAN_POINT ( 'NONE',  ( -11.04065564778000130, -79.38755886051600896, 1.980412446595999798 ) ) ;
#17424=CARTESIAN_POINT ( 'NONE',  ( -10.71602610194999805, -79.72613058880257597, 3.314346869870000489 ) ) ;
#17429=EDGE_CURVE ( 'NONE', #47573, #53816, #56590, .T. ) ;
#17433=CARTESIAN_POINT ( 'NONE',  ( -1.360213228908000005, -77.61426225349798358, -11.90234785270000017 ) ) ;
#17436=CARTESIAN_POINT ( 'NONE',  ( 9.113984702984998520, -77.88244088799798703, 7.705244011730999709 ) ) ;
#17444=CARTESIAN_POINT ( 'NONE',  ( 2.262521961001000115, -79.96634689244729088, -12.06088927786000120 ) ) ;
#17451=CARTESIAN_POINT ( 'NONE',  ( 9.353092632424999664, -76.74803656385299178, 8.121372504915999713 ) ) ;
#17455=CARTESIAN_POINT ( 'NONE',  ( 11.14495853502000067, -79.95735716685899774, -0.2109943715695999922 ) ) ;
#17461=CARTESIAN_POINT ( 'NONE',  ( -7.806617969149999503, -78.75641514274398958, 9.479055599837000301 ) ) ;
#17465=CARTESIAN_POINT ( 'NONE',  ( 0.000000000000000000, -75.15999999999999659, 0.000000000000000000 ) ) ;
#17466=CARTESIAN_POINT ( 'NONE',  ( -10.47020627418440242, -78.47916666666667140, 2.813789756862221214 ) ) ;
#17482=CARTESIAN_POINT ( 'NONE',  ( -7.408849624938999234, -79.26590222969299759, -8.421820339245000397 ) ) ;
#17498=CARTESIAN_POINT ( 'NONE',  ( -10.86381291811999894, -79.48018145514599553, -5.803755483477999633 ) ) ;
#17500=CARTESIAN_POINT ( 'NONE',  ( -6.022804356561167971, -78.02249797650281948, 8.904300299157986487 ) ) ;
#17501=CARTESIAN_POINT ( 'NONE',  ( 5.537129384246000541, -78.97065855411999280, 10.62336504503000079 ) ) ;
#17508=CARTESIAN_POINT ( 'NONE',  ( -10.58739904582000158, -77.85109353173099578, -3.839393962977000196 ) ) ;
#17510=CARTESIAN_POINT ( 'NONE',  ( -8.361631869233999481, -80.26504353420789073, 7.535039759702999440 ) ) ;
#17517=B_SPLINE_CURVE_WITH_KNOTS ( 'NONE', 3,
 ( #35755, #3885, #17466, #53197, #13913, #54077, #374, #31906, #26897, #13615, #35456, #21887, #49948, #4772, #13025, #4483, #27478, #53484 ),
 .UNSPECIFIED., .F., .F.,
 ( 4, 2, 2, 2, 2, 2, 2, 2, 4 ),
 ( 0.000000000000000000, 0.1250000000000000000, 0.2500000000000000000, 0.3750000000000000000, 0.5000000000000000000, 0.6250000000000000000, 0.7500000000000000000, 0.8750000000000000000, 1.000000000000000000 ),
 .UNSPECIFIED. ) ;
#17524=CIRCLE ( 'NONE', #5270, 9.599999999999999645 ) ;
#17529=CARTESIAN_POINT ( 'NONE',  ( 2.958310398169000432, -77.35523885853200454, -10.74723220921999989 ) ) ;
#17535=CARTESIAN_POINT ( 'NONE',  ( -4.082680704644886305, -80.19438284699886310, -9.944308183758115760 ) ) ;
#17538=EDGE_CURVE ( 'NONE', #35854, #1173, #34711, .T. ) ;
#17543=CARTESIAN_POINT ( 'NONE',  ( -9.744524944696001612, -79.43148518439899419, -5.412839751281999234 ) ) ;
#17547=DIRECTION ( 'NONE',  ( -1.558387406072000046E-11, -1.000000000000000000, -1.336738014604999829E-10 ) ) ;
#17550=CARTESIAN_POINT ( 'NONE',  ( 11.05000000000000071, -82.00000000000000000, 0.000000000000000000 ) ) ;
#17553=CARTESIAN_POINT ( 'NONE',  ( -10.22609403765000025, -79.67173935843099741, -4.138687607718999573 ) ) ;
#17554=CARTESIAN_POINT ( 'NONE',  ( -1.570796326794885012, -76.41458333330569985, -12.00000000000000178 ) ) ;
#17563=CARTESIAN_POINT ( 'NONE',  ( 0.000000000000000000, -76.14999999999999147, 0.000000000000000000 ) ) ;
#17576=CARTESIAN_POINT ( 'NONE',  ( 9.514701387850999836, -76.23623749738399624, -5.285895731461000224 ) ) ;
#17584=CARTESIAN_POINT ( 'NONE',  ( -0.8451721318799240157, -80.98139021206071675, 10.71663691162798315 ) ) ;
#17585=CARTESIAN_POINT ( 'NONE',  ( -2.612980907336999614, -80.44026683748349171, -10.95817168551000087 ) ) ;
#17588=ORIENTED_EDGE ( 'NONE', *, *, #42567, .F. ) ;
#17600=CARTESIAN_POINT ( 'NONE',  ( -12.00000000000000178, -78.91041666666664867, -1.570796326794897668 ) ) ;
#17604=DIRECTION ( 'NONE',  ( 0.000000000000000000, -1.000000000000000000, 0.000000000000000000 ) ) ;
#17608=CARTESIAN_POINT ( 'NONE',  ( 8.059793245469082379, -77.29260984181965455, -7.115412693491175666 ) ) ;
#17612=CIRCLE ( 'NONE', #32680, 9.599999999999999645 ) ;
#17613=ORIENTED_EDGE ( 'NONE', *, *, #18928, .T. ) ;
#17619=CARTESIAN_POINT ( 'NONE',  ( 7.966054476048999078, -77.50865908154399619, 9.040893068079999040 ) ) ;
#17625=CARTESIAN_POINT ( 'NONE',  ( 10.48428321214112202, -76.60764424186088206, -6.042971066631413812 ) ) ;
#17629=DIRECTION ( 'NONE',  ( -1.000000000000000000, 0.000000000000000000, 0.000000000000000000 ) ) ;
#17636=CARTESIAN_POINT ( 'NONE',  ( 5.137083998358000336, -77.31100733245999379, -10.56753840748999984 ) ) ;
#17657=CARTESIAN_POINT ( 'NONE',  ( 10.50536548972000084, -77.75467495194999401, -2.968612793496999913 ) ) ;
#17658=CARTESIAN_POINT ( 'NONE',  ( 11.26957934775000147, -78.65591505001499684, 4.877733875464000057 ) ) ;
#17660=CARTESIAN_POINT ( 'NONE',  ( -5.413904038987160661, -79.08333333333332860, -9.393203674808278336 ) ) ;
#17664=ORIENTED_EDGE ( 'NONE', *, *, #46042, .F. ) ;
#17666=CARTESIAN_POINT ( 'NONE',  ( -11.29127801606999881, -79.09732492801998660, 3.839647735398000084 ) ) ;
#17667=CARTESIAN_POINT ( 'NONE',  ( -5.970469449440000353, -81.06265812071879395, 9.021904006163001810 ) ) ;
#17671=CARTESIAN_POINT ( 'NONE',  ( -6.659967121051000305, -76.90830639992499584, -9.025682433062998555 ) ) ;
#17683=CARTESIAN_POINT ( 'NONE',  ( 12.00000000000000888, -77.03958333333333997, -1.570796326794872577 ) ) ;
#17696=AXIS2_PLACEMENT_3D ( 'NONE', #29589, #25752, #43773 ) ;
#17698=CARTESIAN_POINT ( 'NONE',  ( -11.89890540480000070, -77.10472319096498950, 2.846590415137000285 ) ) ;
#17700=EDGE_CURVE ( 'NONE', #47139, #38464, #54469, .T. ) ;
#17702=EDGE_LOOP ( 'NONE', ( #52414, #19242, #5051, #35297 ) ) ;
#17703=B_SPLINE_CURVE_WITH_KNOTS ( 'NONE', 3,
 ( #12816, #30814, #48846, #37734, #55758, #33297, #51334, #46914, #42470, #2037 ),
 .UNSPECIFIED., .F., .F.,
 ( 4, 2, 2, 2, 4 ),
 ( 0.000000000000000000, 0.2500000000000000000, 0.5000000000000000000, 0.7500000000000000000, 1.000000000000000000 ),
 .UNSPECIFIED. ) ;
#17710=CARTESIAN_POINT ( 'NONE',  ( 10.34070037867000202, -77.96833891353188051, -4.346035695907999319 ) ) ;
#17713=CARTESIAN_POINT ( 'NONE',  ( -6.324515969367999979, -78.97901371548900329, -9.263833350438000380 ) ) ;
#17723=CARTESIAN_POINT ( 'NONE',  ( -4.885220488697999741, -76.60923828122899693, 11.26753068192000029 ) ) ;
#17727=CARTESIAN_POINT ( 'NONE',  ( -10.47020627418439354, -79.52083333333331439, -2.813789756862263847 ) ) ;
#17738=CARTESIAN_POINT ( 'NONE',  ( 10.95272639356999989, -78.85909624325299205, 4.740592608656999829 ) ) ;
#17741=CARTESIAN_POINT ( 'NONE',  ( 9.596002108778172612, -78.49791666666668277, -7.374560639698962028 ) ) ;
#17742=CARTESIAN_POINT ( 'NONE',  ( -0.2676215762113999808, -79.33579419080099626, 11.02860431212999970 ) ) ;
#17744=ORIENTED_EDGE ( 'NONE', *, *, #1954, .T. ) ;
#17750=CARTESIAN_POINT ( 'NONE',  ( -11.35613837876999987, -76.40844191910899497, 4.947237039123000280 ) ) ;
#17752=CARTESIAN_POINT ( 'NONE',  ( -5.052420809101000088E-14, -80.84999999994218456, 0.000000000000000000 ) ) ;
#17755=CARTESIAN_POINT ( 'NONE',  ( 8.858182419534999852, -80.07955691727549663, 6.954620140474000678 ) ) ;
#17758=LINE ( 'NONE', #9773, #53734 ) ;
#17764=CARTESIAN_POINT ( 'NONE',  ( -11.14010510836999934, -77.86114773376000642, -5.166607915801000317 ) ) ;
#17771=CARTESIAN_POINT ( 'NONE',  ( 10.54627086670829428, -78.83456760177642764, -2.082643228401557245 ) ) ;
#17777=CARTESIAN_POINT ( 'NONE',  ( 11.01479880718999915, -77.88671134015899611, -0.6131407820820000687 ) ) ;
#17781=CARTESIAN_POINT ( 'NONE',  ( 14.00000000000000000, -91.29999999999999716, 0.000000000000000000 ) ) ;
#17782=CARTESIAN_POINT ( 'NONE',  ( -8.286771986066998608, -78.63946634065099772, 7.559597915363999832 ) ) ;
#17784=EDGE_CURVE ( 'NONE', #21964, #2879, #21334, .T. ) ;
#17785=VERTEX_POINT ( 'NONE', #9542 ) ;
#17790=CARTESIAN_POINT ( 'NONE',  ( 0.000000000000000000, -87.64999999984398471, 0.000000000000000000 ) ) ;
#17793=AXIS2_PLACEMENT_3D ( 'NONE', #32795, #46132, #27502 ) ;
#17801=CARTESIAN_POINT ( 'NONE',  ( 9.131668046799001459, -79.13259514667099381, -8.265509513333999081 ) ) ;
#17802=CARTESIAN_POINT ( 'NONE',  ( 10.84835523999000095, -76.43206733076499404, -3.797607751403000442 ) ) ;
#17803=CARTESIAN_POINT ( 'NONE',  ( -3.181107275394350786, -77.99900448743609616, 10.27437500099360079 ) ) ;
#17804=CARTESIAN_POINT ( 'NONE',  ( 11.53501176087999980, -78.86214129242399906, -3.234124663588000104 ) ) ;
#17812=CARTESIAN_POINT ( 'NONE',  ( 9.608679508909999001, -77.18343933509500232, 5.650475968096999146 ) ) ;
#17813=DIRECTION ( 'NONE',  ( 0.000000000000000000, 1.000000000000000000, 0.000000000000000000 ) ) ;
#17815=ORIENTED_EDGE ( 'NONE', *, *, #30139, .F. ) ;
#17823=CARTESIAN_POINT ( 'NONE',  ( 3.630949683904999947, -79.79999999999999716, -11.17491406647000041 ) ) ;
#17833=CARTESIAN_POINT ( 'NONE',  ( 6.393694643109999909, -77.38247520153299774, -9.131005934809000024 ) ) ;
#17839=CARTESIAN_POINT ( 'NONE',  ( -1.491254300649823561, -80.21401151211460956, -10.64863931018329879 ) ) ;
#17841=CARTESIAN_POINT ( 'NONE',  ( -11.20005099196198195, -78.84553010071444135, 0.6168198611958737310 ) ) ;
#17846=CARTESIAN_POINT ( 'NONE',  ( -10.33279081301000168, -79.92173935843149479, -4.181869747484999955 ) ) ;
#17853=ORIENTED_EDGE ( 'NONE', *, *, #2244, .F. ) ;
#17856=CARTESIAN_POINT ( 'NONE',  ( 2.853743189566999534E-14, -82.05000000008600125, 0.000000000000000000 ) ) ;
#17857=CARTESIAN_POINT ( 'NONE',  ( 3.315825420378000210, -79.29043055640599391, -10.52174111842000137 ) ) ;
#17879=CARTESIAN_POINT ( 'NONE',  ( 11.99999999999999822, -76.56041666666666856, 1.570796326794923203 ) ) ;
#17884=CARTESIAN_POINT ( 'NONE',  ( 5.246383657897999875, -77.46100733245999947, -10.79237965019999912 ) ) ;
#17885=CARTESIAN_POINT ( 'NONE',  ( -9.578166812159000898, -80.28977840746540551, 5.930253639820000089 ) ) ;
#17891=CARTESIAN_POINT ( 'NONE',  ( 10.75000000000000000, -79.25000000000000000, 0.000000000000000000 ) ) ;
#17909=CARTESIAN_POINT ( 'NONE',  ( -3.586356261501751685, -77.19801135428419059, -10.13419940784981499 ) ) ;
#17915=CARTESIAN_POINT ( 'NONE',  ( -9.422718869893611071, -76.08255208300656136, -7.240326068120862324 ) ) ;
#17918=CARTESIAN_POINT ( 'NONE',  ( 1.628430890020000188, -78.98730299628599028, 11.59185972383999896 ) ) ;
#17922=VECTOR ( 'NONE', #49131, 1000.000000000000000 ) ;
#17930=CARTESIAN_POINT ( 'NONE',  ( -11.96333271148828281, -79.79999999999996874, -0.9383198194705477668 ) ) ;
#17943=EDGE_CURVE ( 'NONE', #23718, #6742, #17158, .T. ) ;
#17954=CARTESIAN_POINT ( 'NONE',  ( 10.78933672403999999, -77.26442077791699603, -1.663003020634000073 ) ) ;
#17956=CARTESIAN_POINT ( 'NONE',  ( 0.3923696854197999961, -77.06875387357798957, -11.92498586577000097 ) ) ;
#17958=CARTESIAN_POINT ( 'NONE',  ( -10.47020627418439354, -79.02083333333332860, -2.813789756862263847 ) ) ;
#17963=EDGE_CURVE ( 'NONE', #31041, #8076, #49314, .T. ) ;
#17966=CARTESIAN_POINT ( 'NONE',  ( -6.925639247002999710, -80.71293126068253798, -8.766942257001000272 ) ) ;
#17969=CARTESIAN_POINT ( 'NONE',  ( -3.513443458492000016, -78.50133016130298813, -10.65240647004999985 ) ) ;
#17980=EDGE_CURVE ( 'NONE', #23438, #55197, #3056, .T. ) ;
#17994=CARTESIAN_POINT ( 'NONE',  ( -7.694727692044000200, -76.76262287232799508, -9.663281825523000634 ) ) ;
#17995=CARTESIAN_POINT ( 'NONE',  ( -9.337414570838035388, -78.64153581994834497, -5.340065548460428246 ) ) ;
#18003=CARTESIAN_POINT ( 'NONE',  ( -2.185791986076000004, -77.85939354152488079, -11.00183730042999564 ) ) ;
#18005=CARTESIAN_POINT ( 'NONE',  ( 3.113304451009999863, -78.49783470746899638, -10.55022916317000181 ) ) ;
#18015=CARTESIAN_POINT ( 'NONE',  ( -10.85634995915000012, -76.24039363648499545, -5.741293403527000017 ) ) ;
#18021=CARTESIAN_POINT ( 'NONE',  ( -9.393203674808288994, -77.95833333333331439, 5.413904038987134015 ) ) ;
#18022=AXIS2_PLACEMENT_3D ( 'NONE', #14924, #10516, #28499 ) ;
#18026=CARTESIAN_POINT ( 'NONE',  ( -10.75000000000000000, -79.10000000000000853, 0.000000000000000000 ) ) ;
#18030=CARTESIAN_POINT ( 'NONE',  ( 11.93224739473999918, -77.82818225714999016, 0.2386934378577999782 ) ) ;
#18034=CARTESIAN_POINT ( 'NONE',  ( 6.766101950298000212, -79.28132150479699192, 8.713300108436000002 ) ) ;
#18042=CARTESIAN_POINT ( 'NONE',  ( -10.75000000000000000, -77.50000000000000000, 0.000000000000000000 ) ) ;
#18043=VECTOR ( 'NONE', #37721, 1000.000000000000000 ) ;
#18046=CARTESIAN_POINT ( 'NONE',  ( 10.48543666025108045, -77.69166666666664867, 6.043427764450817641 ) ) ;
#18051=CARTESIAN_POINT ( 'NONE',  ( 2.417503760557000447, -80.13402960327920255, 10.77648496335999972 ) ) ;
#18063=DIRECTION ( 'NONE',  ( 0.000000000000000000, 1.000000000000000000, 0.000000000000000000 ) ) ;
#18064=CARTESIAN_POINT ( 'NONE',  ( 11.68767212001977995, -77.07083333333332575, 3.140974612311385972 ) ) ;
#18066=EDGE_LOOP ( 'NONE', ( #13472, #56367, #49136 ) ) ;
#18069=VERTEX_POINT ( 'NONE', #47743 ) ;
#18071=ORIENTED_EDGE ( 'NONE', *, *, #7408, .T. ) ;
#18073=CARTESIAN_POINT ( 'NONE',  ( -2.149738495732000043, -77.75052962514999422, -10.82036777477999934 ) ) ;
#18077=CARTESIAN_POINT ( 'NONE',  ( 8.822637088635000069, -80.06907204401800016, 6.926713255916000733 ) ) ;
#18078=CARTESIAN_POINT ( 'NONE',  ( 11.00000000000000000, -81.00000000000000000, -2.369510767747999942E-13 ) ) ;
#18097=CARTESIAN_POINT ( 'NONE',  ( -0.5618369672511999147, -78.81976746904300057, 12.30411280745000013 ) ) ;
#18098=CARTESIAN_POINT ( 'NONE',  ( 11.12058147857000101, -76.40800415033000093, 2.393126261371000041 ) ) ;
#18099=CARTESIAN_POINT ( 'NONE',  ( -5.096119853128885602, -78.01436659480762614, 9.465255242693306315 ) ) ;
#18100=CARTESIAN_POINT ( 'NONE',  ( -7.615853692923001184, -78.56371882276300767, 9.247423260715999405 ) ) ;
#18103=CARTESIAN_POINT ( 'NONE',  ( -10.75000000000000000, -79.10000000000000853, 0.000000000000000000 ) ) ;
#18104=DIRECTION ( 'NONE',  ( 0.000000000000000000, 1.000000000000000000, 0.000000000000000000 ) ) ;
#18105=CARTESIAN_POINT ( 'NONE',  ( 4.505820952106676991, -80.94097166855550540, 9.769115195850069711 ) ) ;
#18109=CARTESIAN_POINT ( 'NONE',  ( -8.595972950985999006, -77.94605693914598987, -7.096749227412000316 ) ) ;
#18111=CARTESIAN_POINT ( 'NONE',  ( 0.6391562500349999842, -80.52070440064619561, -11.12244055969000023 ) ) ;
#18116=EDGE_CURVE ( 'NONE', #23662, #18069, #18646, .T. ) ;
#18117=CARTESIAN_POINT ( 'NONE',  ( 10.34070037867000202, -77.91665569944899516, -4.346035695907999319 ) ) ;
#18124=DIRECTION ( 'NONE',  ( 1.000000000000000000, 0.000000000000000000, 0.000000000000000000 ) ) ;
#18127=CARTESIAN_POINT ( 'NONE',  ( 6.226899213932999722, -78.44886817601300777, -9.208165984944999494 ) ) ;
#18135=CARTESIAN_POINT ( 'NONE',  ( 4.039050189702500404, -78.50472688885261618, -10.27665506351381453 ) ) ;
#18139=CARTESIAN_POINT ( 'NONE',  ( -7.362671760698999535, -79.45872152740099637, -8.369328833011000057 ) ) ;
#18146=ORIENTED_EDGE ( 'NONE', *, *, #47949, .T. ) ;
#18148=VECTOR ( 'NONE', #35081, 1000.000000000000114 ) ;
#18154=CARTESIAN_POINT ( 'NONE',  ( -11.68767212001979061, -76.32083333328657204, -3.140974612311365988 ) ) ;
#18160=ORIENTED_EDGE ( 'NONE', *, *, #48091, .T. ) ;
#18167=CARTESIAN_POINT ( 'NONE',  ( 10.97835188747000146, -76.13641167266798959, -2.133021021907000048 ) ) ;
#18171=CARTESIAN_POINT ( 'NONE',  ( 10.72509179124999967, -76.76295827915599546, -1.855488532230999965 ) ) ;
#18173=DIRECTION ( 'NONE',  ( 1.776356839400000238E-14, 1.000000000000000000, -2.368475785867000094E-14 ) ) ;
#18175=CARTESIAN_POINT ( 'NONE',  ( -5.059370734576000395, -80.92182981354159210, -10.06538451635999998 ) ) ;
#18181=CARTESIAN_POINT ( 'NONE',  ( 8.828526701892000617, -80.53055989549440596, -6.997593314318000246 ) ) ;
#18209=CARTESIAN_POINT ( 'NONE',  ( -2.392725975098465074, -77.20730248118280770, -10.48021964594175692 ) ) ;
#18215=CARTESIAN_POINT ( 'NONE',  ( 0.000000000000000000, -91.29999999999999716, 0.000000000000000000 ) ) ;
#18218=CARTESIAN_POINT ( 'NONE',  ( 9.201871282504999527, -77.99698675917198898, 7.779546039068999441 ) ) ;
#18221=VERTEX_POINT ( 'NONE', #26422 ) ;
#18238=CARTESIAN_POINT ( 'NONE',  ( 6.444980599755001371, -77.82020409095497371, -10.09843005143000028 ) ) ;
#18240=CARTESIAN_POINT ( 'NONE',  ( -12.00000000000000000, -77.79999999999999716, 0.000000000000000000 ) ) ;
#18245=CARTESIAN_POINT ( 'NONE',  ( -0.001628325640062127776, -76.28437499999964189, 12.02130491422682113 ) ) ;
#18255=CARTESIAN_POINT ( 'NONE',  ( -6.700596268546000545, -78.59900158500599332, -8.618433365121999756 ) ) ;
#18264=CARTESIAN_POINT ( 'NONE',  ( -3.040271599595000040, -80.53806783066440289, 10.75083736931999923 ) ) ;
#18265=B_SPLINE_CURVE_WITH_KNOTS ( 'NONE', 3,
 ( #3048, #52920, #30174, #24896, #34891, #42914, #34027, #30467, #47938, #2756, #17184, #57344, #44063, #11903, #25179, #48498, #8040, #16337, #25467, #20475, #2472, #38470, #21328, #48224, #56486, #26038, #39338, #43202, #16908, #34316, #21615, #43487, #16043, #57629, #53204, #35171, #21043 ),
 .UNSPECIFIED., .F., .F.,
 ( 4, 2, 1, 2, 2, 1, 2, 2, 2, 2, 2, 1, 1, 1, 2, 2, 1, 1, 1, 1, 2, 2, 4 ),
 ( 0.000000000000000000, 0.1250000000000002498, 0.1875000000000003886, 0.2187500000000004441, 0.2500000000000004996, 0.3125000000000004996, 0.3437500000000005551, 0.3750000000000006106, 0.5000000000000008882, 0.5625000000000008882, 0.6250000000000009992, 0.6875000000000011102, 0.7187500000000013323, 0.7343750000000013323, 0.7421875000000013323, 0.7500000000000013323, 0.8125000000000003331, 0.8437499999999997780, 0.8593749999999994449, 0.8671874999999994449, 0.8710937499999994449, 0.8749999999999994449, 1.000000000000000000 ),
 .UNSPECIFIED. ) ;
#18268=CARTESIAN_POINT ( 'NONE',  ( 0.2654799511899000319, -78.52856650430499030, -11.21373274707999990 ) ) ;
#18272=CARTESIAN_POINT ( 'NONE',  ( 10.23553682900219997, -79.80000000000001137, -5.902732043069990553 ) ) ;
#18280=DIRECTION ( 'NONE',  ( 1.000000000000000000, 0.000000000000000000, 0.000000000000000000 ) ) ;
#18292=CARTESIAN_POINT ( 'NONE',  ( -11.45618833121000080, -76.72164013402299076, -4.619913290770000458 ) ) ;
#18293=DIRECTION ( 'NONE',  ( 0.000000000000000000, -1.000000000000000000, 0.000000000000000000 ) ) ;
#18298=CARTESIAN_POINT ( 'NONE',  ( 1.570796326794909881, -78.93541666666665435, -11.99999999999999822 ) ) ;
#18300=CIRCLE ( 'NONE', #13608, 9.700000000000001066 ) ;
#18314=CARTESIAN_POINT ( 'NONE',  ( 8.174587033571999228, -77.38791030902299894, -8.440297792765999674 ) ) ;
#18318=CARTESIAN_POINT ( 'NONE',  ( -10.39759693597000023, -79.78060327480652347, -4.208097972746998927 ) ) ;
#18319=ADVANCED_FACE ( 'NONE', ( #22887, #4890 ), #54766, .T. ) ;
#18324=CARTESIAN_POINT ( 'NONE',  ( -5.687706977064000746, -77.91268472315900340, 10.54353137130999940 ) ) ;
#18326=CARTESIAN_POINT ( 'NONE',  ( -0.7898276719169999849, -78.69632035071100518, -11.90847071177000061 ) ) ;
#18330=CARTESIAN_POINT ( 'NONE',  ( 2.277702604431000033, -78.60041292975199667, -10.79414087890000040 ) ) ;
#18339=CARTESIAN_POINT ( 'NONE',  ( -10.74112163982999846, -76.41618033130500010, -6.401740506992999791 ) ) ;
#18341=CARTESIAN_POINT ( 'NONE',  ( 6.475177433059985610, -76.82391735373433050, 8.671361647340340539 ) ) ;
#18344=CARTESIAN_POINT ( 'NONE',  ( -10.99597256337999873, -79.22197590580999815, -1.828438666275999935 ) ) ;
#18360=CARTESIAN_POINT ( 'NONE',  ( 6.043427764450761686, -79.63333333333329733, 10.48543666025110888 ) ) ;
#18362=CARTESIAN_POINT ( 'NONE',  ( 10.02574878253000001, -76.53653125905668730, 4.955627619753999902 ) ) ;
#18368=CARTESIAN_POINT ( 'NONE',  ( 5.745747329289000227, -78.59830952192000098, 9.633509135241000720 ) ) ;
#18369=CARTESIAN_POINT ( 'NONE',  ( 2.058965375186439850, -80.99999999999998579, 10.62807325966601724 ) ) ;
#18389=CARTESIAN_POINT ( 'NONE',  ( 8.267499179258999575, -79.69052343751299361, 9.286453045038999932 ) ) ;
#18390=CARTESIAN_POINT ( 'NONE',  ( 7.275132094855999654, -76.38840344678598626, -8.898375939052000305 ) ) ;
#18391=CARTESIAN_POINT ( 'NONE',  ( -5.979430363902880075, -78.02211092265793013, 8.933456918256680979 ) ) ;
#18392=CARTESIAN_POINT ( 'NONE',  ( -11.48784787867999846, -78.15677909140700308, -3.397854551190000016 ) ) ;
#18397=CARTESIAN_POINT ( 'NONE',  ( 6.314250260588329056, -80.92529071434553600, 8.699957920916412846 ) ) ;
#18399=CARTESIAN_POINT ( 'NONE',  ( 10.75000000000000000, -77.25000000000000000, 0.000000000000000000 ) ) ;
#18400=CARTESIAN_POINT ( 'NONE',  ( 7.154950478465999630, -77.21067567809700449, 8.547589380727000474 ) ) ;
#18401=CARTESIAN_POINT ( 'NONE',  ( -6.043427764450832740, -78.21666666666668277, 10.48543666025107512 ) ) ;
#18402=CARTESIAN_POINT ( 'NONE',  ( -10.17218724451999989, -80.42734534903739529, 4.253677135873000559 ) ) ;
#18406=CARTESIAN_POINT ( 'NONE',  ( -12.50000000000000000, -92.79999999999999716, 0.000000000000000000 ) ) ;
#18407=CARTESIAN_POINT ( 'NONE',  ( -8.729704736441000534, -77.64429226943099138, 7.043462628994999974 ) ) ;
#18417=AXIS2_PLACEMENT_3D ( 'NONE', #47404, #58195, #13312 ) ;
#18419=CARTESIAN_POINT ( 'NONE',  ( -9.244881144060999034, -76.75603931249200684, -6.227904302768000555 ) ) ;
#18428=CARTESIAN_POINT ( 'NONE',  ( 10.75000000000000000, -79.84999999999999432, -2.184490103126999767E-14 ) ) ;
#18433=CARTESIAN_POINT ( 'NONE',  ( -3.994755123096000560, -79.29530346938999230, 10.40656197200999955 ) ) ;
#18436=ORIENTED_EDGE ( 'NONE', *, *, #3355, .F. ) ;
#18449=EDGE_CURVE ( 'NONE', #54390, #28730, #54505, .T. ) ;
#18463=CARTESIAN_POINT ( 'NONE',  ( 1.328862289696999932, -80.06390824290198793, 11.18676134159000135 ) ) ;
#18469=CARTESIAN_POINT ( 'NONE',  ( -2.612980907336999614, -80.50805539075979311, -10.95817168551000087 ) ) ;
#18479=CARTESIAN_POINT ( 'NONE',  ( -7.704382235714319904, -79.53873634255802472, 7.497057296163620599 ) ) ;
#18482=ORIENTED_EDGE ( 'NONE', *, *, #13845, .T. ) ;
#18492=EDGE_CURVE ( 'NONE', #9748, #16988, #14327, .T. ) ;
#18493=CARTESIAN_POINT ( 'NONE',  ( -3.536653132374341979, -77.19840948458308105, -10.15163854538700505 ) ) ;
#18494=CARTESIAN_POINT ( 'NONE',  ( 12.00000000000000000, -79.04999999999999716, 0.000000000000000000 ) ) ;
#18500=CYLINDRICAL_SURFACE ( 'NONE', #40716, 12.00000000000000000 ) ;
#18502=CARTESIAN_POINT ( 'NONE',  ( -1.845833107322000011, -78.07837470544299663, 11.90750485256000069 ) ) ;
#18505=ORIENTED_EDGE ( 'NONE', *, *, #28091, .F. ) ;
#18509=CARTESIAN_POINT ( 'NONE',  ( 11.68767212001977995, -78.57083333333332575, 3.140974612311385972 ) ) ;
#18518=FACE_OUTER_BOUND ( 'NONE', #24251, .T. ) ;
#18519=CARTESIAN_POINT ( 'NONE',  ( 2.076475668830000121, -76.05845572278499844, 10.98918251355999942 ) ) ;
#18523=EDGE_CURVE ( 'NONE', #57578, #46084, #13817, .T. ) ;
#18525=CARTESIAN_POINT ( 'NONE',  ( 10.76566337430111275, -77.11291972185833288, -5.417667412981277408 ) ) ;
#18554=AXIS2_PLACEMENT_3D ( 'NONE', #35494, #53231, #57083 ) ;
#18556=CARTESIAN_POINT ( 'NONE',  ( -7.213067475145999552, -79.55009665242799599, 9.497763435974000856 ) ) ;
#18557=CARTESIAN_POINT ( 'NONE',  ( 11.01264074648000069, -80.33045002223688869, 0.9768939932525001479 ) ) ;
#18561=CARTESIAN_POINT ( 'NONE',  ( 0.1392748842281999744, -77.20790617294500180, 11.21600254538999941 ) ) ;
#18605=CARTESIAN_POINT ( 'NONE',  ( 6.233047529871999615, -78.98050366622999263, 9.960502923565000444 ) ) ;
#18607=CARTESIAN_POINT ( 'NONE',  ( -3.164411967817999827, -77.30594483241300452, -11.86639179494000018 ) ) ;
#18608=B_SPLINE_CURVE_WITH_KNOTS ( 'NONE', 3,
 ( #41894, #50770, #5871, #1182 ),
 .UNSPECIFIED., .F., .F.,
 ( 4, 4 ),
 ( 0.000000000000000000, 1.000000000000000000 ),
 .UNSPECIFIED. ) ;
#18617=CARTESIAN_POINT ( 'NONE',  ( 11.36821324764999908, -77.72277951519299677, -3.778861202892000115 ) ) ;
#18619=CARTESIAN_POINT ( 'NONE',  ( 6.071186539538999227, -77.84184313900898644, 10.40848046910999791 ) ) ;
#18623=CARTESIAN_POINT ( 'NONE',  ( 9.849799932654001111, -79.81206640024099386, 4.707101791649999534 ) ) ;
#18625=EDGE_LOOP ( 'NONE', ( #26533, #39685, #14568, #49753, #14708 ) ) ;
#18637=CARTESIAN_POINT ( 'NONE',  ( 8.591781367357000931, -78.51383098776300073, 7.101823234627000048 ) ) ;
#18646=CIRCLE ( 'NONE', #39363, 9.700000000000001066 ) ;
#18655=ORIENTED_EDGE ( 'NONE', *, *, #46553, .F. ) ;
#18656=CARTESIAN_POINT ( 'NONE',  ( 7.602019699312583256, -78.78750673935347493, -7.600759696224709927 ) ) ;
#18658=ORIENTED_EDGE ( 'NONE', *, *, #17700, .F. ) ;
#18662=CARTESIAN_POINT ( 'NONE',  ( 9.271914673454089595, -76.74308161707607212, -7.928664495432715675 ) ) ;
#18663=CARTESIAN_POINT ( 'NONE',  ( 10.69399390970047747, -78.26269357169036311, -5.399859776636326103 ) ) ;
#18664=CARTESIAN_POINT ( 'NONE',  ( -5.268979267983999293, -78.68001855092498431, 9.902321347348999936 ) ) ;
#18665=CARTESIAN_POINT ( 'NONE',  ( 10.98952246480719808, -80.99999999999997158, 0.8689862965050588750 ) ) ;
#18668=ORIENTED_EDGE ( 'NONE', *, *, #27751, .F. ) ;
#18676=LINE ( 'NONE', #18962, #7323 ) ;
#18682=CARTESIAN_POINT ( 'NONE',  ( -8.405409561606999702, -79.37590556260300900, 9.003060531051000126 ) ) ;
#18683=CARTESIAN_POINT ( 'NONE',  ( -10.05101082620999797, -76.10235696248199133, 5.326514725976999820 ) ) ;
#18684=CARTESIAN_POINT ( 'NONE',  ( 4.695313984048824274, -77.93919653761264499, 9.670285837986678956 ) ) ;
#18690=CARTESIAN_POINT ( 'NONE',  ( 11.12972475151000040, -78.13671134015899611, -0.6195381557079999713 ) ) ;
#18692=CARTESIAN_POINT ( 'NONE',  ( -6.449172644969999979, -80.46700902863899785, -9.084347907802998279 ) ) ;
#18696=CARTESIAN_POINT ( 'NONE',  ( 9.869466656387999137, -76.90891100838200600, -5.330266269891000164 ) ) ;
#18700=CARTESIAN_POINT ( 'NONE',  ( -9.984017254981614187, -78.53079889738936004, -4.071156503779041813 ) ) ;
#18706=B_SPLINE_SURFACE_WITH_KNOTS ( 'NONE', 3, 3, ( 
 ( #25790, #39375, #30783, #53237, #12785, #21358, #44377, #57661, #35205, #53530, #12219, #26071, #3363, #57381, #48817, #40239, #34922, #8956, #26358, #52953, #3929, #12502, #44973, #26940, #39940, #57956, #30501, #48530, #17510, #44097, #35500, #13070, #39081, #31068, #44677 ),
 ( #21075, #57088, #4230, #22228, #58254, #49997, #27816, #36105, #5396, #32824, #4822, #50574, #27526, #40539, #23405, #41415, #37265, #32531, #19274, #27234, #45568, #18111, #14825, #18692, #50869, #50284, #13663, #9543, #31658, #10129, #134, #5113, #55279, #23692, #998 ),
 ( #28107, #13956, #23112, #10415, #18984, #32241, #41120, #36685, #54701, #14245, #9835, #28401, #46157, #9249, #5682, #41705, #45863, #4529, #36976, #22529, #45273, #49702, #54122, #1281, #22821, #40831, #424, #18402, #54989, #54420, #14537, #31952, #6265, #20152, #43169 ),
 ( #46447, #6851, #56162, #20436, #23979, #38139, #47032, #52030, #2726, #24861, #42877, #20722, #2435, #28694, #1566, #11870, #15711, #34279, #47322, #56742, #51744, #55873, #19858, #37556, #38432, #33120, #24280, #33705, #11294, #29274, #46745, #56449, #24570, #42587, #16004 ) ),
 .UNSPECIFIED., .F., .F., .F.,
 ( 4, 4 ),
 ( 4, 1, 1, 1, 1, 1, 1, 1, 1, 1, 1, 1, 1, 1, 1, 1, 1, 1, 1, 1, 1, 1, 1, 1, 1, 1, 1, 1, 1, 1, 1, 1, 4 ),
 ( -0.1772706441294000235, 1.177270644128999955 ),
 ( 0.4972775948320999895, 0.5132957106829999505, 0.5293138265339000226, 0.5453319423849000147, 0.5613500582358000868, 0.5773681740867999679, 0.5933862899377000399, 0.6094044057886000010, 0.6254225216395999931, 0.6414406374904999542, 0.6574587533414000262, 0.6734768691924000183, 0.6894949850432999794, 0.7055131008942999715, 0.7215312167452000436, 0.7375493325960998936, 0.7535674484470999968, 0.7695855642979999578, 0.7856036801490000610, 0.8016217959999000220, 0.8176399118507999830, 0.8336580277017999752, 0.8496761435527000472, 0.8656942594036999283, 0.8817123752546000004, 0.8977304911055000725, 0.9137486069564999536, 0.9297667228074000256, 0.9457848386584000178, 0.9618029545093000898, 0.9778210703601999398, 0.9938391862111999320, 1.009857302061999862 ),
 .UNSPECIFIED. ) ;
#18707=B_SPLINE_CURVE_WITH_KNOTS ( 'NONE', 3,
 ( #50552, #9810, #37531, #23382, #33393, #28967, #46134, #10986, #27795, #5658, #41392, #14804, #10693, #45839, #23667, #10104, #46422, #36953 ),
 .UNSPECIFIED., .F., .F.,
 ( 4, 2, 2, 2, 2, 2, 2, 2, 4 ),
 ( 0.000000000000000000, 0.1250000000000000000, 0.2500000000000000000, 0.3750000000000000000, 0.5000000000000000000, 0.6250000000000000000, 0.7500000000000000000, 0.8750000000000000000, 1.000000000000000000 ),
 .UNSPECIFIED. ) ;
#18721=CARTESIAN_POINT ( 'NONE',  ( 8.680500415593000341, -78.62837685893698847, 7.175156920760000112 ) ) ;
#18723=ORIENTED_EDGE ( 'NONE', *, *, #756, .F. ) ;
#18733=CARTESIAN_POINT ( 'NONE',  ( -5.413904038987160661, -78.08333333333332860, -9.393203674808278336 ) ) ;
#18749=CARTESIAN_POINT ( 'NONE',  ( 7.551392188974999975, -80.01374543289598762, 8.117862728809001283 ) ) ;
#18752=CARTESIAN_POINT ( 'NONE',  ( 7.288337508342944027, -76.16067708288093741, -9.485192864111416711 ) ) ;
#18759=DIRECTION ( 'NONE',  ( 1.186310310053999794E-10, -0.9999999999999998890, -1.114594443524999723E-08 ) ) ;
#18766=CARTESIAN_POINT ( 'NONE',  ( -7.882289591833920639, -79.54063170175217579, 7.310012099975937261 ) ) ;
#18784=CARTESIAN_POINT ( 'NONE',  ( -7.474107310857593944, -77.16382243072474978, -7.726686437686844044 ) ) ;
#18785=CARTESIAN_POINT ( 'NONE',  ( 7.223234266884172250, -79.12379502737748282, 9.635782272402776627 ) ) ;
#18786=VERTEX_POINT ( 'NONE', #38498 ) ;
#18794=CARTESIAN_POINT ( 'NONE',  ( 4.928445265185000146, -78.34966785968099146, -10.99573548889999941 ) ) ;
#18800=CARTESIAN_POINT ( 'NONE',  ( -6.043427764450832740, -78.71666666666668277, 10.48543666025107512 ) ) ;
#18810=CARTESIAN_POINT ( 'NONE',  ( -7.860507001410999450, -76.63534038853499908, 7.955276143908999842 ) ) ;
#18836=CARTESIAN_POINT ( 'NONE',  ( -11.14010510836999934, -77.40796654052100223, -5.166607915801000317 ) ) ;
#18843=CARTESIAN_POINT ( 'NONE',  ( 1.303850919141000153, -79.25712671310500923, -11.85478070107000015 ) ) ;
#18844=CARTESIAN_POINT ( 'NONE',  ( -4.745830983694999894, -81.18645468754350247, 10.10305395880000034 ) ) ;
#18863=CARTESIAN_POINT ( 'NONE',  ( 10.43567240482000003, -78.62076856562599403, 6.472443173969999464 ) ) ;
#18870=CARTESIAN_POINT ( 'NONE',  ( -12.22965310686000073, -76.12113747164599431, 0.3492514087541000456 ) ) ;
#18891=CARTESIAN_POINT ( 'NONE',  ( 8.135116633385999663, -77.01906566427899747, 9.200136113044999675 ) ) ;
#18904=CARTESIAN_POINT ( 'NONE',  ( 10.24006772854000147, -78.30304150121298790, 6.351124671173999481 ) ) ;
#18907=CARTESIAN_POINT ( 'NONE',  ( 9.298000630789001519, -79.25408516179498974, 5.937079976835999418 ) ) ;
#18914=CARTESIAN_POINT ( 'NONE',  ( -10.87500000000999911, -76.17499999999400018, 1.221063213659000093E-09 ) ) ;
#18916=CARTESIAN_POINT ( 'NONE',  ( -7.918603267607000618, -76.30298211639099293, 9.677277400644999972 ) ) ;
#18921=CARTESIAN_POINT ( 'NONE',  ( 7.759949366729999909, -78.89513978978800424, -8.002361301306001096 ) ) ;
#18923=CARTESIAN_POINT ( 'NONE',  ( -1.628633640557669793, -79.43583583485381894, 11.72084692437723596 ) ) ;
#18928=EDGE_CURVE ( 'NONE', #38464, #47139, #33620, .T. ) ;
#18941=CARTESIAN_POINT ( 'NONE',  ( 6.844432534029042614, -78.78001192501054106, -8.289462398550917044 ) ) ;
#18943=CARTESIAN_POINT ( 'NONE',  ( -10.15953550767560287, -76.71853632512886634, 4.239958222269431865 ) ) ;
#18948=CARTESIAN_POINT ( 'NONE',  ( -11.48800504392370136, -78.07278836372438491, -3.397901037234756672 ) ) ;
#18949=CARTESIAN_POINT ( 'NONE',  ( -1.780884232981000181, -79.94620619628149427, -11.07459082487999957 ) ) ;
#18953=ORIENTED_EDGE ( 'NONE', *, *, #57145, .F. ) ;
#18957=CARTESIAN_POINT ( 'NONE',  ( 8.899186938125001944, -76.04999999999999716, 6.465637775217000005 ) ) ;
#18960=CARTESIAN_POINT ( 'NONE',  ( -9.596002108778160178, -78.45208333333329165, -7.374560639698984232 ) ) ;
#18962=CARTESIAN_POINT ( 'NONE',  ( 12.00000000000000000, -79.65000000000000568, 0.000000000000000000 ) ) ;
#18970=CARTESIAN_POINT ( 'NONE',  ( 11.88227737747000035, -79.09962671310499616, -3.660809691553999823 ) ) ;
#18972=CARTESIAN_POINT ( 'NONE',  ( 10.62431421503999829, -76.29661320193899599, -3.719179278686000067 ) ) ;
#18973=CARTESIAN_POINT ( 'NONE',  ( 6.557452544417663454, -77.92303101572309743, 8.547671910063542100 ) ) ;
#18974=CARTESIAN_POINT ( 'NONE',  ( 11.88382656225999945, -78.30602506152000331, -1.513515996960000054 ) ) ;
#18977=DIRECTION ( 'NONE',  ( 0.000000000000000000, -1.000000000000000000, 0.000000000000000000 ) ) ;
#18979=CARTESIAN_POINT ( 'NONE',  ( 3.801865584756635386, -80.94637847883083737, 10.05558785843397196 ) ) ;
#18982=CARTESIAN_POINT ( 'NONE',  ( 1.499018853861999956, -77.75540253813299785, 11.04570246958999924 ) ) ;
#18984=CARTESIAN_POINT ( 'NONE',  ( -5.192477750132000303, -81.04484212712090141, -9.726524605103000098 ) ) ;
#18988=CARTESIAN_POINT ( 'NONE',  ( -3.633103876188000125, -77.09956540939499803, 10.61219425078000000 ) ) ;
#19001=CARTESIAN_POINT ( 'NONE',  ( -3.140974612311351777, -79.40416666666665435, -11.68767212001978884 ) ) ;
#19010=CARTESIAN_POINT ( 'NONE',  ( 8.677112325477001065, -80.26182985286258997, 6.812460760216000111 ) ) ;
#19026=CARTESIAN_POINT ( 'NONE',  ( 2.813789756862274505, -78.14583333333331439, -10.47020627418438821 ) ) ;
#19044=CARTESIAN_POINT ( 'NONE',  ( -10.34138800174999950, -80.73365051625088995, 4.468208825537999473 ) ) ;
#19045=CARTESIAN_POINT ( 'NONE',  ( -1.570796326794938524, -76.68541666666665435, 11.99999999999999645 ) ) ;
#19049=CARTESIAN_POINT ( 'NONE',  ( 6.043427764450763462, -78.23333333333330586, 10.48543666025111065 ) ) ;
#19053=DIRECTION ( 'NONE',  ( 0.000000000000000000, 1.000000000000000000, 0.000000000000000000 ) ) ;
#19058=FACE_OUTER_BOUND ( 'NONE', #8737, .T. ) ;
#19062=CARTESIAN_POINT ( 'NONE',  ( 7.556724790768792666, -79.41296073501848696, 7.645833190873140950 ) ) ;
#19066=FACE_OUTER_BOUND ( 'NONE', #50575, .T. ) ;
#19082=CARTESIAN_POINT ( 'NONE',  ( 11.66950233118999947, -79.43216740133399867, -2.920592611544999606 ) ) ;
#19095=CARTESIAN_POINT ( 'NONE',  ( 6.436424241555000592, -80.32391735373440156, 8.610165096135999008 ) ) ;
#19099=CARTESIAN_POINT ( 'NONE',  ( -4.800187936532999800, -76.17640816003999760, 10.10109298474000106 ) ) ;
#19112=AXIS2_PLACEMENT_3D ( 'NONE', #56326, #38012, #10582 ) ;
#19118=LINE ( 'NONE', #37108, #12797 ) ;
#19132=CARTESIAN_POINT ( 'NONE',  ( 2.357318282665999742, -80.85060369710272710, -11.04016127279999893 ) ) ;
#19135=CARTESIAN_POINT ( 'NONE',  ( -11.21668965365999959, -77.90213061526299043, -0.06311738993059998193 ) ) ;
#19141=CARTESIAN_POINT ( 'NONE',  ( -4.467577721914089750, -76.11770833332741404, 10.04328771562428813 ) ) ;
#19142=EDGE_CURVE ( 'NONE', #33872, #41200, #28329, .T. ) ;
#19144=CARTESIAN_POINT ( 'NONE',  ( 12.00000000000000000, -77.14999999999999147, 0.000000000000000000 ) ) ;
#19148=VERTEX_POINT ( 'NONE', #53165 ) ;
#19151=CARTESIAN_POINT ( 'NONE',  ( 6.544501642745999881, -77.92906724646599059, -10.25436633016999899 ) ) ;
#19163=CARTESIAN_POINT ( 'NONE',  ( -10.47145679359999981, -76.08015473334098999, 6.327539751872000018 ) ) ;
#19164=CARTESIAN_POINT ( 'NONE',  ( 10.35105862822000056, -79.84913938103490239, 3.468557695829999954 ) ) ;
#19166=CARTESIAN_POINT ( 'NONE',  ( 5.387243066085122933, -80.76671136794503525, -9.328540033652242158 ) ) ;
#19171=CARTESIAN_POINT ( 'NONE',  ( -9.302864017704999711, -76.79717616445388728, -6.266965030820998983 ) ) ;
#19183=CARTESIAN_POINT ( 'NONE',  ( 12.24159337356999977, -76.30973022145700213, -0.9828625608234000666 ) ) ;
#19190=ADVANCED_FACE ( 'NONE', ( #9172 ), #12985, .F. ) ;
#19198=CARTESIAN_POINT ( 'NONE',  ( 12.02223179210000126, -78.76423986341698935, 0.8134715296432000198 ) ) ;
#19209=CARTESIAN_POINT ( 'NONE',  ( -6.633107506946999798, -76.45391306960999600, -10.59980473414000102 ) ) ;
#19212=DIRECTION ( 'NONE',  ( 0.000000000000000000, -1.000000000000000000, 0.000000000000000000 ) ) ;
#19214=CARTESIAN_POINT ( 'NONE',  ( -10.80063122475000092, -78.79944879618999209, -3.190662894339999944 ) ) ;
#19216=CARTESIAN_POINT ( 'NONE',  ( -11.75721612854724363, -79.54603331170258684, 0.5654014867660701604 ) ) ;
#19231=CARTESIAN_POINT ( 'NONE',  ( 6.075412649139570576, -78.77296812514245516, -8.868588324655249266 ) ) ;
#19233=CARTESIAN_POINT ( 'NONE',  ( 7.995633008690000487, -76.56161320104568802, 7.819446035993999899 ) ) ;
#19238=CARTESIAN_POINT ( 'NONE',  ( 0.4844351086939314155, -77.42168479355439104, 11.97018437499462351 ) ) ;
#19239=CARTESIAN_POINT ( 'NONE',  ( 6.879576957522999692, -79.08856369595298474, 8.859431780707000215 ) ) ;
#19240=ORIENTED_EDGE ( 'NONE', *, *, #30139, .T. ) ;
#19242=ORIENTED_EDGE ( 'NONE', *, *, #55070, .T. ) ;
#19261=CARTESIAN_POINT ( 'NONE',  ( -10.48543666025109289, -79.44166666666666288, -6.043427764450796325 ) ) ;
#19263=CARTESIAN_POINT ( 'NONE',  ( 4.370542281221782233, -77.94187509226848931, 9.823968797400164377 ) ) ;
#19265=CARTESIAN_POINT ( 'NONE',  ( 4.458743082292000004, -77.47854620581199470, 11.11915799896999957 ) ) ;
#19272=CARTESIAN_POINT ( 'NONE',  ( -9.889498855898999352, -78.42232914858598747, 4.888716273084000363 ) ) ;
#19273=CARTESIAN_POINT ( 'NONE',  ( -7.650089724727000551, -76.72148282161819566, -9.607224057717001386 ) ) ;
#19274=CARTESIAN_POINT ( 'NONE',  ( 9.770225111710999499, -80.60124745865709883, -5.353494744805000316 ) ) ;
#19279=CARTESIAN_POINT ( 'NONE',  ( -9.302864017704999711, -76.74549295037100194, -6.266965030821000759 ) ) ;
#19284=CARTESIAN_POINT ( 'NONE',  ( -2.717027075192881114, -78.60471625112383265, -10.43420719071179548 ) ) ;
#19293=CARTESIAN_POINT ( 'NONE',  ( 3.140974612311327796, -77.65416666666665435, 11.68767212001979594 ) ) ;
#19296=CARTESIAN_POINT ( 'NONE',  ( -5.969148455088877370, -80.17823147499480285, -8.940398062078001473 ) ) ;
#19304=CARTESIAN_POINT ( 'NONE',  ( -11.13008859988999966, -78.88675832436199187, 0.6129668257943999832 ) ) ;
#19310=ORIENTED_EDGE ( 'NONE', *, *, #32952, .T. ) ;
#19311=ORIENTED_EDGE ( 'NONE', *, *, #35614, .T. ) ;
#19322=DIRECTION ( 'NONE',  ( 0.000000000000000000, -1.000000000000000000, 0.000000000000000000 ) ) ;
#19329=CARTESIAN_POINT ( 'NONE',  ( 12.00000000000000000, -76.64999999999999147, 0.000000000000000000 ) ) ;
#19333=CARTESIAN_POINT ( 'NONE',  ( 8.440675369999999234, -80.00371287089478756, 7.053722371789000967 ) ) ;
#19335=CARTESIAN_POINT ( 'NONE',  ( 11.68767212001978173, -77.17083333333333428, 3.140974612311388192 ) ) ;
#19342=LINE ( 'NONE', #41774, #45959 ) ;
#19344=ORIENTED_EDGE ( 'NONE', *, *, #55333, .F. ) ;
#19351=CARTESIAN_POINT ( 'NONE',  ( 10.66182291595043452, -79.36152322765421729, 1.544088080186965195 ) ) ;
#19365=CARTESIAN_POINT ( 'NONE',  ( -6.990209140086781403, -77.16870983874881063, -8.167017623392847980 ) ) ;
#19370=CARTESIAN_POINT ( 'NONE',  ( 3.552363299575000077, -79.78274967992298627, -11.49294985030999960 ) ) ;
#19374=CARTESIAN_POINT ( 'NONE',  ( -11.01904509677000021, -78.09203558730200712, 4.584337204197000304 ) ) ;
#19391=DIRECTION ( 'NONE',  ( -1.000000000000000000, 0.000000000000000000, 0.000000000000000000 ) ) ;
#19393=CARTESIAN_POINT ( 'NONE',  ( 5.380788203752000065, -76.03337378079599773, 9.804131929786001010 ) ) ;
#19403=CARTESIAN_POINT ( 'NONE',  ( 0.000000000000000000, -75.15999999999999659, 0.000000000000000000 ) ) ;
#19404=CARTESIAN_POINT ( 'NONE',  ( -10.55336135317719304, -78.08483439053425457, 2.046528030539819021 ) ) ;
#19426=CARTESIAN_POINT ( 'NONE',  ( -2.590408569657000282, -80.88335807551204937, -11.10753917875999974 ) ) ;
#19429=CARTESIAN_POINT ( 'NONE',  ( 9.144378690012999300, -77.60253084224299869, -6.496033325431000094 ) ) ;
#19446=CARTESIAN_POINT ( 'NONE',  ( -9.840265838668001308, -78.30887766239899861, -7.152041583326999685 ) ) ;
#19452=EDGE_CURVE ( 'NONE', #15698, #1523, #8551, .T. ) ;
#19460=CARTESIAN_POINT ( 'NONE',  ( -10.31421052434999908, -76.72175206120299151, 3.823226550887000030 ) ) ;
#19471=CARTESIAN_POINT ( 'NONE',  ( -11.38972971424999869, -76.59660938959198972, -4.593112662244999811 ) ) ;
#19476=CARTESIAN_POINT ( 'NONE',  ( -9.066796825632000179, -78.80009492674068383, -6.603885667862000375 ) ) ;
#19478=DIRECTION ( 'NONE',  ( 0.000000000000000000, 0.000000000000000000, -1.000000000000000000 ) ) ;
#19483=CARTESIAN_POINT ( 'NONE',  ( -9.747171129529000666, -78.05887766239899861, -7.084379058567000342 ) ) ;
#19487=CARTESIAN_POINT ( 'NONE',  ( 8.414343270883998471, -78.83155805217599266, 6.955155862361000807 ) ) ;
#19494=CARTESIAN_POINT ( 'NONE',  ( 0.000000000000000000, -75.15999999999999659, 0.000000000000000000 ) ) ;
#19499=CARTESIAN_POINT ( 'NONE',  ( -9.103325846391999931, -78.82668513919199427, -6.630491919364000175 ) ) ;
#19501=CARTESIAN_POINT ( 'NONE',  ( 11.75055246895291994, -79.79038423862893126, -1.413995404558705760 ) ) ;
#19502=LINE ( 'NONE', #15065, #53297 ) ;
#19508=CARTESIAN_POINT ( 'NONE',  ( -2.848604465265602403, -78.95447547272175370, -10.84928852802099009 ) ) ;
#19512=CARTESIAN_POINT ( 'NONE',  ( 0.000000000000000000, -87.25000000009099210, -9.649999999909001147 ) ) ;
#19515=CARTESIAN_POINT ( 'NONE',  ( -11.68767212001979594, -77.27916666666666856, 3.140974612311315806 ) ) ;
#19520=DIRECTION ( 'NONE',  ( 0.000000000000000000, 1.000000000000000000, 0.000000000000000000 ) ) ;
#19521=CARTESIAN_POINT ( 'NONE',  ( 8.948459357138670356, -78.80341436924688026, -5.956977988863866535 ) ) ;
#19524=CARTESIAN_POINT ( 'NONE',  ( 7.778176538613999824, -76.43620349110052814, -8.035785801754000701 ) ) ;
#19528=CARTESIAN_POINT ( 'NONE',  ( 9.789953784408815807, -78.75102124931834169, -6.904838711737845358 ) ) ;
#19529=CARTESIAN_POINT ( 'NONE',  ( -0.4146318973827000098, -79.38816346897299070, -11.20920117498000046 ) ) ;
#19547=CARTESIAN_POINT ( 'NONE',  ( 8.098906566116852446, -77.90749627220959894, 7.103892318221430635 ) ) ;
#19548=CARTESIAN_POINT ( 'NONE',  ( 0.9627474882855999727, -78.19750779982500433, -11.94107121277999894 ) ) ;
#19553=CARTESIAN_POINT ( 'NONE',  ( 10.43503646057562229, -80.86970219550423167, 2.582246741427850267 ) ) ;
#19556=CARTESIAN_POINT ( 'NONE',  ( 6.225574660483999878, -78.28614743357699979, 9.107357164861998200 ) ) ;
#19557=CARTESIAN_POINT ( 'NONE',  ( -11.38972971424999869, -76.68050008331320555, -4.593112662244999811 ) ) ;
#19564=CARTESIAN_POINT ( 'NONE',  ( 0.1392748842281999744, -77.14011761966898462, 11.21600254538999941 ) ) ;
#19578=CARTESIAN_POINT ( 'NONE',  ( 11.99999999999999822, -77.56041666666668277, 1.570796326794923203 ) ) ;
#19587=CARTESIAN_POINT ( 'NONE',  ( 2.165712778014000417, -78.75057660935300419, 10.93454565734000106 ) ) ;
#19600=CARTESIAN_POINT ( 'NONE',  ( 7.374560639698993114, -76.47708333331846120, -9.596002108778149520 ) ) ;
#19602=CARTESIAN_POINT ( 'NONE',  ( -1.407171709420418138, -78.11458333333331439, -10.75000000000000000 ) ) ;
#19606=CARTESIAN_POINT ( 'NONE',  ( 12.00000000000000000, -77.64999999999999147, 0.000000000000000000 ) ) ;
#19609=DIRECTION ( 'NONE',  ( 0.000000000000000000, 1.000000000000000000, 0.000000000000000000 ) ) ;
#19611=EDGE_CURVE ( 'NONE', #18221, #33152, #57930, .T. ) ;
#19615=CARTESIAN_POINT ( 'NONE',  ( 4.336551063001060413, -77.45429869360749819, -11.23466680206521673 ) ) ;
#19631=ORIENTED_EDGE ( 'NONE', *, *, #9718, .F. ) ;
#19640=CIRCLE ( 'NONE', #1786, 9.599999999999999645 ) ;
#19651=CARTESIAN_POINT ( 'NONE',  ( 7.614522461194726866, -80.28763416514415496, -7.588239908555904023 ) ) ;
#19652=CARTESIAN_POINT ( 'NONE',  ( -6.215526947630453769, -77.17609984879747742, -8.770830743108882999 ) ) ;
#19657=CARTESIAN_POINT ( 'NONE',  ( 0.4713521909880000194, -79.07356383116399456, 12.02020425643999957 ) ) ;
#19662=CARTESIAN_POINT ( 'NONE',  ( -11.91766194687999914, -78.11916490272500369, 0.6362673702790999641 ) ) ;
#19666=CARTESIAN_POINT ( 'NONE',  ( -10.75000000000000355, -78.98958333333331439, 1.407171709420384609 ) ) ;
#19676=CARTESIAN_POINT ( 'NONE',  ( 1.005394801847710129, -79.80000000000001137, -11.73748890211396301 ) ) ;
#19682=CARTESIAN_POINT ( 'NONE',  ( 7.778176538613999824, -76.38452096864399721, -8.035785801754000701 ) ) ;
#19689=CARTESIAN_POINT ( 'NONE',  ( 0.000000000000000000, -75.15999999999999659, 0.000000000000000000 ) ) ;
#19694=CARTESIAN_POINT ( 'NONE',  ( -10.65825678370000063, -79.61563558397199358, -5.693941594808000772 ) ) ;
#19695=CARTESIAN_POINT ( 'NONE',  ( -10.58971709958329477, -78.08629155915249953, 1.850469969248101254 ) ) ;
#19716=CARTESIAN_POINT ( 'NONE',  ( 1.860817577827999836, -80.63854927348660340, 11.25277748102000075 ) ) ;
#19720=CARTESIAN_POINT ( 'NONE',  ( 1.633411169670999863, -78.03831233027200653, -11.09730050697999992 ) ) ;
#19724=DIRECTION ( 'NONE',  ( 0.000000000000000000, -1.000000000000000000, 0.000000000000000000 ) ) ;
#19725=CARTESIAN_POINT ( 'NONE',  ( 10.61868686143207441, -80.99999999999998579, -2.878266372804510809 ) ) ;
#19728=CARTESIAN_POINT ( 'NONE',  ( 3.228614917279000185, -80.84644807899644547, -10.79283437469000084 ) ) ;
#19737=CARTESIAN_POINT ( 'NONE',  ( -11.66523904145000046, -78.28174834697500728, -3.450322983582000180 ) ) ;
#19745=CARTESIAN_POINT ( 'NONE',  ( 6.606167539452195925, -77.77712013868713825, -8.596032059636364409 ) ) ;
#19749=CARTESIAN_POINT ( 'NONE',  ( 3.281228840419999848, -79.22270349199298778, -10.41195962760999905 ) ) ;
#19761=CARTESIAN_POINT ( 'NONE',  ( -9.393203674808267678, -77.54166666666665719, -5.413904038987171319 ) ) ;
#19766=CARTESIAN_POINT ( 'NONE',  ( 4.297951556683999641, -76.78734615778300565, -11.50435740523999861 ) ) ;
#19771=CARTESIAN_POINT ( 'NONE',  ( 6.766402264611000028, -79.42653081578252738, -8.946167390840999545 ) ) ;
#19780=CARTESIAN_POINT ( 'NONE',  ( 11.05834404496999923, -78.79136917884000013, 4.786306364259000468 ) ) ;
#19786=CARTESIAN_POINT ( 'NONE',  ( -10.54577208822472834, -79.58458823469565857, 2.085048453671053181 ) ) ;
#19797=VERTEX_POINT ( 'NONE', #31481 ) ;
#19798=CARTESIAN_POINT ( 'NONE',  ( -7.330610599118999815, -79.20799394121699777, 8.549626471514999437 ) ) ;
#19799=CARTESIAN_POINT ( 'NONE',  ( 10.97853902630967937, -76.08461633803946711, -2.133057381744011938 ) ) ;
#19800=CARTESIAN_POINT ( 'NONE',  ( -11.58850405216667667, -79.03337548462275208, 2.406487868672887664 ) ) ;
#19807=CARTESIAN_POINT ( 'NONE',  ( -11.05000000000000071, -76.00000000000000000, 0.000000000000000000 ) ) ;
#19816=CARTESIAN_POINT ( 'NONE',  ( 3.168421713927999761, -77.47183533742300199, -12.18315494261000076 ) ) ;
#19817=CARTESIAN_POINT ( 'NONE',  ( 8.368138856150174831, -78.79614046870541699, -6.748098975523931564 ) ) ;
#19818=AXIS2_PLACEMENT_3D ( 'NONE', #48482, #24881, #15731 ) ;
#19825=CARTESIAN_POINT ( 'NONE',  ( -7.654125837341301697, -77.12040900012513589, -9.499792065586241563 ) ) ;
#19826=CARTESIAN_POINT ( 'NONE',  ( -1.835150331438888616, -77.93714178660536618, 11.83859006001563507 ) ) ;
#19827=CARTESIAN_POINT ( 'NONE',  ( -11.04065564778000130, -79.31977030723999178, 1.980412446595999798 ) ) ;
#19832=CARTESIAN_POINT ( 'NONE',  ( -7.803971648336165856, -78.28613751752133965, 8.057272210502093301 ) ) ;
#19839=CARTESIAN_POINT ( 'NONE',  ( 0.000000000000000000, -81.00000000000000000, 0.000000000000000000 ) ) ;
#19846=CARTESIAN_POINT ( 'NONE',  ( -5.768141930173999121, -78.78679903547799768, 11.01445829398999798 ) ) ;
#19849=CARTESIAN_POINT ( 'NONE',  ( 11.95248949435000085, -78.82148205457200163, 0.8087524912306001124 ) ) ;
#19856=CARTESIAN_POINT ( 'NONE',  ( 8.921077980507002181, -78.25891109057499762, 6.489691983999000158 ) ) ;
#19857=CARTESIAN_POINT ( 'NONE',  ( 7.144724566336000393, -76.47558639178819817, 9.988770583665001368 ) ) ;
#19858=CARTESIAN_POINT ( 'NONE',  ( -3.014980776116999994, -80.62931084346850241, -10.48587037275000000 ) ) ;
#19863=CARTESIAN_POINT ( 'NONE',  ( 10.75000000000000000, -80.34999999999999432, 0.000000000000000000 ) ) ;
#19864=CARTESIAN_POINT ( 'NONE',  ( -3.633103876188000125, -77.16735396267098679, 10.61219425078000000 ) ) ;
#19868=CARTESIAN_POINT ( 'NONE',  ( -7.695965602004000594, -76.50616330962898815, 9.405193249304000247 ) ) ;
#19871=TOROIDAL_SURFACE ( 'NONE', #3779, 12.50000000000000000, 1.500000000000000000 ) ;
#19876=CARTESIAN_POINT ( 'NONE',  ( 11.13061814830999907, -77.01442077791699603, -1.715606072514000102 ) ) ;
#19879=CARTESIAN_POINT ( 'NONE',  ( 1.570796326794857478, -77.66458333333333997, 12.00000000000000533 ) ) ;
#19886=CARTESIAN_POINT ( 'NONE',  ( -10.53927088184999938, -79.93499373684079501, 3.259678459687000096 ) ) ;
#19902=CARTESIAN_POINT ( 'NONE',  ( 11.21485848424000054, -79.94681080473810653, -0.2123177049684000228 ) ) ;
#19908=CARTESIAN_POINT ( 'NONE',  ( 10.10565965529137422, -76.05000000000001137, -4.494725398901759483 ) ) ;
#19911=CARTESIAN_POINT ( 'NONE',  ( 9.760776772971999193, -92.33215535459000023, 3.252741292258000451E-10 ) ) ;
#19913=CARTESIAN_POINT ( 'NONE',  ( 7.374560639698954922, -76.72291666666664867, 9.596002108778179718 ) ) ;
#19921=CARTESIAN_POINT ( 'NONE',  ( 7.374560639698954922, -77.22291666666666288, 9.596002108778179718 ) ) ;
#19925=CARTESIAN_POINT ( 'NONE',  ( -11.68767212001980127, -78.37916666666666288, 3.140974612311317138 ) ) ;
#19929=ORIENTED_EDGE ( 'NONE', *, *, #48693, .F. ) ;
#19939=CARTESIAN_POINT ( 'NONE',  ( -1.242042303480714205, -79.48436884964252158, 10.67792447292398705 ) ) ;
#19952=CARTESIAN_POINT ( 'NONE',  ( 8.165383881631132823, -80.29366675105114837, -6.993337379266368004 ) ) ;
#19953=CARTESIAN_POINT ( 'NONE',  ( -7.580572135914469101, -77.16272471331792815, -7.622152899789345959 ) ) ;
#19959=CARTESIAN_POINT ( 'NONE',  ( -5.246265831776000255, -79.72298241822798559, -10.82514862071000117 ) ) ;
#19963=CARTESIAN_POINT ( 'NONE',  ( -5.666254562607999645, -78.03777695645399604, 10.50376416711000083 ) ) ;
#19968=ORIENTED_EDGE ( 'NONE', *, *, #1247, .F. ) ;
#19979=CARTESIAN_POINT ( 'NONE',  ( 11.15514985639044276, -79.79999999999998295, 3.879996556239171834 ) ) ;
#19983=CARTESIAN_POINT ( 'NONE',  ( -7.695020077040999773, -76.26927865530500128, 8.115451295621999961 ) ) ;
#19984=CARTESIAN_POINT ( 'NONE',  ( 10.38093530541932985, -76.32946667606279334, -2.901028463810237490 ) ) ;
#19994=CARTESIAN_POINT ( 'NONE',  ( -7.318775999449999681, -79.58266715040700490, -9.761385579090999798 ) ) ;
#19996=CARTESIAN_POINT ( 'NONE',  ( -8.368009042705715217, -78.04613955777109879, 6.748258816816721684 ) ) ;
#20001=CARTESIAN_POINT ( 'NONE',  ( 6.233047529871999615, -78.98050366622999263, 9.960502923565000444 ) ) ;
#20016=CARTESIAN_POINT ( 'NONE',  ( -4.413100828165999800, -80.04845022661349674, 10.26392002655999924 ) ) ;
#20019=CARTESIAN_POINT ( 'NONE',  ( 11.08595418830999968, -77.13951301121200288, -1.708721840212999998 ) ) ;
#20026=DIRECTION ( 'NONE',  ( 0.000000000000000000, 1.000000000000000000, -1.657933050107000062E-13 ) ) ;
#20029=ORIENTED_EDGE ( 'NONE', *, *, #26108, .T. ) ;
#20034=CARTESIAN_POINT ( 'NONE',  ( 11.16396169635999946, -79.04136917884000013, 4.832020119862000307 ) ) ;
#20036=CARTESIAN_POINT ( 'NONE',  ( -8.596529571091879873, -77.54793149518738460, 6.606441957186066638 ) ) ;
#20044=CARTESIAN_POINT ( 'NONE',  ( -0.7035745874731462735, -77.71981679028705514, -10.74957825944642487 ) ) ;
#20048=CARTESIAN_POINT ( 'NONE',  ( 10.60715898610999908, -79.30441252099899430, -2.581384170113000032 ) ) ;
#20055=CARTESIAN_POINT ( 'NONE',  ( 11.70000000000000107, -79.79999999999999716, 0.000000000000000000 ) ) ;
#20065=CARTESIAN_POINT ( 'NONE',  ( 2.548493721447000038, -76.99225984930698985, 12.01365081398999912 ) ) ;
#20068=ORIENTED_EDGE ( 'NONE', *, *, #45244, .T. ) ;
#20075=CARTESIAN_POINT ( 'NONE',  ( 4.484759669696999573, -77.35351546138099366, 11.18403784080000030 ) ) ;
#20080=CARTESIAN_POINT ( 'NONE',  ( -10.75000000000000000, -79.59999999999999432, 0.000000000000000000 ) ) ;
#20085=CARTESIAN_POINT ( 'NONE',  ( -6.654586241810727998, -76.22057291693802483, -8.660536402383590016 ) ) ;
#20093=CARTESIAN_POINT ( 'NONE',  ( -7.553623922565042115, -79.11961698824401878, -9.109432733142380556 ) ) ;
#20110=CARTESIAN_POINT ( 'NONE',  ( 5.096297253146042650, -78.76436718932042425, -9.465160375605314869 ) ) ;
#20119=CARTESIAN_POINT ( 'NONE',  ( -9.805641529082999241, -79.37424299324300137, -5.446788484474000214 ) ) ;
#20126=CARTESIAN_POINT ( 'NONE',  ( -6.884902925240382388, -78.42231923253098103, -8.855492064945991615 ) ) ;
#20133=VECTOR ( 'NONE', #43108, 1000.000000000000000 ) ;
#20135=DIRECTION ( 'NONE',  ( 1.000000000000000000, 0.000000000000000000, 0.000000000000000000 ) ) ;
#20136=CARTESIAN_POINT ( 'NONE',  ( 11.92746894621999942, -79.41036807549798482, 1.562891678063999867 ) ) ;
#20140=CARTESIAN_POINT ( 'NONE',  ( -12.14769635903000200, -78.85631629717299518, 2.650188445066000043 ) ) ;
#20142=CARTESIAN_POINT ( 'NONE',  ( 9.329378798893031899, -79.30846558317799122, -5.387576131639663757 ) ) ;
#20143=CARTESIAN_POINT ( 'NONE',  ( 11.81379047889000056, -77.39715825954098705, 1.987564636421000008 ) ) ;
#20149=CARTESIAN_POINT ( 'NONE',  ( -10.60678368039263297, -76.58707232302387524, 1.749019199596896001 ) ) ;
#20150=CARTESIAN_POINT ( 'NONE',  ( -7.585478157043000103, -77.52352982952599803, -8.010134550088000793 ) ) ;
#20152=CARTESIAN_POINT ( 'NONE',  ( 7.321105331825000562, -80.27520846168349067, 8.057475193947000847 ) ) ;
#20157=CARTESIAN_POINT ( 'NONE',  ( -8.595351952246861771, -80.54797288116316167, 6.605825225780209919 ) ) ;
#20158=CARTESIAN_POINT ( 'NONE',  ( -3.244487197725999916, -76.86775418965099504, -10.73738397614000029 ) ) ;
#20162=CARTESIAN_POINT ( 'NONE',  ( 8.006345619697000870, -77.19309101131499062, -8.693492320142999219 ) ) ;
#20165=ORIENTED_EDGE ( 'NONE', *, *, #42080, .T. ) ;
#20172=CARTESIAN_POINT ( 'NONE',  ( 0.000000000000000000, -87.29999999999999716, 0.000000000000000000 ) ) ;
#20175=FACE_BOUND ( 'NONE', #33000, .T. ) ;
#20185=EDGE_LOOP ( 'NONE', ( #55543, #15154 ) ) ;
#20192=CARTESIAN_POINT ( 'NONE',  ( 3.340492633907115039, -76.26875000031391494, -10.28561997391731175 ) ) ;
#20195=VERTEX_POINT ( 'NONE', #16532 ) ;
#20196=VERTEX_POINT ( 'NONE', #15659 ) ;
#20198=CARTESIAN_POINT ( 'NONE',  ( -11.87139580924456261, -76.91341727770499404, -2.023209039049733704 ) ) ;
#20200=DIRECTION ( 'NONE',  ( 0.000000000000000000, -1.000000000000000000, 0.000000000000000000 ) ) ;
#20203=CARTESIAN_POINT ( 'NONE',  ( -6.606377239730330864, -76.57291666666665719, -8.596418555780440229 ) ) ;
#20204=CARTESIAN_POINT ( 'NONE',  ( 11.68767212001978173, -76.67083333333333428, 3.140974612311388192 ) ) ;
#20218=CARTESIAN_POINT ( 'NONE',  ( 1.570796326794856590, -78.26458333333330586, 12.00000000000000711 ) ) ;
#20230=CARTESIAN_POINT ( 'NONE',  ( -2.521418227633154263, -79.49383760258125164, 10.45011237715473129 ) ) ;
#20235=CARTESIAN_POINT ( 'NONE',  ( 4.205198518925999274, -76.79725762008598622, -10.19892346455999999 ) ) ;
#20241=CARTESIAN_POINT ( 'NONE',  ( 6.107111665684042734, -80.27352331620853931, -8.846533776856475129 ) ) ;
#20242=CARTESIAN_POINT ( 'NONE',  ( -10.94712378871737535, -76.21666666663080036, 4.871360733705688340 ) ) ;
#20244=CARTESIAN_POINT ( 'NONE',  ( -11.60111135005000094, -79.15519343212500303, -3.181408645392000523 ) ) ;
#20247=DIRECTION ( 'NONE',  ( 0.000000000000000000, 1.000000000000000000, 0.000000000000000000 ) ) ;
#20251=CARTESIAN_POINT ( 'NONE',  ( -11.69669687464000063, -78.60749258035299647, 2.371241166392999755 ) ) ;
#20266=CARTESIAN_POINT ( 'NONE',  ( 1.052500557283970073, -79.80000000000002558, -11.73283057634160720 ) ) ;
#20267=CARTESIAN_POINT ( 'NONE',  ( -5.880916218342844282, -80.02142361888905953, 9.002827806299052327 ) ) ;
#20269=CARTESIAN_POINT ( 'NONE',  ( 7.486068761172999686, -75.95067068213799644, -8.059700645992000645 ) ) ;
#20273=CARTESIAN_POINT ( 'NONE',  ( -9.877439518601001112, -76.85324162823199856, 5.094664542828000187 ) ) ;
#20279=CARTESIAN_POINT ( 'NONE',  ( 6.411492066225999764, -79.40708379888700108, 10.24266459616000091 ) ) ;
#20280=CARTESIAN_POINT ( 'NONE',  ( -10.39983874692026866, -78.07962607350559381, 2.743425914733084614 ) ) ;
#20288=DIRECTION ( 'NONE',  ( 0.000000000000000000, 1.000000000000000000, 0.000000000000000000 ) ) ;
#20296=VERTEX_POINT ( 'NONE', #30371 ) ;
#20301=CARTESIAN_POINT ( 'NONE',  ( 10.34070037867000202, -78.12002135927799884, -4.346035695907999319 ) ) ;
#20317=CARTESIAN_POINT ( 'NONE',  ( 11.54375705602000046, -77.98332587731398746, -3.837213001227999687 ) ) ;
#20322=CARTESIAN_POINT ( 'NONE',  ( 11.99999999999999822, -79.56041666666666856, 1.570796326794923203 ) ) ;
#20324=ORIENTED_EDGE ( 'NONE', *, *, #55347, .F. ) ;
#20326=CARTESIAN_POINT ( 'NONE',  ( 8.500174178665998781, -78.26943148693000296, -6.849988769802000554 ) ) ;
#20338=CARTESIAN_POINT ( 'NONE',  ( 6.606377239730347739, -77.67708333333330017, -8.596418555780422466 ) ) ;
#20341=ADVANCED_FACE ( 'NONE', ( #8527 ), #27042, .F. ) ;
#20344=CARTESIAN_POINT ( 'NONE',  ( -4.885220488697999741, -76.54144972795299395, 11.26753068192000029 ) ) ;
#20348=TOROIDAL_SURFACE ( 'NONE', #27872, 9.799999999999998934, 0.2000000000000000111 ) ;
#20357=CARTESIAN_POINT ( 'NONE',  ( -12.04425331849999914, -78.45234896019000814, -1.708359618215999909 ) ) ;
#20361=CARTESIAN_POINT ( 'NONE',  ( 10.91653581620999880, -78.77708536617198831, 0.06787400445098999702 ) ) ;
#20369=CARTESIAN_POINT ( 'NONE',  ( -2.047671225339077468E-06, -76.25353340279926329, -10.79679441329301959 ) ) ;
#20375=CARTESIAN_POINT ( 'NONE',  ( 10.09881335831000015, -78.99010319720299833, -4.984770136353999348 ) ) ;
#20376=CARTESIAN_POINT ( 'NONE',  ( 7.995769303601012012, -76.66150100378845877, 7.819579327592078855 ) ) ;
#20381=CARTESIAN_POINT ( 'NONE',  ( 10.75000000000000000, -79.75000000000000000, 0.000000000000000000 ) ) ;
#20389=CARTESIAN_POINT ( 'NONE',  ( -3.243675144747000250, -77.43085259911799767, -12.16362487391999991 ) ) ;
#20390=CARTESIAN_POINT ( 'NONE',  ( 5.081957869198564737, -78.76424439475270844, -9.472868843939814099 ) ) ;
#20392=ORIENTED_EDGE ( 'NONE', *, *, #18116, .T. ) ;
#20403=CARTESIAN_POINT ( 'NONE',  ( 0.9578316561262000262, -78.96569784821599569, -11.17589679220000143 ) ) ;
#20406=CARTESIAN_POINT ( 'NONE',  ( 12.50000000000000000, -92.79999999999999716, 0.000000000000000000 ) ) ;
#20407=EDGE_LOOP ( 'NONE', ( #42619, #12297, #19310, #46112, #47650, #51409, #6955, #27987, #17815 ) ) ;
#20411=CARTESIAN_POINT ( 'NONE',  ( 12.00000000000000000, -78.14999999999999147, 0.000000000000000000 ) ) ;
#20413=DIRECTION ( 'NONE',  ( 0.000000000000000000, 1.000000000000000000, 2.042110567139000169E-13 ) ) ;
#20427=CARTESIAN_POINT ( 'NONE',  ( 8.547552837677239168, -79.29805100310200316, -6.557471810879811791 ) ) ;
#20428=CARTESIAN_POINT ( 'NONE',  ( -3.085175050843000477, -78.10258993112499581, -11.57574012064000080 ) ) ;
#20432=CARTESIAN_POINT ( 'NONE',  ( 10.45146978769019519, -80.86920117642237926, 2.514705922069923716 ) ) ;
#20435=CARTESIAN_POINT ( 'NONE',  ( 2.927762776937000044, -77.60523885853200454, -10.63625589685999984 ) ) ;
#20436=CARTESIAN_POINT ( 'NONE',  ( -1.662621324463000150, -81.13941687753749932, -10.78329382847999973 ) ) ;
#20444=CARTESIAN_POINT ( 'NONE',  ( 4.275724345439000373, -76.92222687565399042, -10.36997068233999997 ) ) ;
#20448=CARTESIAN_POINT ( 'NONE',  ( 6.568955083609000489, -77.24824049629300760, -9.863814250127001415 ) ) ;
#20459=CARTESIAN_POINT ( 'NONE',  ( 1.570796326794909881, -76.93541666666666856, -11.99999999999999822 ) ) ;
#20464=DIRECTION ( 'NONE',  ( 0.000000000000000000, -1.000000000000000000, 0.000000000000000000 ) ) ;
#20466=EDGE_LOOP ( 'NONE', ( #3023, #20756, #30666, #18658 ) ) ;
#20475=CARTESIAN_POINT ( 'NONE',  ( -8.593914503524631598, -81.00000000000001421, -6.616432748763715566 ) ) ;
#20476=CARTESIAN_POINT ( 'NONE',  ( 0.1355484243948000267, -76.94742129968800270, 10.91590548763000079 ) ) ;
#20491=CARTESIAN_POINT ( 'NONE',  ( -10.48543666025111776, -76.85833333333330586, 6.043427764450754580 ) ) ;
#20498=CARTESIAN_POINT ( 'NONE',  ( 3.140974612311326908, -77.25416666666664867, 11.68767212001979772 ) ) ;
#20514=CARTESIAN_POINT ( 'NONE',  ( -8.098724780893656217, -77.04286527309800192, 7.103750973452154227 ) ) ;
#20522=CARTESIAN_POINT ( 'NONE',  ( -7.719769492146999923, -76.57936687607200099, 7.579341418041000367 ) ) ;
#20528=CARTESIAN_POINT ( 'NONE',  ( 8.058982427891788092, -80.29245933814496539, -7.115972638186089938 ) ) ;
#20530=CARTESIAN_POINT ( 'NONE',  ( -11.97916666630055715, -76.27916666661793954, 1.256637064247476676 ) ) ;
#20532=CARTESIAN_POINT ( 'NONE',  ( 8.348735229153000148, -78.87821946291599318, 8.268078378528999295 ) ) ;
#20534=CARTESIAN_POINT ( 'NONE',  ( -9.018305195942000196, -79.77230326501299373, 6.745675351750000104 ) ) ;
#20546=EDGE_LOOP ( 'NONE', ( #49967, #49588, #13246, #16467 ) ) ;
#20553=CARTESIAN_POINT ( 'NONE',  ( -5.576379918403213232, -79.79999999999998295, -10.46867297261899488 ) ) ;
#20554=CARTESIAN_POINT ( 'NONE',  ( -9.416831372289546920, -80.06003372581248811, 5.217560844161510225 ) ) ;
#20557=CARTESIAN_POINT ( 'NONE',  ( 11.01994305158000031, -76.63805051245100231, -1.906499110313000234 ) ) ;
#20558=CARTESIAN_POINT ( 'NONE',  ( 3.687685142782404224, -76.44819997255908106, 10.12799054552703382 ) ) ;
#20560=CARTESIAN_POINT ( 'NONE',  ( 7.516229220974000924, -76.00797436215698610, -8.092172198832999541 ) ) ;
#20566=CARTESIAN_POINT ( 'NONE',  ( 4.732552697730000091, -79.16556358023599671, -11.24509117424000060 ) ) ;
#20567=CARTESIAN_POINT ( 'NONE',  ( -10.54480093980093791, -78.08451164641000730, 2.090071665737717410 ) ) ;
#20572=CARTESIAN_POINT ( 'NONE',  ( 6.232755757386176043, -78.94717033289664698, 9.960036924250847079 ) ) ;
#20573=CARTESIAN_POINT ( 'NONE',  ( 5.413904038987148226, -80.16666666666664298, -9.393203674808285442 ) ) ;
#20579=CARTESIAN_POINT ( 'NONE',  ( 0.000000000000000000, -75.15999999999999659, 0.000000000000000000 ) ) ;
#20586=CARTESIAN_POINT ( 'NONE',  ( -9.421357847594000745, -80.29617642373133890, -6.176342950743000770 ) ) ;
#20587=CARTESIAN_POINT ( 'NONE',  ( -4.505191439890000815, -80.18390435543939532, 10.47810291308999986 ) ) ;
#20594=CARTESIAN_POINT ( 'NONE',  ( -1.575545371556065222, -79.98714921115445975, 10.63364149761491362 ) ) ;
#20607=AXIS2_PLACEMENT_3D ( 'NONE', #20579, #56884, #38577 ) ;
#20612=CARTESIAN_POINT ( 'NONE',  ( 4.654517711782999889, -79.41335789300599401, 9.874757255799998745 ) ) ;
#20624=CARTESIAN_POINT ( 'NONE',  ( 0.9627474882855999727, -78.28140245315898937, -11.94107121277999894 ) ) ;
#20633=CARTESIAN_POINT ( 'NONE',  ( -7.374560639698971798, -77.87291666666668277, -9.596002108778163731 ) ) ;
#20639=CARTESIAN_POINT ( 'NONE',  ( 11.36512682855729750, -78.67683455540999660, 3.982123233433211063 ) ) ;
#20641=CARTESIAN_POINT ( 'NONE',  ( 7.024610939158000278, -78.61512485273199502, -9.931634882699999167 ) ) ;
#20647=CARTESIAN_POINT ( 'NONE',  ( -10.56288039171200488, -79.58526307256707355, 1.996919741384027835 ) ) ;
#20650=CARTESIAN_POINT ( 'NONE',  ( -12.15598897987000093, -79.25941268769399528, -0.08388850244461000527 ) ) ;
#20653=CARTESIAN_POINT ( 'NONE',  ( -1.881081600302069390, -79.78749999999999432, 11.88906204917373088 ) ) ;
#20660=CARTESIAN_POINT ( 'NONE',  ( 5.177840772445237327, -76.68658294577745949, 9.913027470100756133 ) ) ;
#20662=CARTESIAN_POINT ( 'NONE',  ( 9.594300353386179481, -79.34959433123279382, 6.930735968784434320 ) ) ;
#20674=VERTEX_POINT ( 'NONE', #44128 ) ;
#20676=CARTESIAN_POINT ( 'NONE',  ( -1.955611496805000238, -76.87133267504599132, -12.31633344284000131 ) ) ;
#20677=CARTESIAN_POINT ( 'NONE',  ( -5.302235804606764802, -78.68411842716731996, -9.360073049705164294 ) ) ;
#20680=EDGE_CURVE ( 'NONE', #43698, #14636, #8605, .T. ) ;
#20685=EDGE_CURVE ( 'NONE', #32066, #38434, #17703, .T. ) ;
#20689=CARTESIAN_POINT ( 'NONE',  ( -5.268979267983999293, -78.74780710420199625, 9.902321347348999936 ) ) ;
#20705=CARTESIAN_POINT ( 'NONE',  ( -11.60111135005000094, -79.17129902871758418, -3.181408645392000523 ) ) ;
#20713=CARTESIAN_POINT ( 'NONE',  ( -4.743879332790999825, -78.59091760875300281, -11.00053059214000051 ) ) ;
#20720=CARTESIAN_POINT ( 'NONE',  ( 7.307192483546000261, -77.20994809191398645, -8.110505779365999146 ) ) ;
#20721=CARTESIAN_POINT ( 'NONE',  ( 10.75000000000000355, -79.23958333333332860, -1.407171709420407035 ) ) ;
#20722=CARTESIAN_POINT ( 'NONE',  ( -3.115648671636999989, -80.92463538950839563, 10.45640090600000072 ) ) ;
#20728=CARTESIAN_POINT ( 'NONE',  ( 0.000000000000000000, -75.15999999999999659, 0.000000000000000000 ) ) ;
#20730=CARTESIAN_POINT ( 'NONE',  ( 10.29113596735999892, -77.54866276469599029, 4.462133020506000136 ) ) ;
#20735=CARTESIAN_POINT ( 'NONE',  ( -2.462645637647999930, -77.18535259911799074, -11.90051400241999957 ) ) ;
#20755=VERTEX_POINT ( 'NONE', #49438 ) ;
#20756=ORIENTED_EDGE ( 'NONE', *, *, #26342, .T. ) ;
#20758=CARTESIAN_POINT ( 'NONE',  ( 8.060704535212000366, -77.76451158974199984, -7.362092663522999736 ) ) ;
#20763=CARTESIAN_POINT ( 'NONE',  ( 6.349001246031294343, -76.28437500015692763, -8.735174149410413591 ) ) ;
#20789=CARTESIAN_POINT ( 'NONE',  ( 7.102903299382745672, -80.31775757425651818, 8.111946779019859832 ) ) ;
#20794=CARTESIAN_POINT ( 'NONE',  ( -10.75000000000000000, -77.10000000000000853, 0.000000000000000000 ) ) ;
#20802=CARTESIAN_POINT ( 'NONE',  ( 10.27624888046999985, -77.92720206157000007, -4.318947732659999872 ) ) ;
#20808=CARTESIAN_POINT ( 'NONE',  ( 6.913388667549481781, -80.28076439126193975, -8.232022196888907573 ) ) ;
#20812=CARTESIAN_POINT ( 'NONE',  ( -11.95950202284999975, -78.98973269472499226, 1.295167635372999948 ) ) ;
#20814=CARTESIAN_POINT ( 'NONE',  ( 6.907293935673000540, -79.14586737597099386, 8.895125352942999442 ) ) ;
#20815=EDGE_LOOP ( 'NONE', ( #4714, #37482, #55598, #10311 ) ) ;
#20833=CARTESIAN_POINT ( 'NONE',  ( -4.881323669191630188, -80.01262565301878738, 9.577793144389749713 ) ) ;
#20834=DIRECTION ( 'NONE',  ( 1.000000000000000000, 0.000000000000000000, 0.000000000000000000 ) ) ;
#20836=CARTESIAN_POINT ( 'NONE',  ( -10.85772169724999969, -76.82108137906500644, 1.763485056683000041 ) ) ;
#20841=CARTESIAN_POINT ( 'NONE',  ( 11.14347266599000008, -76.08322018812400245, 1.380835503201000014 ) ) ;
#20848=CARTESIAN_POINT ( 'NONE',  ( -6.217680906644530658, -78.02424479843827498, 8.769644482899945359 ) ) ;
#20855=CARTESIAN_POINT ( 'NONE',  ( 1.384588047529715649, -79.16581540243207371, 11.96733435986142347 ) ) ;
#20867=CARTESIAN_POINT ( 'NONE',  ( -2.895922040489999905, -80.14568799371318164, 10.88681414971999928 ) ) ;
#20874=CARTESIAN_POINT ( 'NONE',  ( -1.846742135806079599, -79.98920618438151564, 10.59049653823865178 ) ) ;
#20877=CARTESIAN_POINT ( 'NONE',  ( 10.07294373702136170, -77.32156161217383783, -3.779831308317421534 ) ) ;
#20904=CARTESIAN_POINT ( 'NONE',  ( -8.328265577977349565, -80.29148630941537590, 7.504971905104131480 ) ) ;
#20905=EDGE_CURVE ( 'NONE', #4925, #4724, #46479, .T. ) ;
#20913=CARTESIAN_POINT ( 'NONE',  ( -11.38972971424999869, -76.52882083631500620, -4.593112662244999811 ) ) ;
#20925=CARTESIAN_POINT ( 'NONE',  ( 6.482586803565999922, -77.67906724646599059, -10.15735398655000132 ) ) ;
#20933=CARTESIAN_POINT ( 'NONE',  ( -11.45393214452999864, -79.28604631854099694, -4.072167004989999839 ) ) ;
#20939=CARTESIAN_POINT ( 'NONE',  ( -3.140974612311352221, -78.00416666666664867, -11.68767212001979061 ) ) ;
#20944=CARTESIAN_POINT ( 'NONE',  ( -2.463227758765337505, -79.15794654540887620, -11.57512065399542855 ) ) ;
#20951=LINE ( 'NONE', #38376, #48674 ) ;
#20959=CARTESIAN_POINT ( 'NONE',  ( -9.126129491359000312, -77.19919458148599745, 8.498837978755000577 ) ) ;
#20960=CARTESIAN_POINT ( 'NONE',  ( -2.423311762192682739, -78.70718521568076653, -10.49559937800138698 ) ) ;
#20968=CARTESIAN_POINT ( 'NONE',  ( 10.47045947498260965, -79.82917641337841985, -2.813952884208940741 ) ) ;
#20971=CARTESIAN_POINT ( 'NONE',  ( 10.05828973332000054, -79.04740687722198800, -4.964767691657000270 ) ) ;
#20982=CARTESIAN_POINT ( 'NONE',  ( -4.647153543919563923, -78.25890117452027539, 10.20909265806945676 ) ) ;
#20985=CARTESIAN_POINT ( 'NONE',  ( 2.813789756862229652, -80.85416666666665719, 10.47020627418440064 ) ) ;
#20993=CARTESIAN_POINT ( 'NONE',  ( 2.269106295766999856E-14, -92.56607767729998670, 0.000000000000000000 ) ) ;
#20998=CARTESIAN_POINT ( 'NONE',  ( 11.95248949435000085, -78.75369350129598445, 0.8087524912306001124 ) ) ;
#21008=AXIS2_PLACEMENT_3D ( 'NONE', #25355, #12077, #30058 ) ;
#21017=CARTESIAN_POINT ( 'NONE',  ( 4.610941639127999814, -76.73255973945900621, -11.24387672497000068 ) ) ;
#21022=CARTESIAN_POINT ( 'NONE',  ( -11.01515889844999840, -78.63675832436199187, 0.6066373079611000474 ) ) ;
#21026=CARTESIAN_POINT ( 'NONE',  ( -10.48543666025109111, -76.84166666666665435, -6.043427764450793660 ) ) ;
#21033=DIRECTION ( 'NONE',  ( -1.000000000000000000, 0.000000000000000000, 0.000000000000000000 ) ) ;
#21043=CARTESIAN_POINT ( 'NONE',  ( -10.75000000000000000, -81.00000000000000000, 2.851355842494999902E-13 ) ) ;
#21044=CARTESIAN_POINT ( 'NONE',  ( 9.410240357728000049, -76.86571227068199619, 5.533781925607000218 ) ) ;
#21048=CARTESIAN_POINT ( 'NONE',  ( 2.039250879084999912, -79.83786543273089364, -11.02993955029000084 ) ) ;
#21059=CARTESIAN_POINT ( 'NONE',  ( 10.75000000000000000, -76.75000000000000000, 0.000000000000000000 ) ) ;
#21064=CARTESIAN_POINT ( 'NONE',  ( -10.15836276337999955, -76.54404187781499047, 3.905545731297999978 ) ) ;
#21073=CARTESIAN_POINT ( 'NONE',  ( -9.563148796606999014, -77.27913032869298604, 5.948121522994000543 ) ) ;
#21075=CARTESIAN_POINT ( 'NONE',  ( 5.448459039171999585, -81.05765812071879850, -9.476848501824999715 ) ) ;
#21082=CARTESIAN_POINT ( 'NONE',  ( -11.14038684213999986, -78.18901912946698474, 1.307628137226999998 ) ) ;
#21091=DIRECTION ( 'NONE',  ( 0.000000000000000000, 1.000000000000000000, 0.000000000000000000 ) ) ;
#21094=CARTESIAN_POINT ( 'NONE',  ( -8.595972950985999006, -77.76378400355899601, -7.096749227412000316 ) ) ;
#21100=CARTESIAN_POINT ( 'NONE',  ( -3.746558969565879416, -80.19711350692230667, -10.07601878856429423 ) ) ;
#21103=CARTESIAN_POINT ( 'NONE',  ( 8.348735229153000148, -78.81043090964000442, 8.268078378528999295 ) ) ;
#21105=CARTESIAN_POINT ( 'NONE',  ( -2.860041384466000203, -78.92797663195699442, -10.89284755413000028 ) ) ;
#21123=CARTESIAN_POINT ( 'NONE',  ( -10.21779526337023114, -80.07488518645870101, 3.340465863513364830 ) ) ;
#21126=CARTESIAN_POINT ( 'NONE',  ( 2.076475668830000121, -76.19403282933799915, 10.98918251355999942 ) ) ;
#21129=CARTESIAN_POINT ( 'NONE',  ( 7.863749243303001180, -76.77047704070999146, 7.690468382148999638 ) ) ;
#21131=CARTESIAN_POINT ( 'NONE',  ( 0.000000000000000000, -75.15999999999999659, 0.000000000000000000 ) ) ;
#21134=CARTESIAN_POINT ( 'NONE',  ( -7.477182751274228600, -78.03619407845222611, 7.725621107446211333 ) ) ;
#21137=CARTESIAN_POINT ( 'NONE',  ( -0.8560878949168587715, -80.98146821848625621, 10.71577390680143971 ) ) ;
#21147=AXIS2_PLACEMENT_3D ( 'NONE', #57091, #24931, #24644 ) ;
#21153=CARTESIAN_POINT ( 'NONE',  ( 4.537811113640745297, -80.09166625100542092, 10.16818905941867968 ) ) ;
#21157=CARTESIAN_POINT ( 'NONE',  ( 9.596002108778174389, -79.09791666666666288, -7.374560639698961140 ) ) ;
#21160=CARTESIAN_POINT ( 'NONE',  ( 4.030751681420186472, -79.94461808928627988, 9.966766518696916322 ) ) ;
#21169=EDGE_CURVE ( 'NONE', #22103, #51194, #48800, .T. ) ;
#21173=CARTESIAN_POINT ( 'NONE',  ( -4.771559678803999560, -78.78373690646100158, -11.06471824780000013 ) ) ;
#21175=ORIENTED_EDGE ( 'NONE', *, *, #17963, .F. ) ;
#21183=CARTESIAN_POINT ( 'NONE',  ( -9.393849266501053563, -80.64169200378464097, -5.414091273218729405 ) ) ;
#21189=FACE_OUTER_BOUND ( 'NONE', #51989, .T. ) ;
#21199=CARTESIAN_POINT ( 'NONE',  ( 2.548493721447000038, -76.85668274275499812, 12.01365081398999912 ) ) ;
#21207=CARTESIAN_POINT ( 'NONE',  ( 11.88669912479000068, -78.20818512137599043, 2.586293583890999948 ) ) ;
#21212=CARTESIAN_POINT ( 'NONE',  ( -8.033734583472570634, -79.54227913950597895, 7.144481850731994932 ) ) ;
#21213=EDGE_LOOP ( 'NONE', ( #57245, #37021, #28993, #20165 ) ) ;
#21216=CARTESIAN_POINT ( 'NONE',  ( 11.77121427762000039, -79.45802193175599371, 2.535895762643999962 ) ) ;
#21241=CARTESIAN_POINT ( 'NONE',  ( -10.75040831495720361, -78.58963204257108259, 1.407120353455911133 ) ) ;
#21245=CARTESIAN_POINT ( 'NONE',  ( -7.768219623894999870, -76.83034993674100122, -9.755575312415000866 ) ) ;
#21246=CARTESIAN_POINT ( 'NONE',  ( 4.370112803705837656, -78.75831584482018854, -9.822244704776046831 ) ) ;
#21254=CARTESIAN_POINT ( 'NONE',  ( 6.329984427696999205, -78.07728428553903655, 9.260097609460000712 ) ) ;
#21257=CARTESIAN_POINT ( 'NONE',  ( -2.710423231297999891, -79.79610400554300043, 10.88447134676999895 ) ) ;
#21267=CARTESIAN_POINT ( 'NONE',  ( -11.14658556052672367, -76.84470657150592388, 0.7341312425827495325 ) ) ;
#21276=CARTESIAN_POINT ( 'NONE',  ( -5.092641036025000290, -79.55978622973557890, 10.89826376711000044 ) ) ;
#21278=CARTESIAN_POINT ( 'NONE',  ( -8.596418555780466875, -77.94791666666667140, 6.606377239730298001 ) ) ;
#21283=CARTESIAN_POINT ( 'NONE',  ( 3.249499231398999655, -78.64517623960099968, -11.53069031867000049 ) ) ;
#21286=CARTESIAN_POINT ( 'NONE',  ( -10.44638973513362856, -76.35792952211139095, 6.036140669651893553 ) ) ;
#21293=ORIENTED_EDGE ( 'NONE', *, *, #4233, .F. ) ;
#21297=CARTESIAN_POINT ( 'NONE',  ( 5.985848557435999417, -79.99298052329480413, -10.45156471383000074 ) ) ;
#21298=DIRECTION ( 'NONE',  ( 1.000000000000000000, 0.000000000000000000, 0.000000000000000000 ) ) ;
#21302=CARTESIAN_POINT ( 'NONE',  ( 12.18980338489999937, -76.24977255369199725, -1.398660325409999849 ) ) ;
#21306=CARTESIAN_POINT ( 'NONE',  ( 11.08725735368000009, -79.46710299282599976, 1.152095891907999992 ) ) ;
#21325=EDGE_LOOP ( 'NONE', ( #41210, #16407, #1892, #40818 ) ) ;
#21328=CARTESIAN_POINT ( 'NONE',  ( -9.538057720467248757, -80.99999999999997158, -5.099884920957399537 ) ) ;
#21329=CARTESIAN_POINT ( 'NONE',  ( 10.89987286286000057, -77.81898427574600419, -0.6067434084558999130 ) ) ;
#21331=CARTESIAN_POINT ( 'NONE',  ( 5.986115112277999195, -80.09630838701978917, 9.486000076385000312 ) ) ;
#21332=ORIENTED_EDGE ( 'NONE', *, *, #25946, .T. ) ;
#21334=B_SPLINE_CURVE_WITH_KNOTS ( 'NONE', 3,
 ( #49406, #13364, #133, #58253, #4821, #31362, #44376, #49105, #22820, #31951, #49996, #18401, #8955, #54419, #39655, #26939, #21930, #57955 ),
 .UNSPECIFIED., .F., .F.,
 ( 4, 2, 2, 2, 2, 2, 2, 2, 4 ),
 ( 0.000000000000000000, 0.1249999999999999722, 0.2499999999999999445, 0.3749999999999998890, 0.4999999999999998890, 0.6249999999999998890, 0.7499999999999997780, 0.8749999999999998890, 1.000000000000000000 ),
 .UNSPECIFIED. ) ;
#21343=CARTESIAN_POINT ( 'NONE',  ( 6.365665562422999635, -78.73050366622999263, 10.17242851768000023 ) ) ;
#21347=B_SPLINE_CURVE_WITH_KNOTS ( 'NONE', 3,
 ( #32936, #29387, #6965, #24686 ),
 .UNSPECIFIED., .F., .F.,
 ( 4, 4 ),
 ( 0.000000000000000000, 1.000000000000000000 ),
 .UNSPECIFIED. ) ;
#21350=CARTESIAN_POINT ( 'NONE',  ( -9.690626710582000314, -78.25169696010699738, -7.043281791253000357 ) ) ;
#21356=CARTESIAN_POINT ( 'NONE',  ( 2.866472250631999952, -78.17792964775300391, 10.89115702734000024 ) ) ;
#21358=CARTESIAN_POINT ( 'NONE',  ( -8.288807259790001325, -80.88254031229138263, -7.615077709626000058 ) ) ;
#21377=CARTESIAN_POINT ( 'NONE',  ( 0.1369776181910999924, -77.01514836410099463, 11.03100047655000004 ) ) ;
#21384=CARTESIAN_POINT ( 'NONE',  ( -4.634473952174339217, -80.18982139357595429, -9.715902795605705577 ) ) ;
#21386=CARTESIAN_POINT ( 'NONE',  ( -11.99999999994999911, -76.29999999994899440, 3.078392110872999642E-09 ) ) ;
#21388=CARTESIAN_POINT ( 'NONE',  ( 9.785129497364000173, -79.26670666393400211, -6.997026981537000090 ) ) ;
#21390=CARTESIAN_POINT ( 'NONE',  ( -9.845147265217999433, -79.36375811998600227, -5.468732932272000191 ) ) ;
#21413=EDGE_CURVE ( 'NONE', #40983, #49519, #22621, .T. ) ;
#21414=CARTESIAN_POINT ( 'NONE',  ( -3.411549236729638945, -80.00087276832812222, 10.19443305130964283 ) ) ;
#21422=CARTESIAN_POINT ( 'NONE',  ( 1.521043722421000055, -76.59490344678600593, -10.89349724765000005 ) ) ;
#21426=DIRECTION ( 'NONE',  ( 0.000000000000000000, -1.000000000000000000, 0.000000000000000000 ) ) ;
#21430=CARTESIAN_POINT ( 'NONE',  ( 1.483688553140142252, -80.96438982575540422, 10.64694122786772468 ) ) ;
#21434=CARTESIAN_POINT ( 'NONE',  ( 10.47020627418437932, -80.22916666666665719, -2.813789756862290492 ) ) ;
#21435=CARTESIAN_POINT ( 'NONE',  ( -9.797890753601748770, -79.25056356931708024, 7.009672782845666639 ) ) ;
#21453=CARTESIAN_POINT ( 'NONE',  ( -2.804788745061338240, -79.99636019303807188, 10.37822998189701806 ) ) ;
#21465=CARTESIAN_POINT ( 'NONE',  ( 0.4919088493939999807, -77.63064477680499920, 12.15485731165999894 ) ) ;
#21466=EDGE_LOOP ( 'NONE', ( #29889, #44934, #55744, #21965, #41871 ) ) ;
#21472=B_SPLINE_SURFACE_WITH_KNOTS ( 'NONE', 3, 3, ( 
 ( #34317, #7472, #11622, #25762, #43782, #33745, #7180, #43203, #29311, #12191, #56777, #3334, #29597, #47361, #30470, #21616, #47653, #21329, #16339, #20758, #8041, #11333, #52921, #2473, #42915, #25468, #34028, #34892, #34606, #48499, #48225, #56487, #16909, #7757, #51781, #39339, #52353, #43488, #25180, #57345, #12468, #6891, #2757, #38759, #24897, #26039, #11904, #44064, #3049, #20476, #3612, #39622, #21044, #57630, #39047, #57061, #16044, #52067, #36356, #44342, #3895, #49368, #13036, #49959, #13625, #27489, #12754 ),
 ( #13330, #5076, #48784, #23071, #53796, #31034, #35767, #8620, #41085, #17185, #44936, #40502, #39907, #21898, #98, #22192, #44643, #17777, #30750, #4196, #31623, #58215, #18073, #36067, #54087, #27195, #49666, #26605, #45235, #8328, #9209, #4782, #57920, #22784, #40792, #387, #56700, #15799, #24943, #7807, #57107, #48271, #11385, #47698, #29360, #30228, #56249, #43252, #34939, #21377, #39098, #56535, #56827, #25808, #25519, #2236, #43836, #20235, #47409, #3383, #2808, #16096, #12521, #52682, #39392, #7228, #20522 ),
 ( #38520, #47984, #8095, #29932, #7522, #11954, #38809, #12237, #57399, #30518, #48548, #43535, #38229, #25232, #3099, #34076, #33788, #11671, #20802, #51830, #6940, #42963, #2520, #16673, #21094, #52112, #16957, #34654, #29646, #26090, #16381, #34366, #52400, #21665, #9265, #31969, #13974, #44694, #17833, #17529, #4249, #26959, #35820, #22246, #49722, #40849, #22547, #40558, #441, #150, #26374, #57677, #9558, #53850, #50012, #44989, #54438, #49423, #27250, #44116, #39671, #18419, #30801, #3945, #13382, #31382, #8973 ),
 ( #40257, #18127, #35222, #31085, #53252, #12802, #58270, #4840, #17235, #3665, #4545, #57973, #36122, #44393, #48833, #8376, #54138, #13678, #21948, #39960, #31676, #49122, #13087, #45290, #35520, #8672, #22835, #26661, #36410, #53549, #41719, #37574, #10431, #1017, #55590, #15442, #46463, #28416, #1882, #15140, #42313, #50302, #10145, #41137, #9851, #33135, #23997, #51178, #36702, #14554, #54717, #10735, #23128, #28122, #19876, #46763, #5991, #23419, #23709, #28711, #50885, #27542, #6285, #45585, #14260, #24300, #46172 ) ),
 .UNSPECIFIED., .F., .F., .F.,
 ( 4, 4 ),
 ( 4, 1, 1, 1, 1, 1, 1, 1, 1, 1, 1, 1, 1, 1, 1, 1, 1, 1, 1, 1, 1, 1, 1, 1, 1, 1, 1, 1, 1, 1, 1, 1, 1, 1, 1, 1, 1, 1, 1, 1, 1, 1, 1, 1, 1, 1, 1, 1, 1, 1, 1, 1, 1, 1, 1, 1, 1, 1, 1, 1, 1, 1, 1, 1, 4 ),
 ( -0.1772706441294000235, 1.177270644128999955 ),
 ( -0.02000000000000000042, -0.003749999999999999861, 0.01250000000000000069, 0.02875000000000000125, 0.04499999999999999833, 0.06124999999999999889, 0.07749999999999999944, 0.09375000000000000000, 0.1100000000000000006, 0.1262500000000000011, 0.1424999999999999878, 0.1587500000000000022, 0.1749999999999999889, 0.1912500000000000033, 0.2074999999999999900, 0.2237500000000000044, 0.2399999999999999911, 0.2562499999999999778, 0.2725000000000000200, 0.2887500000000000067, 0.3049999999999999933, 0.3212499999999999800, 0.3375000000000000222, 0.3537500000000000089, 0.3699999999999999956, 0.3862499999999999822, 0.4025000000000000244, 0.4187500000000000111, 0.4349999999999999978, 0.4512499999999999845, 0.4675000000000000266, 0.4837500000000000133, 0.5000000000000000000, 0.5162499999999999867, 0.5324999999999999734, 0.5487499999999999600, 0.5649999999999999467, 0.5812500000000000444, 0.5975000000000000311, 0.6137500000000000178, 0.6300000000000000044, 0.6462499999999999911, 0.6624999999999999778, 0.6787499999999999645, 0.6949999999999999512, 0.7112500000000000488, 0.7275000000000000355, 0.7437500000000000222, 0.7600000000000000089, 0.7762499999999999956, 0.7924999999999999822, 0.8087499999999999689, 0.8249999999999999556, 0.8412500000000000533, 0.8575000000000000400, 0.8737500000000000266, 0.8900000000000000133, 0.9062500000000000000, 0.9224999999999999867, 0.9387499999999999734, 0.9549999999999999600, 0.9712499999999999467, 0.9875000000000000444, 1.003749999999999920, 1.020000000000000018 ),
 .UNSPECIFIED. ) ;
#21480=DIRECTION ( 'NONE',  ( 0.000000000000000000, -1.000000000000000000, 0.000000000000000000 ) ) ;
#21491=CARTESIAN_POINT ( 'NONE',  ( 5.459501886381000091, -76.15997619157100473, -11.00074850082999767 ) ) ;
#21500=CARTESIAN_POINT ( 'NONE',  ( 0.9868626873424000134, -78.00481147984399399, -12.24017488508000007 ) ) ;
#21505=CARTESIAN_POINT ( 'NONE',  ( -8.125470958442424063, -79.54330210541110091, 7.039620741617721222 ) ) ;
#21507=CARTESIAN_POINT ( 'NONE',  ( -12.00000000000000000, -78.89999999999999147, -1.868256502752000067E-14 ) ) ;
#21508=CARTESIAN_POINT ( 'NONE',  ( 7.657575756372000164, -79.51128919345099177, 9.292673803815999278 ) ) ;
#21536=CARTESIAN_POINT ( 'NONE',  ( 1.330647945963000067, -76.69316330962899997, 12.51808036622999865 ) ) ;
#21545=CARTESIAN_POINT ( 'NONE',  ( 10.29113596735999892, -77.53255742550288687, 4.462133020506000136 ) ) ;
#21556=CARTESIAN_POINT ( 'NONE',  ( 9.579193661067593624, -77.09808761060168081, -7.313663711862215422 ) ) ;
#21566=CARTESIAN_POINT ( 'NONE',  ( 11.00000000000000000, -76.04999999999999716, -1.235102163740000267E-09 ) ) ;
#21569=CARTESIAN_POINT ( 'NONE',  ( 1.407171709420391936, -77.86458333333330017, 10.75000000000000178 ) ) ;
#21574=CARTESIAN_POINT ( 'NONE',  ( -3.545645331619000196, -77.46501628338398859, 11.44309676683000099 ) ) ;
#21577=VECTOR ( 'NONE', #23159, 1000.000000000000000 ) ;
#21578=CARTESIAN_POINT ( 'NONE',  ( 10.14226539039000130, -78.37076856562599403, 6.290465419776000822 ) ) ;
#21586=CARTESIAN_POINT ( 'NONE',  ( -11.56229308710999959, -79.35377338295398886, -4.110692102696999584 ) ) ;
#21591=CARTESIAN_POINT ( 'NONE',  ( -11.42709289613000045, -75.91791632114400556, 3.432315517540000194 ) ) ;
#21593=CARTESIAN_POINT ( 'NONE',  ( 9.046072084723403961, -76.79619834608396900, 5.940455828180382980 ) ) ;
#21596=CARTESIAN_POINT ( 'NONE',  ( -5.360806944915999850, -79.79393910884799368, -9.773246618612999370 ) ) ;
#21610=CARTESIAN_POINT ( 'NONE',  ( 10.57259517296283491, -78.83558926200460348, -1.944988004412892657 ) ) ;
#21615=CARTESIAN_POINT ( 'NONE',  ( -10.47544694528181886, -81.00000000000000000, -2.552740764969549936 ) ) ;
#21616=CARTESIAN_POINT ( 'NONE',  ( 8.827997450462000018, -77.87345696174899956, 6.421979991006000255 ) ) ;
#21621=CARTESIAN_POINT ( 'NONE',  ( -1.780884232981000181, -79.87841764300529235, -11.07459082487999957 ) ) ;
#21622=ORIENTED_EDGE ( 'NONE', *, *, #6279, .T. ) ;
#21638=CARTESIAN_POINT ( 'NONE',  ( 7.547699635377999705, -79.68694304294899666, -9.585476548908999916 ) ) ;
#21647=CARTESIAN_POINT ( 'NONE',  ( 9.181220278661999856, -77.52425741570898765, -6.522205052974000772 ) ) ;
#21655=CARTESIAN_POINT ( 'NONE',  ( 4.013660496580000903, -78.35243718747800301, -10.47417304634999979 ) ) ;
#21661=AXIS2_PLACEMENT_3D ( 'NONE', #2957, #29226, #2105 ) ;
#21663=DIRECTION ( 'NONE',  ( 1.000000000000000000, 0.000000000000000000, 0.000000000000000000 ) ) ;
#21665=CARTESIAN_POINT ( 'NONE',  ( 8.145565103785999739, -77.51865691654299440, 7.609492079688000565 ) ) ;
#21671=CARTESIAN_POINT ( 'NONE',  ( -1.946241567991743304, -80.21069342602670815, -10.57240121655948606 ) ) ;
#21673=CARTESIAN_POINT ( 'NONE',  ( -2.813789756862251856, -77.10416666666665719, -10.47020627418439709 ) ) ;
#21676=CARTESIAN_POINT ( 'NONE',  ( 11.43764105185000091, -79.76670709676099591, 2.691257544168000226 ) ) ;
#21678=CARTESIAN_POINT ( 'NONE',  ( -4.036005110416000186, -79.22757640497698617, 10.51402051105999824 ) ) ;
#21679=CARTESIAN_POINT ( 'NONE',  ( -7.103581178201927138, -77.53231073429024889, 8.098573607620954462 ) ) ;
#21683=ORIENTED_EDGE ( 'NONE', *, *, #50667, .T. ) ;
#21686=DIRECTION ( 'NONE',  ( 0.000000000000000000, -1.000000000000000000, 0.000000000000000000 ) ) ;
#21687=CARTESIAN_POINT ( 'NONE',  ( -10.74525019809999904, -79.05928543398199793, 1.927424232126999870 ) ) ;
#21694=ORIENTED_EDGE ( 'NONE', *, *, #11702, .T. ) ;
#21706=CARTESIAN_POINT ( 'NONE',  ( -10.56721085596999998, -77.01377769904699733, 1.716300984214999881 ) ) ;
#21714=CARTESIAN_POINT ( 'NONE',  ( -1.429395846838289241, -80.98573564870306996, 10.65686433594883198 ) ) ;
#21722=CIRCLE ( 'NONE', #13241, 9.599999999999999645 ) ;
#21734=CARTESIAN_POINT ( 'NONE',  ( -1.552587846661832138, -79.98697443929660267, 10.63702038836880881 ) ) ;
#21742=ORIENTED_EDGE ( 'NONE', *, *, #38273, .T. ) ;
#21774=CARTESIAN_POINT ( 'NONE',  ( -0.6669403506045999963, -76.11899345326600042, -12.26286337364000012 ) ) ;
#21782=CARTESIAN_POINT ( 'NONE',  ( -9.053955183288000086, -77.07376637690499876, -6.099285168125999412 ) ) ;
#21783=CARTESIAN_POINT ( 'NONE',  ( -10.88187945745999841, -78.41175121120100755, -5.690384754473000406 ) ) ;
#21789=CARTESIAN_POINT ( 'NONE',  ( -5.015684137145860255, -79.51374401593871255, 9.508478352445903781 ) ) ;
#21792=CARTESIAN_POINT ( 'NONE',  ( 5.072393583102999592, -79.09961090260800631, 11.04742415471000072 ) ) ;
#21793=CARTESIAN_POINT ( 'NONE',  ( 6.689487621035000053, -80.75012225428049817, -8.802461778990000596 ) ) ;
#21795=CARTESIAN_POINT ( 'NONE',  ( 9.736961952457013680, -79.69999999999997442, 7.076710841379813210 ) ) ;
#21811=DIRECTION ( 'NONE',  ( -1.000000000000000000, 0.000000000000000000, 0.000000000000000000 ) ) ;
#21812=AXIS2_PLACEMENT_3D ( 'NONE', #52568, #42267, #38979 ) ;
#21820=VERTEX_POINT ( 'NONE', #5499 ) ;
#21822=CARTESIAN_POINT ( 'NONE',  ( 8.182584713298000523, -77.00851930215799257, 9.253818538989998288 ) ) ;
#21823=CARTESIAN_POINT ( 'NONE',  ( -10.45676550743384858, -78.61867176466869012, -2.493575623787820827 ) ) ;
#21829=CARTESIAN_POINT ( 'NONE',  ( -9.457500717944000712, -78.29517502955388863, -6.031068363571000290 ) ) ;
#21831=CARTESIAN_POINT ( 'NONE',  ( 10.12058791103999944, -79.68715863353600071, 4.836508133599999759 ) ) ;
#21847=CARTESIAN_POINT ( 'NONE',  ( -5.413904038987160661, -79.58333333333330017, -9.393203674808278336 ) ) ;
#21848=CARTESIAN_POINT ( 'NONE',  ( -11.20683111097000051, -79.75336693180456393, -0.4743912329535999728 ) ) ;
#21849=ORIENTED_EDGE ( 'NONE', *, *, #11702, .F. ) ;
#21857=CARTESIAN_POINT ( 'NONE',  ( -5.666254562607999645, -77.99095814969300022, 10.50376416711000083 ) ) ;
#21862=B_SPLINE_CURVE_WITH_KNOTS ( 'NONE', 3,
 ( #46858, #51571, #11128, #1984, #19979, #6386, #37966, #24690, #47151, #16413, #44148, #29677, #25837, #43567, #26128, #7262, #2836, #12552, #48015, #12834, #52715, #57429, #45242, #7550, #25262, #16990, #34970, #31631 ),
 .UNSPECIFIED., .F., .F.,
 ( 4, 2, 1, 2, 2, 1, 2, 2, 2, 2, 2, 2, 2, 2, 4 ),
 ( 0.000000000000000000, 0.1249999999999998612, 0.1874999999999997502, 0.2187499999999996669, 0.2499999999999996114, 0.3124999999999996114, 0.3437499999999996114, 0.3749999999999995559, 0.4999999999999996669, 0.5624999999999996669, 0.6249999999999997780, 0.6874999999999997780, 0.7499999999999997780, 0.8749999999999998890, 1.000000000000000000 ),
 .UNSPECIFIED. ) ;
#21873=CARTESIAN_POINT ( 'NONE',  ( -5.277198993124000204, -76.03111453605899328, -11.20659448217999987 ) ) ;
#21876=VERTEX_POINT ( 'NONE', #6084 ) ;
#21877=CARTESIAN_POINT ( 'NONE',  ( 8.767647372505999570, -80.01182985286258997, 6.883540450345000394 ) ) ;
#21882=CARTESIAN_POINT ( 'NONE',  ( 0.000000000000000000, -76.14999999999999147, -10.90000000000000036 ) ) ;
#21884=CARTESIAN_POINT ( 'NONE',  ( 8.480197680338001476, -78.51225130393000029, -8.881555409017000358 ) ) ;
#21887=CARTESIAN_POINT ( 'NONE',  ( 5.413904038987143785, -78.33333333333332860, 9.393203674808290771 ) ) ;
#21890=EDGE_LOOP ( 'NONE', ( #4407, #10513, #38400, #22188, #46992 ) ) ;
#21892=CARTESIAN_POINT ( 'NONE',  ( 10.59031137979719084, -78.83631738623206786, -1.847091933338027125 ) ) ;
#21898=CARTESIAN_POINT ( 'NONE',  ( 2.807878695492000087, -77.99565671216601004, 10.66853090226000056 ) ) ;
#21902=CARTESIAN_POINT ( 'NONE',  ( -11.04065564778000130, -79.18419320068699108, 1.980412446595999798 ) ) ;
#21904=VERTEX_POINT ( 'NONE', #36504 ) ;
#21920=CARTESIAN_POINT ( 'NONE',  ( -7.458578474212999687, -79.44721302158100684, -9.947846520260998915 ) ) ;
#21922=CARTESIAN_POINT ( 'NONE',  ( 11.70594025892000012, -78.46873148349699534, 2.546964289010999583 ) ) ;
#21929=CARTESIAN_POINT ( 'NONE',  ( 1.639991984446999895, -77.96003890373799550, -11.14201017990999887 ) ) ;
#21930=CARTESIAN_POINT ( 'NONE',  ( -12.00000000000000355, -78.28958333333331154, 1.570796326794848596 ) ) ;
#21948=CARTESIAN_POINT ( 'NONE',  ( 10.38236180178000012, -77.99492912598299199, -4.363545344708000151 ) ) ;
#21954=CARTESIAN_POINT ( 'NONE',  ( -4.109693089787123554, -80.19415985813694192, -9.933173281240437191 ) ) ;
#21956=CARTESIAN_POINT ( 'NONE',  ( 3.113304451009999863, -78.49783470746899638, -10.55022916317000181 ) ) ;
#21961=ADVANCED_FACE ( 'NONE', ( #533 ), #54381, .F. ) ;
#21962=CARTESIAN_POINT ( 'NONE',  ( 5.768896245881999896, -78.65561320193899064, 9.672321370914000127 ) ) ;
#21964=VERTEX_POINT ( 'NONE', #24092 ) ;
#21965=ORIENTED_EDGE ( 'NONE', *, *, #1941, .T. ) ;
#21967=ORIENTED_EDGE ( 'NONE', *, *, #4247, .F. ) ;
#21972=CARTESIAN_POINT ( 'NONE',  ( 8.677112325477001065, -79.94410278844959805, 6.812460760216000111 ) ) ;
#21992=CARTESIAN_POINT ( 'NONE',  ( 8.020449964080999194, -76.26883820092800192, 7.526900779542000208 ) ) ;
#21999=CARTESIAN_POINT ( 'NONE',  ( 6.252156853421744209, -77.46842338808832551, -10.30345392412948158 ) ) ;
#22000=CARTESIAN_POINT ( 'NONE',  ( -1.258323786088432650, -80.98444689146701592, 10.67706056211495813 ) ) ;
#22001=CARTESIAN_POINT ( 'NONE',  ( 3.862060628231000159, -80.74883687878880778, 10.58270681924999934 ) ) ;
#22019=CARTESIAN_POINT ( 'NONE',  ( 11.68767212001979239, -79.12916666666667709, -3.140974612311342451 ) ) ;
#22025=CARTESIAN_POINT ( 'NONE',  ( 1.900435629933197923, -77.23927092607918610, -10.60415385166746027 ) ) ;
#22032=CARTESIAN_POINT ( 'NONE',  ( -11.75000000000000000, -76.04999999999999716, -3.652443742841000169E-09 ) ) ;
#22036=CARTESIAN_POINT ( 'NONE',  ( 10.24006772854000147, -78.48531443679999597, 6.351124671173999481 ) ) ;
#22040=CARTESIAN_POINT ( 'NONE',  ( 12.00000000000000000, -76.64999999999999147, 0.000000000000000000 ) ) ;
#22045=CARTESIAN_POINT ( 'NONE',  ( 0.000000000000000000, -75.15999999999999659, 0.000000000000000000 ) ) ;
#22048=CARTESIAN_POINT ( 'NONE',  ( 12.00000000000000000, -77.54999999999999716, 0.000000000000000000 ) ) ;
#22051=CARTESIAN_POINT ( 'NONE',  ( -10.86788298907000083, -77.68455751383611130, -5.040355520269000245 ) ) ;
#22070=CARTESIAN_POINT ( 'NONE',  ( 2.778581917921999711, -78.38111084099200809, 10.55721783972000161 ) ) ;
#22071=CARTESIAN_POINT ( 'NONE',  ( -9.108185712014998714, -77.81490627187800158, 8.236305738405000909 ) ) ;
#22076=VERTEX_POINT ( 'NONE', #6523 ) ;
#22077=CARTESIAN_POINT ( 'NONE',  ( 4.484526869169065399, -78.74462836071080574, 11.18137712903838299 ) ) ;
#22078=CARTESIAN_POINT ( 'NONE',  ( 9.798978774566998950, -80.78509494028411098, -5.119823760639000909 ) ) ;
#22095=CARTESIAN_POINT ( 'NONE',  ( -1.570796326794885012, -76.91458333333332575, -12.00000000000000178 ) ) ;
#22103=VERTEX_POINT ( 'NONE', #7105 ) ;
#22111=CARTESIAN_POINT ( 'NONE',  ( -3.720841153849000271, -77.09048477876800121, 11.77893002587000026 ) ) ;
#22112=CARTESIAN_POINT ( 'NONE',  ( -10.44660810894644598, -78.61899168769637924, -2.535882402899716670 ) ) ;
#22120=CARTESIAN_POINT ( 'NONE',  ( 11.01642476344999899, -77.01506690846845515, 2.111041454437999842 ) ) ;
#22121=DIRECTION ( 'NONE',  ( -1.000000000000000000, 0.000000000000000000, 1.929499587357000000E-14 ) ) ;
#22123=CARTESIAN_POINT ( 'NONE',  ( -6.206245474241999460, -79.82334034854498839, 9.343480492029000217 ) ) ;
#22135=CARTESIAN_POINT ( 'NONE',  ( -12.17466003208999936, -76.69120375783900556, 1.612538369963999907 ) ) ;
#22136=CARTESIAN_POINT ( 'NONE',  ( 0.000000000000000000, -75.15999999999999659, 0.000000000000000000 ) ) ;
#22140=CARTESIAN_POINT ( 'NONE',  ( 6.233047529871999615, -78.98050366622999263, 9.960502923565000444 ) ) ;
#22142=AXIS2_PLACEMENT_3D ( 'NONE', #33499, #24065, #41491 ) ;
#22144=VERTEX_POINT ( 'NONE', #43705 ) ;
#22151=CARTESIAN_POINT ( 'NONE',  ( -11.44451898095999987, -78.09947541138799920, -3.385038809382000302 ) ) ;
#22156=CARTESIAN_POINT ( 'NONE',  ( 5.472379214682000281, -80.19337520226639526, -9.446080217779000421 ) ) ;
#22162=CARTESIAN_POINT ( 'NONE',  ( -11.21736175386999967, -79.85981236905720948, -4.975459846704000100 ) ) ;
#22167=CARTESIAN_POINT ( 'NONE',  ( -6.570942521484999688, -76.52164013402300213, -10.50046416013000083 ) ) ;
#22171=CARTESIAN_POINT ( 'NONE',  ( -10.17265785211000129, -78.60952198136099867, 4.268344714933999917 ) ) ;
#22179=CARTESIAN_POINT ( 'NONE',  ( 11.82394432951000063, -79.05483761240600415, -3.315134025842000121 ) ) ;
#22187=CARTESIAN_POINT ( 'NONE',  ( 10.72009390921250649, -78.84356995979068472, -0.8762394021455865989 ) ) ;
#22188=ORIENTED_EDGE ( 'NONE', *, *, #38962, .T. ) ;
#22192=CARTESIAN_POINT ( 'NONE',  ( 8.921077980507002181, -77.94118402616200569, 6.489691983999000158 ) ) ;
#22198=CARTESIAN_POINT ( 'NONE',  ( -8.382198119002001846, -79.82394495700170012, -7.453647783897999979 ) ) ;
#22215=CARTESIAN_POINT ( 'NONE',  ( 6.596971017208000276, -79.20390260564799689, 10.53897607326000063 ) ) ;
#22216=CARTESIAN_POINT ( 'NONE',  ( 0.000000000000000000, -87.20000000000000284, 0.000000000000000000 ) ) ;
#22217=CARTESIAN_POINT ( 'NONE',  ( -5.561497340033285219, -78.01840227481952184, 9.199883782775010843 ) ) ;
#22218=CARTESIAN_POINT ( 'NONE',  ( -3.545645331619000196, -77.60059338993599454, 11.44309676683000099 ) ) ;
#22223=CARTESIAN_POINT ( 'NONE',  ( 6.596840968109408898, -80.92259746458073266, 8.494723663472855790 ) ) ;
#22226=CARTESIAN_POINT ( 'NONE',  ( -9.340344124447998553, -76.87058518366599458, -6.292213870087999261 ) ) ;
#22228=CARTESIAN_POINT ( 'NONE',  ( -1.697681976669999981, -81.00396274871158653, -11.01068734798000115 ) ) ;
#22236=CARTESIAN_POINT ( 'NONE',  ( 10.68101746380904515, -76.86058654510705423, 1.407256982417045332 ) ) ;
#22242=CARTESIAN_POINT ( 'NONE',  ( -11.55514622889111465, -76.05000000000001137, 2.460715416399694266 ) ) ;
#22246=CARTESIAN_POINT ( 'NONE',  ( -9.936460025306999455, -77.24629348652399585, -5.051867252445999767 ) ) ;
#22252=CARTESIAN_POINT ( 'NONE',  ( -1.229427629842215985, -80.21594462373234080, -10.68102437834389207 ) ) ;
#22254=CARTESIAN_POINT ( 'NONE',  ( 0.9578449722871110739, -78.98171181572377009, -11.17605216401635637 ) ) ;
#22257=CARTESIAN_POINT ( 'NONE',  ( 2.188076007269000200, -78.68284954493999805, 11.04745617521000156 ) ) ;
#22265=B_SPLINE_CURVE_WITH_KNOTS ( 'NONE', 3,
 ( #28418, #51762, #56182, #21026, #38452, #11313, #39033, #33727, #22095, #20459, #35672, #34013, #7740, #52049, #29294, #29868, #17683, #56469 ),
 .UNSPECIFIED., .F., .F.,
 ( 4, 2, 2, 2, 2, 2, 2, 2, 4 ),
 ( 0.000000000000000000, 0.1250000000000000000, 0.2500000000000000000, 0.3750000000000000000, 0.5000000000000000000, 0.6250000000000000000, 0.7500000000000000000, 0.8750000000000000000, 1.000000000000000000 ),
 .UNSPECIFIED. ) ;
#22268=CARTESIAN_POINT ( 'NONE',  ( 10.97276992925000094, -79.39937592841299363, 1.140199307644999882 ) ) ;
#22273=CARTESIAN_POINT ( 'NONE',  ( 7.083715465317824922, -78.28195011990158036, -8.166873904374831739 ) ) ;
#22288=CARTESIAN_POINT ( 'NONE',  ( -1.910682550011000291, -76.63754856920999714, -10.71539657768000176 ) ) ;
#22295=CARTESIAN_POINT ( 'NONE',  ( 10.76566337430111275, -77.51291972185832435, -5.417667412981278297 ) ) ;
#22296=CARTESIAN_POINT ( 'NONE',  ( -0.9849936891751999157, -81.01971605282150790, -11.22225356808999841 ) ) ;
#22322=CARTESIAN_POINT ( 'NONE',  ( -2.739655911418338530, -77.20466484327231171, -10.39613826528414364 ) ) ;
#22325=ORIENTED_EDGE ( 'NONE', *, *, #11767, .T. ) ;
#22326=AXIS2_PLACEMENT_3D ( 'NONE', #51806, #6629, #24637 ) ;
#22328=CARTESIAN_POINT ( 'NONE',  ( 11.77452260639999970, -79.96011154630718920, 1.259536412044000020 ) ) ;
#22333=CARTESIAN_POINT ( 'NONE',  ( 11.77424395174999994, -78.45818512137599043, 2.561825723684000078 ) ) ;
#22338=CARTESIAN_POINT ( 'NONE',  ( 11.92322513370752191, -76.63885875642324663, -1.571131804317056568 ) ) ;
#22356=TOROIDAL_SURFACE ( 'NONE', #706, 9.799999999999998934, 0.2000000000000000111 ) ;
#22373=CARTESIAN_POINT ( 'NONE',  ( 2.897215155706000189, -77.67296592294499646, -10.52527958449999979 ) ) ;
#22374=CARTESIAN_POINT ( 'NONE',  ( -12.11185258877999971, -77.44856428951000282, -1.133824260204999934 ) ) ;
#22377=CARTESIAN_POINT ( 'NONE',  ( 2.813789756862274505, -79.14583333333331439, -10.47020627418438821 ) ) ;
#22382=CARTESIAN_POINT ( 'NONE',  ( -8.708695699441999949, -79.68326480666600276, -8.148281476810998569 ) ) ;
#22383=CARTESIAN_POINT ( 'NONE',  ( -5.726205896150999841, -80.22331365663170288, -9.593452009017001458 ) ) ;
#22385=CARTESIAN_POINT ( 'NONE',  ( 0.000000000000000000, -87.25000000009099210, 0.000000000000000000 ) ) ;
#22386=CARTESIAN_POINT ( 'NONE',  ( -9.302864017704999711, -76.88107005692299367, -6.266965030821000759 ) ) ;
#22396=CARTESIAN_POINT ( 'NONE',  ( 10.75000000000000000, -80.84999999999999432, -1.053639850055999980E-14 ) ) ;
#22400=CARTESIAN_POINT ( 'NONE',  ( -9.599999999916001059, -90.40000000008399184, 6.531558194539000517E-10 ) ) ;
#22407=FILL_AREA_STYLE_COLOUR ( '', #47341 ) ;
#22412=CARTESIAN_POINT ( 'NONE',  ( 11.09583276434000076, -76.40801663978099612, 5.154565694333999915 ) ) ;
#22420=CARTESIAN_POINT ( 'NONE',  ( 11.19180402071999936, -77.50532108250102681, 0.7494220128532999015 ) ) ;
#22422=CARTESIAN_POINT ( 'NONE',  ( -4.019809786096000259, -79.30584983151099721, 10.47183077952999852 ) ) ;
#22433=CARTESIAN_POINT ( 'NONE',  ( -0.6669403506045999963, -76.32235911309500409, -12.26286337364000012 ) ) ;
#22438=CARTESIAN_POINT ( 'NONE',  ( 7.910349975595998728, -79.56271253079168559, 7.952639426948999279 ) ) ;
#22440=EDGE_CURVE ( 'NONE', #7885, #56550, #38092, .T. ) ;
#22445=CARTESIAN_POINT ( 'NONE',  ( 6.444980599754999595, -77.66852088434498569, -10.09843005143000028 ) ) ;
#22448=CARTESIAN_POINT ( 'NONE',  ( 3.237243043699999934, -78.72344966613400175, -11.48719983142999901 ) ) ;
#22453=CARTESIAN_POINT ( 'NONE',  ( 10.21235917355000034, -80.24784788827008697, -3.857859667932999947 ) ) ;
#22458=CARTESIAN_POINT ( 'NONE',  ( -1.807666384373000090, -79.87198619718679993, -12.02113240485999945 ) ) ;
#22462=CARTESIAN_POINT ( 'NONE',  ( 10.20634188032000012, -76.21203981538700134, -6.810150128040000084 ) ) ;
#22464=DIRECTION ( 'NONE',  ( 0.000000000000000000, 0.000000000000000000, -1.000000000000000000 ) ) ;
#22466=CARTESIAN_POINT ( 'NONE',  ( -7.362671760698999535, -79.27644859181400250, -8.369328833011000057 ) ) ;
#22474=CARTESIAN_POINT ( 'NONE',  ( -7.229432123683867673, -76.43333333333332291, 8.035240866938302418 ) ) ;
#22476=CARTESIAN_POINT ( 'NONE',  ( 0.9868626873424000134, -78.45799267308299818, -12.24017488508000007 ) ) ;
#22481=( NAMED_UNIT ( * ) PLANE_ANGLE_UNIT ( ) SI_UNIT ( $, .RADIAN. ) );
#22496=CARTESIAN_POINT ( 'NONE',  ( -0.2721098858049000313, -79.07524782868000557, 11.21356619464000026 ) ) ;
#22516=CARTESIAN_POINT ( 'NONE',  ( -3.843694318990999559, -79.27341986734299439, 11.82438401172999853 ) ) ;
#22517=CARTESIAN_POINT ( 'NONE',  ( 1.582175077527999907, -76.41246662722099359, -11.50424973215999991 ) ) ;
#22518=CARTESIAN_POINT ( 'NONE',  ( -6.074904069602191647, -78.02296353543388818, 8.868935607531122756 ) ) ;
#22520=CARTESIAN_POINT ( 'NONE',  ( -4.743879332790999825, -78.72649471530600351, -11.00053059214000051 ) ) ;
#22527=CARTESIAN_POINT ( 'NONE',  ( 6.393694643109999909, -77.56474813712100058, -9.131005934809000024 ) ) ;
#22529=CARTESIAN_POINT ( 'NONE',  ( 7.370453364210000302, -80.64212683706639950, -8.200218203919000359 ) ) ;
#22536=CARTESIAN_POINT ( 'NONE',  ( -0.8253947190445000137, -77.31745615340899747, -11.18645762290999990 ) ) ;
#22545=CARTESIAN_POINT ( 'NONE',  ( -3.630949683904999947, -76.04999999999999716, 11.17491406647000041 ) ) ;
#22547=CARTESIAN_POINT ( 'NONE',  ( -9.465408641230000697, -77.16458445751899831, 5.887328751257999926 ) ) ;
#22554=CARTESIAN_POINT ( 'NONE',  ( 1.407171709420440342, -77.13541666666665719, -10.74999999999999822 ) ) ;
#22555=CARTESIAN_POINT ( 'NONE',  ( 6.766496333857535461, -79.52643867575977765, -8.946291764058088347 ) ) ;
#22556=VECTOR ( 'NONE', #55470, 1000.000000000000000 ) ;
#22560=CARTESIAN_POINT ( 'NONE',  ( 6.724228645090999379, -79.56766689940799608, -8.890407735272999545 ) ) ;
#22587=CARTESIAN_POINT ( 'NONE',  ( 7.362589990311000143, -76.14342849098198940, -7.926760118590000737 ) ) ;
#22590=CARTESIAN_POINT ( 'NONE',  ( -8.418594644163000851, -80.89173212753800613, -7.485750452785000064 ) ) ;
#22599=CARTESIAN_POINT ( 'NONE',  ( -4.454457568640999732, -80.80903225079606500, 10.34731867136000005 ) ) ;
#22609=FACE_OUTER_BOUND ( 'NONE', #42687, .T. ) ;
#22621=B_SPLINE_CURVE_WITH_KNOTS ( 'NONE', 3,
 ( #53787, #26899, #18064, #36057, #27185, #45225, #46110, #23934, #32196, #1522, #28943, #41952, #32484, #28650, #46986, #19515, #37510, #33372 ),
 .UNSPECIFIED., .F., .F.,
 ( 4, 2, 2, 2, 2, 2, 2, 2, 4 ),
 ( 0.000000000000000000, 0.1249999999999999722, 0.2499999999999999445, 0.3749999999999998890, 0.4999999999999998890, 0.6249999999999998890, 0.7499999999999997780, 0.8749999999999998890, 1.000000000000000000 ),
 .UNSPECIFIED. ) ;
#22624=CARTESIAN_POINT ( 'NONE',  ( 0.2747012913232428910, -77.22714148007511881, -10.74666282699171838 ) ) ;
#22626=ORIENTED_EDGE ( 'NONE', *, *, #5557, .T. ) ;
#22629=B_SPLINE_CURVE_WITH_KNOTS ( 'NONE', 3,
 ( #21507, #35061, #16510, #38933, #25930, #57235, #39222, #52809, #3790, #43957, #56951, #8505, #12648, #25357, #48676, #22077, #52522, #39796 ),
 .UNSPECIFIED., .F., .F.,
 ( 4, 2, 2, 2, 2, 2, 2, 2, 4 ),
 ( 0.000000000000000000, 0.1249999999999998890, 0.2499999999999998335, 0.3749999999999997780, 0.4999999999999997780, 0.6249999999999997780, 0.7499999999999997780, 0.8749999999999998890, 1.000000000000000000 ),
 .UNSPECIFIED. ) ;
#22632=CARTESIAN_POINT ( 'NONE',  ( -10.07076617545328467, -80.47065289228903850, 3.889019895268755356 ) ) ;
#22634=CARTESIAN_POINT ( 'NONE',  ( 12.04731061283000138, -77.94272812832399211, 0.2409951698105000095 ) ) ;
#22637=ORIENTED_EDGE ( 'NONE', *, *, #9082, .F. ) ;
#22640=EDGE_CURVE ( 'NONE', #19148, #18069, #7233, .T. ) ;
#22641=CARTESIAN_POINT ( 'NONE',  ( -9.541585721800542430, -76.45157166904904500, -7.319559354884466629 ) ) ;
#22645=ORIENTED_EDGE ( 'NONE', *, *, #9988, .F. ) ;
#22652=CARTESIAN_POINT ( 'NONE',  ( 6.060555231919183328, -77.31796419498604678, -10.11800260501370730 ) ) ;
#22665=DIRECTION ( 'NONE',  ( 0.000000000000000000, -1.000000000000000000, 0.000000000000000000 ) ) ;
#22673=CARTESIAN_POINT ( 'NONE',  ( 10.89987286286000057, -78.27216546898499416, -0.6067434084558999130 ) ) ;
#22675=CARTESIAN_POINT ( 'NONE',  ( -10.11841891201000010, -77.39430565866300071, 6.752786780719000070 ) ) ;
#22682=CARTESIAN_POINT ( 'NONE',  ( 3.695666939335999768, -80.22553196422599342, -10.41991477582000059 ) ) ;
#22691=ORIENTED_EDGE ( 'NONE', *, *, #49273, .T. ) ;
#22693=LINE ( 'NONE', #28567, #54279 ) ;
#22696=CARTESIAN_POINT ( 'NONE',  ( 2.264809212410999647E-14, -92.79999999999999716, 0.000000000000000000 ) ) ;
#22700=AXIS2_PLACEMENT_3D ( 'NONE', #55300, #51180, #32840 ) ;
#22708=VERTEX_POINT ( 'NONE', #34372 ) ;
#22709=CARTESIAN_POINT ( 'NONE',  ( 4.281740904750999555, -76.77686128452499759, -11.46096623826999839 ) ) ;
#22710=CARTESIAN_POINT ( 'NONE',  ( -9.586068793935504928, -78.63753982021442823, -4.864924515320017129 ) ) ;
#22717=CARTESIAN_POINT ( 'NONE',  ( -3.244487197725999916, -76.85164885045787742, -10.73738397614000029 ) ) ;
#22722=ORIENTED_EDGE ( 'NONE', *, *, #21413, .F. ) ;
#22730=CARTESIAN_POINT ( 'NONE',  ( 3.090997446795999970, -77.34692757071799463, -11.88544462247999967 ) ) ;
#22747=CARTESIAN_POINT ( 'NONE',  ( -0.4035379437255999791, -79.64864834222998979, -10.90928609572000063 ) ) ;
#22752=CARTESIAN_POINT ( 'NONE',  ( -10.75000000000000355, -77.48958333333332860, 1.407171709420384609 ) ) ;
#22756=CARTESIAN_POINT ( 'NONE',  ( -12.00000000000000000, -77.89999999999999147, -2.795183092923000262E-14 ) ) ;
#22761=CARTESIAN_POINT ( 'NONE',  ( -11.25198206936999945, -79.77995714425598806, -0.4763024974861999605 ) ) ;
#22764=EDGE_CURVE ( 'NONE', #35854, #55147, #35227, .T. ) ;
#22767=ADVANCED_FACE ( 'NONE', ( #13388 ), #30792, .T. ) ;
#22768=CARTESIAN_POINT ( 'NONE',  ( 7.229432123684064848, -76.31666666666667709, 8.035240866938130111 ) ) ;
#22781=CARTESIAN_POINT ( 'NONE',  ( -5.279550234765999939, -76.33587572314411318, -9.859017853534000508 ) ) ;
#22784=CARTESIAN_POINT ( 'NONE',  ( 8.061453700986000115, -77.45092985212998826, 7.530916186516999566 ) ) ;
#22788=CARTESIAN_POINT ( 'NONE',  ( 4.653115705712000505, -78.92514563794199489, -10.20620521156999949 ) ) ;
#22792=ORIENTED_EDGE ( 'NONE', *, *, #39537, .F. ) ;
#22808=CARTESIAN_POINT ( 'NONE',  ( -0.5565216587110000113, -78.88749453345599250, 12.18770865518000157 ) ) ;
#22809=CARTESIAN_POINT ( 'NONE',  ( -5.797379302154999969, -76.05869307850399252, 9.786931085294000354 ) ) ;
#22810=CARTESIAN_POINT ( 'NONE',  ( -4.117775072621233434, -78.00630082584859792, 9.930058322751628808 ) ) ;
#22811=CARTESIAN_POINT ( 'NONE',  ( -1.835125225091999823, -78.02113251428799856, 11.83842809849000055 ) ) ;
#22816=CARTESIAN_POINT ( 'NONE',  ( 6.297347977225174809, -80.92545155199817941, 8.712196151594245208 ) ) ;
#22819=CARTESIAN_POINT ( 'NONE',  ( 6.290530912463999869, -78.21842036916400787, 9.202381290206000486 ) ) ;
#22820=CARTESIAN_POINT ( 'NONE',  ( 1.570796326794857478, -78.16458333333332575, 12.00000000000000533 ) ) ;
#22821=CARTESIAN_POINT ( 'NONE',  ( -8.998761386569000820, -80.50788840704829852, -6.370985394032000926 ) ) ;
#22826=CARTESIAN_POINT ( 'NONE',  ( -5.859445663532000914, -77.61705592642898921, 9.564779511708000115 ) ) ;
#22833=CARTESIAN_POINT ( 'NONE',  ( -8.782705134682748493, -76.05000000000001137, 7.901937436400075399 ) ) ;
#22835=CARTESIAN_POINT ( 'NONE',  ( -11.26188033092999952, -77.77703838196799779, -0.06337168221170999538 ) ) ;
#22850=CARTESIAN_POINT ( 'NONE',  ( 8.500810681529999968, -80.08515741644239938, -7.210465973013999275 ) ) ;
#22863=CIRCLE ( 'NONE', #21008, 9.760776772971999193 ) ;
#22878=CARTESIAN_POINT ( 'NONE',  ( 10.80179710294999929, -76.28640138136300664, 1.338497018408000061 ) ) ;
#22881=CARTESIAN_POINT ( 'NONE',  ( -0.3187246912203000049, -80.71114601151622026, 11.26088853021000169 ) ) ;
#22887=FACE_BOUND ( 'NONE', #37183, .T. ) ;
#22888=CARTESIAN_POINT ( 'NONE',  ( 10.78853149093999875, -80.56065758149809142, -3.242959171380999983 ) ) ;
#22899=CARTESIAN_POINT ( 'NONE',  ( -6.290935915195801975, -79.52477021992575601, 8.717027692168942465 ) ) ;
#22915=CARTESIAN_POINT ( 'NONE',  ( -3.256966265956249273, -77.20063234487528803, -10.24510830600284628 ) ) ;
#22919=ORIENTED_EDGE ( 'NONE', *, *, #51521, .T. ) ;
#22920=CARTESIAN_POINT ( 'NONE',  ( -12.02912753549999891, -79.70112007896199202, 0.08506824670321999626 ) ) ;
#22922=CARTESIAN_POINT ( 'NONE',  ( 5.642595794959916589, -80.33125413066214549, 9.203581900605376731 ) ) ;
#22924=CARTESIAN_POINT ( 'NONE',  ( 3.947980971697000019, -78.53957306764699808, 11.38460442531999917 ) ) ;
#22930=CARTESIAN_POINT ( 'NONE',  ( -1.571007341338103158, -76.51400069817373151, -12.00174526218152593 ) ) ;
#22935=ORIENTED_EDGE ( 'NONE', *, *, #32881, .T. ) ;
#22946=CARTESIAN_POINT ( 'NONE',  ( -11.06076315228000340, -78.11862656061613563, 4.601693484369000053 ) ) ;
#22950=CYLINDRICAL_SURFACE ( 'NONE', #3179, 9.599999999999999645 ) ;
#22959=EDGE_CURVE ( 'NONE', #42525, #45004, #33140, .T. ) ;
#22961=CARTESIAN_POINT ( 'NONE',  ( -10.75000000000000000, -78.10000000000000853, 0.000000000000000000 ) ) ;
#22977=CARTESIAN_POINT ( 'NONE',  ( 2.308634773277999930, -80.71514956827684273, -10.81215905564999957 ) ) ;
#23000=AXIS2_PLACEMENT_3D ( 'NONE', #830, #36223, #40660 ) ;
#23002=CARTESIAN_POINT ( 'NONE',  ( -10.81540289212000161, -76.16212020995099863, -5.719638876297000074 ) ) ;
#23021=CARTESIAN_POINT ( 'NONE',  ( -3.699256142337000064, -77.10103114088899190, 11.71059914860999918 ) ) ;
#23031=CARTESIAN_POINT ( 'NONE',  ( -8.885616033064000163, -77.93981403858299473, 8.035041515002001589 ) ) ;
#23033=CARTESIAN_POINT ( 'NONE',  ( 2.241689414777999989, -77.86897245443199722, 11.83936654731000004 ) ) ;
#23037=CARTESIAN_POINT ( 'NONE',  ( -10.11939726227999969, -80.05719348725739337, -4.095505467953000078 ) ) ;
#23039=ORIENTED_EDGE ( 'NONE', *, *, #10974, .F. ) ;
#23043=CARTESIAN_POINT ( 'NONE',  ( -1.407171709420465211, -77.38541666666665719, 10.74999999999999467 ) ) ;
#23046=DIRECTION ( 'NONE',  ( -3.552713678800000476E-14, -1.000000000000000000, -5.625129991434000464E-14 ) ) ;
#23050=CARTESIAN_POINT ( 'NONE',  ( -5.416162833245999231, -79.86166617326099981, -9.874165520190000933 ) ) ;
#23052=CARTESIAN_POINT ( 'NONE',  ( 9.750701472721992502, -79.75205468146413068, -6.704702372767138208 ) ) ;
#23066=CARTESIAN_POINT ( 'NONE',  ( 10.05419478484149209, -78.82130372894751247, -3.806463643893830184 ) ) ;
#23071=CARTESIAN_POINT ( 'NONE',  ( 0.2611009988844999463, -78.26802014218399961, -11.02876811737000118 ) ) ;
#23073=CARTESIAN_POINT ( 'NONE',  ( 10.14802651313347681, -76.25255601911207748, -6.771239379213880305 ) ) ;
#23074=CARTESIAN_POINT ( 'NONE',  ( -7.167702442858890244, -77.47594342440135051, 9.599168351470673599 ) ) ;
#23075=CARTESIAN_POINT ( 'NONE',  ( 11.21485848424000054, -80.08238791129060985, -0.2123177049684000228 ) ) ;
#23076=CARTESIAN_POINT ( 'NONE',  ( 9.313025180101760725, -81.00000000000001421, 5.731444158754912088 ) ) ;
#23079=CARTESIAN_POINT ( 'NONE',  ( 2.853743189567553630E-14, -82.09999999999999432, -10.25000000000000000 ) ) ;
#23099=CARTESIAN_POINT ( 'NONE',  ( 11.77091756615000051, -79.16735377751798808, -3.626500858022000173 ) ) ;
#23100=CARTESIAN_POINT ( 'NONE',  ( -5.736890744663000419, -75.99096601409100060, 9.684816437834999903 ) ) ;
#23101=CARTESIAN_POINT ( 'NONE',  ( 5.302235052053965170, -77.93411949478270628, 9.360072782316642304 ) ) ;
#23102=CARTESIAN_POINT ( 'NONE',  ( 8.272973658470998970, -78.31955498394898996, -8.664523719228998999 ) ) ;
#23107=CARTESIAN_POINT ( 'NONE',  ( 6.281390822460244827, -80.92560318168439437, 8.723718198624005993 ) ) ;
#23110=CARTESIAN_POINT ( 'NONE',  ( -6.618456890295999706, -76.96554859108100288, -8.969427176287000592 ) ) ;
#23112=CARTESIAN_POINT ( 'NONE',  ( 2.021665076779000092, -81.09853749912809917, -10.83880671474999957 ) ) ;
#23117=CARTESIAN_POINT ( 'NONE',  ( 2.976864594307000011, -77.34469249641099964, -10.81463766284999828 ) ) ;
#23118=DIRECTION ( 'NONE',  ( 1.000000000000000000, 0.000000000000000000, 0.000000000000000000 ) ) ;
#23128=CARTESIAN_POINT ( 'NONE',  ( 9.707899084501001141, -77.06889346392100038, 5.708822989341999943 ) ) ;
#23134=B_SPLINE_CURVE_WITH_KNOTS ( 'NONE', 3,
 ( #5404, #14546, #32538, #13671 ),
 .UNSPECIFIED., .F., .F.,
 ( 4, 4 ),
 ( 0.000000000000000000, 1.000000000000000000 ),
 .UNSPECIFIED. ) ;
#23141=CARTESIAN_POINT ( 'NONE',  ( -11.24501830132000002, -78.81903125994999471, 0.6192963436278000611 ) ) ;
#23153=CARTESIAN_POINT ( 'NONE',  ( -7.374560639698971798, -76.37291666663053036, -9.596002108778163731 ) ) ;
#23159=DIRECTION ( 'NONE',  ( 0.000000000000000000, -1.000000000000000000, 9.177843670233999678E-14 ) ) ;
#23168=STYLED_ITEM ( 'NONE', ( #43229 ), #36141 ) ;
#23174=CARTESIAN_POINT ( 'NONE',  ( -9.578166812159000898, -80.22198985418920358, 5.930253639820000089 ) ) ;
#23177=CARTESIAN_POINT ( 'NONE',  ( 11.58335411283808902, -76.19322916655099220, -3.113814941787591994 ) ) ;
#23185=ORIENTED_EDGE ( 'NONE', *, *, #13106, .T. ) ;
#23192=CARTESIAN_POINT ( 'NONE',  ( -7.605077663679784550, -79.53769900547050042, 7.597564707201073908 ) ) ;
#23193=DIRECTION ( 'NONE',  ( 0.000000000000000000, 1.000000000000000000, 0.000000000000000000 ) ) ;
#23206=CARTESIAN_POINT ( 'NONE',  ( -3.830267234649249897, -77.19605609133061819, -10.04658309097634650 ) ) ;
#23209=ORIENTED_EDGE ( 'NONE', *, *, #19142, .F. ) ;
#23214=CARTESIAN_POINT ( 'NONE',  ( -10.93129665128000028, -77.72569360493399415, -5.069765792968000007 ) ) ;
#23218=ADVANCED_FACE ( 'NONE', ( #31310 ), #49649, .F. ) ;
#23223=CARTESIAN_POINT ( 'NONE',  ( -7.320008597215652557, -76.47238134542388366, -9.541710111217275525 ) ) ;
#23225=ORIENTED_EDGE ( 'NONE', *, *, #48378, .F. ) ;
#23229=CARTESIAN_POINT ( 'NONE',  ( -6.606377239730330864, -80.57291666666665719, -8.596418555780440229 ) ) ;
#23233=CARTESIAN_POINT ( 'NONE',  ( -7.695020077040999773, -76.13370154875299534, 8.115451295621999961 ) ) ;
#23259=CARTESIAN_POINT ( 'NONE',  ( 10.73158301355000077, -77.16380270170699873, 5.968995448363000556 ) ) ;
#23264=ORIENTED_EDGE ( 'NONE', *, *, #9288, .T. ) ;
#23267=CARTESIAN_POINT ( 'NONE',  ( 10.70141235895999898, -79.33702760564798950, -5.264563250036999875 ) ) ;
#23268=CARTESIAN_POINT ( 'NONE',  ( 5.141835936095000115, -80.04623191901920620, 10.04998108304999782 ) ) ;
#23272=DIRECTION ( 'NONE',  ( 0.000000000000000000, -1.000000000000000000, 0.000000000000000000 ) ) ;
#23317=CARTESIAN_POINT ( 'NONE',  ( 11.75000000000000000, -79.79999999999999716, -4.009019365174000020E-13 ) ) ;
#23330=CARTESIAN_POINT ( 'NONE',  ( 3.947980971697000019, -78.35730013205999001, 11.38460442531999917 ) ) ;
#23333=CARTESIAN_POINT ( 'NONE',  ( 4.576365007000999796, -79.11790344678600206, -10.03785921918999868 ) ) ;
#23335=VERTEX_POINT ( 'NONE', #19807 ) ;
#23340=CARTESIAN_POINT ( 'NONE',  ( 6.084904940690000430, -76.03885294825599317, -10.92373034159999889 ) ) ;
#23344=VERTEX_POINT ( 'NONE', #9780 ) ;
#23345=CARTESIAN_POINT ( 'NONE',  ( 3.485296502184999756, -79.05855784779899409, 10.58807389768000107 ) ) ;
#23347=CARTESIAN_POINT ( 'NONE',  ( -5.664454919952616407, -79.46458300272750819, 10.39013350000020530 ) ) ;
#23361=ORIENTED_EDGE ( 'NONE', *, *, #51521, .F. ) ;
#23364=CARTESIAN_POINT ( 'NONE',  ( 9.888817398439529782, -78.81797029978375235, -4.217298846466132289 ) ) ;
#23371=CARTESIAN_POINT ( 'NONE',  ( 11.53516957136256416, -78.77815056474238986, -3.234168909645118717 ) ) ;
#23372=CARTESIAN_POINT ( 'NONE',  ( 2.039250879084999912, -79.97344253928329749, -11.02993955029000084 ) ) ;
#23373=CARTESIAN_POINT ( 'NONE',  ( 8.136205013521058405, -81.00000000000001421, 7.261636552250462451 ) ) ;
#23380=CARTESIAN_POINT ( 'NONE',  ( 10.81758370320302731, -76.05000000000001137, 2.303648476915329368 ) ) ;
#23382=CARTESIAN_POINT ( 'NONE',  ( 10.48543666025110355, -77.60833333333330586, -6.043427764450775008 ) ) ;
#23391=CARTESIAN_POINT ( 'NONE',  ( -12.12831959444000063, -78.89107492802000365, -2.737500678952999422 ) ) ;
#23392=CARTESIAN_POINT ( 'NONE',  ( 8.153967731313999323, -76.38394096989499360, 7.760240090419999959 ) ) ;
#23393=CARTESIAN_POINT ( 'NONE',  ( 10.45286035002862768, -77.86879287204392597, 2.509877197284648975 ) ) ;
#23394=CARTESIAN_POINT ( 'NONE',  ( -8.148905501844000199, -78.63157684660600921, -8.781309899900000104 ) ) ;
#23403=CARTESIAN_POINT ( 'NONE',  ( 11.12204776531999961, -77.64645716612598392, 0.7447510167176000229 ) ) ;
#23405=CARTESIAN_POINT ( 'NONE',  ( 7.367354511904000702, -80.70863820267163646, 8.356990619368000139 ) ) ;
#23409=CARTESIAN_POINT ( 'NONE',  ( -4.647088938219000376, -78.17509865373799016, 10.20895072913000057 ) ) ;
#23419=CARTESIAN_POINT ( 'NONE',  ( 4.292950718366999929, -76.93271174891199848, -10.41175003194000048 ) ) ;
#23432=CARTESIAN_POINT ( 'NONE',  ( 4.703593957913000168, -79.79881202183199207, 9.978874598900000947 ) ) ;
#23438=VERTEX_POINT ( 'NONE', #47102 ) ;
#23448=CARTESIAN_POINT ( 'NONE',  ( 6.486170634443213956, -79.97433694125503223, 8.676707126471709941 ) ) ;
#23459=CARTESIAN_POINT ( 'NONE',  ( -2.612980907336999614, -80.37247828420728979, -10.95817168551000087 ) ) ;
#23460=CARTESIAN_POINT ( 'NONE',  ( -6.043427764450832740, -76.71666666666666856, 10.48543666025107512 ) ) ;
#23461=CARTESIAN_POINT ( 'NONE',  ( -12.00000000000000000, -79.39999999999999147, 0.000000000000000000 ) ) ;
#23476=CARTESIAN_POINT ( 'NONE',  ( 5.932307977941824184, -79.42851911752600813, 8.979481857698141667 ) ) ;
#23480=CYLINDRICAL_SURFACE ( 'NONE', #22142, 10.75000000000000000 ) ;
#23491=CARTESIAN_POINT ( 'NONE',  ( -7.597510670570571278, -77.16254964678856254, -7.605260874623661849 ) ) ;
#23495=CARTESIAN_POINT ( 'NONE',  ( -8.734850699938000673, -79.57356426399098837, 8.271005326623001253 ) ) ;
#23496=EDGE_CURVE ( 'NONE', #51603, #7386, #57225, .T. ) ;
#23499=DIRECTION ( 'NONE',  ( 0.000000000000000000, -1.000000000000000000, 0.000000000000000000 ) ) ;
#23514=CARTESIAN_POINT ( 'NONE',  ( 2.813789756862274505, -80.64583333333331439, -10.47020627418438821 ) ) ;
#23519=DIRECTION ( 'NONE',  ( 0.000000000000000000, 1.000000000000000000, 0.000000000000000000 ) ) ;
#23520=CARTESIAN_POINT ( 'NONE',  ( -1.660522255173999984, -76.65296505783298642, 11.05968181062000077 ) ) ;
#23522=CARTESIAN_POINT ( 'NONE',  ( -1.438191329984999989, -76.20862989806899179, 11.13621724565999926 ) ) ;
#23541=ADVANCED_FACE ( 'NONE', ( #51522 ), #44113, .F. ) ;
#23550=CARTESIAN_POINT ( 'NONE',  ( 6.830552694284000026, -80.88557638310635411, -8.988084353687998629 ) ) ;
#23553=CARTESIAN_POINT ( 'NONE',  ( 1.508420534579999917, -77.76594890025400275, 11.11497989572000122 ) ) ;
#23558=CARTESIAN_POINT ( 'NONE',  ( 4.810664641798661378, -79.80000000000001137, -10.79160144070993610 ) ) ;
#23559=CARTESIAN_POINT ( 'NONE',  ( 2.295494558656228534, -76.08645833332937514, 10.78189851169432956 ) ) ;
#23580=FACE_OUTER_BOUND ( 'NONE', #382, .T. ) ;
#23594=CARTESIAN_POINT ( 'NONE',  ( -10.47020627418439354, -77.52083333333331439, -2.813789756862263847 ) ) ;
#23600=CARTESIAN_POINT ( 'NONE',  ( 1.298131932841000147, -76.43267843637200087, 12.21218573294999921 ) ) ;
#23613=CARTESIAN_POINT ( 'NONE',  ( 11.27339212957999948, -77.78758450816098957, 4.255161755617000274 ) ) ;
#23620=( GEOMETRIC_REPRESENTATION_CONTEXT ( 3 ) GLOBAL_UNCERTAINTY_ASSIGNED_CONTEXT ( ( #46722 ) ) GLOBAL_UNIT_ASSIGNED_CONTEXT ( ( #31315, #22481, #36056 ) ) REPRESENTATION_CONTEXT ( 'NONE', 'WORKASPACE' ) );
#23627=CARTESIAN_POINT ( 'NONE',  ( -12.00000000000000888, -77.88958333333334849, 1.570796326794847264 ) ) ;
#23632=CARTESIAN_POINT ( 'NONE',  ( 3.521285801175999985, -79.12628491221198601, 10.69740673549999954 ) ) ;
#23634=CARTESIAN_POINT ( 'NONE',  ( 0.07899549168242259167, -79.67539556713441584, -11.83310309920475767 ) ) ;
#23643=CARTESIAN_POINT ( 'NONE',  ( 10.75000000000000000, -79.25000000000000000, 0.000000000000000000 ) ) ;
#23646=ORIENTED_EDGE ( 'NONE', *, *, #26394, .F. ) ;
#23649=CARTESIAN_POINT ( 'NONE',  ( 6.826798571050595399, -78.77984587750025014, -8.303980297556394774 ) ) ;
#23652=CARTESIAN_POINT ( 'NONE',  ( -7.695020077041000661, -76.18538407120952627, 8.115451295621999961 ) ) ;
#23657=CARTESIAN_POINT ( 'NONE',  ( 11.79859628133356786, -77.28603821643537231, -2.076809670760434656 ) ) ;
#23658=CARTESIAN_POINT ( 'NONE',  ( 8.733858618705999888, -78.46212780691099908, -7.038306768505999678 ) ) ;
#23662=VERTEX_POINT ( 'NONE', #11089 ) ;
#23667=CARTESIAN_POINT ( 'NONE',  ( -10.48543666025109289, -77.44166666666666288, -6.043427764450796325 ) ) ;
#23669=FACE_OUTER_BOUND ( 'NONE', #44901, .T. ) ;
#23678=CARTESIAN_POINT ( 'NONE',  ( -9.831591192207000063, -78.92583355886799268, -7.611166649991000455 ) ) ;
#23681=CARTESIAN_POINT ( 'NONE',  ( -0.5817747831294644012, -77.97935686554528445, 10.73539099268632846 ) ) ;
#23682=CARTESIAN_POINT ( 'NONE',  ( -11.61454496413000115, -77.61419278293099921, 2.935712811417999557 ) ) ;
#23687=CARTESIAN_POINT ( 'NONE',  ( 10.44832407724852530, -80.86929795574350521, 2.527760674094279736 ) ) ;
#23690=CARTESIAN_POINT ( 'NONE',  ( 9.509459933319000413, -77.25116639950799424, 5.592128946851999238 ) ) ;
#23692=CARTESIAN_POINT ( 'NONE',  ( 7.397492105520000472, -80.20748139727048454, 8.141545085894000167 ) ) ;
#23697=CARTESIAN_POINT ( 'NONE',  ( 4.275724345439000373, -76.85443832237800166, -10.36997068233999997 ) ) ;
#23699=CARTESIAN_POINT ( 'NONE',  ( 6.486265764543627022, -80.27377157478035485, 8.676841151407936437 ) ) ;
#23704=DIRECTION ( 'NONE',  ( 0.000000000000000000, -1.000000000000000000, 0.000000000000000000 ) ) ;
#23709=CARTESIAN_POINT ( 'NONE',  ( 0.5495723139228999576, -76.90547540590999631, -11.24864145460999865 ) ) ;
#23712=CARTESIAN_POINT ( 'NONE',  ( -12.00000000000000178, -79.31041666666665435, -1.570796326794897890 ) ) ;
#23718=VERTEX_POINT ( 'NONE', #17823 ) ;
#23720=CARTESIAN_POINT ( 'NONE',  ( -0.4077927620925000385, -79.58092127781698366, -11.02431129116999919 ) ) ;
#23735=CARTESIAN_POINT ( 'NONE',  ( 10.75000000000000000, -78.25000000000000000, 1.005550720961999908E-14 ) ) ;
#23739=CARTESIAN_POINT ( 'NONE',  ( 6.436424241555000592, -79.92391735373439587, 8.610165096135999008 ) ) ;
#23745=CARTESIAN_POINT ( 'NONE',  ( 0.3704480450335023156, -77.42746413819746465, -12.03686759590604005 ) ) ;
#23751=CARTESIAN_POINT ( 'NONE',  ( -11.03620408507000050, -80.21439667292020204, -2.260839449595000161 ) ) ;
#23752=CARTESIAN_POINT ( 'NONE',  ( -9.596002108778193929, -76.74791666666664014, 7.374560639698935383 ) ) ;
#23753=CARTESIAN_POINT ( 'NONE',  ( -2.813846212576811556, -76.70429982244345979, -10.47057735762498609 ) ) ;
#23768=CARTESIAN_POINT ( 'NONE',  ( -0.05316490922953205633, -79.47551739595091647, 10.74981279920144672 ) ) ;
#23786=ORIENTED_EDGE ( 'NONE', *, *, #31817, .T. ) ;
#23787=CARTESIAN_POINT ( 'NONE',  ( -11.15966350340000091, -79.60344789483799843, 4.490997254915999548 ) ) ;
#23798=EDGE_LOOP ( 'NONE', ( #3579, #22919, #7720, #29516, #1282, #44194, #6564, #14926 ) ) ;
#23801=ORIENTED_EDGE ( 'NONE', *, *, #26512, .F. ) ;
#23804=AXIS2_PLACEMENT_3D ( 'NONE', #33614, #33896, #46941 ) ;
#23805=CARTESIAN_POINT ( 'NONE',  ( -6.943703696083231236, -79.79999999999999716, -9.645494662058867519 ) ) ;
#23809=CARTESIAN_POINT ( 'NONE',  ( 8.154961773732001262, -76.07608039208299999, 7.653135223926000208 ) ) ;
#23833=CARTESIAN_POINT ( 'NONE',  ( -10.21414511300999983, -77.32657859425000879, 6.816672119949999775 ) ) ;
#23840=CARTESIAN_POINT ( 'NONE',  ( 1.841799093115999986, -80.57082220907369674, 11.13776847689000071 ) ) ;
#23844=CARTESIAN_POINT ( 'NONE',  ( -2.185791986076000004, -78.01107598727000436, -11.00183730042999919 ) ) ;
#23848=CYLINDRICAL_SURFACE ( 'NONE', #38727, 10.75000000000000000 ) ;
#23849=CARTESIAN_POINT ( 'NONE',  ( 5.533470947122165917, -81.00000000000000000, -9.578222253839143718 ) ) ;
#23852=CARTESIAN_POINT ( 'NONE',  ( 10.78853149093999875, -80.42508047494558809, -3.242959171380999983 ) ) ;
#23856=AXIS2_PLACEMENT_3D ( 'NONE', #57769, #39180, #7315 ) ;
#23859=CARTESIAN_POINT ( 'NONE',  ( -8.274737932560000786, -78.82433465545000217, -8.916907688993001457 ) ) ;
#23868=B_SPLINE_CURVE_WITH_KNOTS ( 'NONE', 3,
 ( #48101, #43363, #2922, #38350, #42795, #47817, #20639, #43087, #16214, #25634 ),
 .UNSPECIFIED., .F., .F.,
 ( 4, 2, 2, 2, 4 ),
 ( 0.000000000000000000, 0.2500000000000000000, 0.5000000000000000000, 0.7500000000000000000, 1.000000000000000000 ),
 .UNSPECIFIED. ) ;
#23884=ORIENTED_EDGE ( 'NONE', *, *, #48808, .F. ) ;
#23889=CARTESIAN_POINT ( 'NONE',  ( -8.987350104473000201, -77.00643677264099551, 8.369597699504998545 ) ) ;
#23897=EDGE_CURVE ( 'NONE', #1042, #45906, #23134, .T. ) ;
#23899=DIRECTION ( 'NONE',  ( -1.000000000000000000, 0.000000000000000000, 0.000000000000000000 ) ) ;
#23903=CARTESIAN_POINT ( 'NONE',  ( 7.889971116623999414, -77.39411321036999425, 8.954543982858998774 ) ) ;
#23907=CARTESIAN_POINT ( 'NONE',  ( 8.500174178665998781, -78.72261268016799818, -6.849988769802000554 ) ) ;
#23909=ORIENTED_EDGE ( 'NONE', *, *, #37415, .T. ) ;
#23913=CARTESIAN_POINT ( 'NONE',  ( 5.413904038987143785, -77.33333333333332860, 9.393203674808290771 ) ) ;
#23921=CARTESIAN_POINT ( 'NONE',  ( 0.9616906432771999969, -78.90839416819699181, -11.22092312000000014 ) ) ;
#23926=CARTESIAN_POINT ( 'NONE',  ( 5.745827208979935818, -78.68211204270377834, 9.633643064159604918 ) ) ;
#23933=AXIS2_PLACEMENT_3D ( 'NONE', #17752, #9479, #22464 ) ;
#23934=CARTESIAN_POINT ( 'NONE',  ( 3.140974612311327796, -77.15416666666668277, 11.68767212001979594 ) ) ;
#23938=CARTESIAN_POINT ( 'NONE',  ( 6.833867832890341276, -78.77991242188969068, -8.298164777206682885 ) ) ;
#23946=CARTESIAN_POINT ( 'NONE',  ( -0.7928288024956133828, -78.66963330304734825, -11.95371966526608176 ) ) ;
#23947=CARTESIAN_POINT ( 'NONE',  ( 5.986115112277999195, -80.16409694029599109, 9.486000076385000312 ) ) ;
#23949=DIRECTION ( 'NONE',  ( 1.000000000000000000, 0.000000000000000000, 0.000000000000000000 ) ) ;
#23955=DIRECTION ( 'NONE',  ( 0.000000000000000000, -1.000000000000000000, 0.000000000000000000 ) ) ;
#23966=CARTESIAN_POINT ( 'NONE',  ( -1.570796326794884790, -79.51458333333332007, -12.00000000000000355 ) ) ;
#23968=CARTESIAN_POINT ( 'NONE',  ( 10.36866725643501752, -77.87135762240245640, 2.843763427746201611 ) ) ;
#23970=CARTESIAN_POINT ( 'NONE',  ( 4.899854808515000215, -78.22463711524899566, -10.93194800986000104 ) ) ;
#23973=CARTESIAN_POINT ( 'NONE',  ( 6.606447392468458801, -78.92306693067979495, 8.596639545930225168 ) ) ;
#23975=CARTESIAN_POINT ( 'NONE',  ( 10.34875727357672304, -80.87214758697167838, 2.910059915723667512 ) ) ;
#23977=CARTESIAN_POINT ( 'NONE',  ( 10.61613183210000066, -77.68694788753698788, -2.999913216257000137 ) ) ;
#23979=CARTESIAN_POINT ( 'NONE',  ( -5.138300599984000350, -81.11256919153379386, -9.625040225332000432 ) ) ;
#23983=AXIS2_PLACEMENT_3D ( 'NONE', #17108, #18293, #35094 ) ;
#23985=CARTESIAN_POINT ( 'NONE',  ( -5.413111254871178168, -80.51674528042237000, 9.391950811569177660 ) ) ;
#23987=CARTESIAN_POINT ( 'NONE',  ( 5.151324428776999476, -77.60313545069999464, 9.964033682248000900 ) ) ;
#23997=CARTESIAN_POINT ( 'NONE',  ( -9.563148796606999014, -77.23231152193199023, 5.948121522994000543 ) ) ;
#24003=ORIENTED_EDGE ( 'NONE', *, *, #23897, .F. ) ;
#24011=CARTESIAN_POINT ( 'NONE',  ( 3.572416533754999790, -80.30722375786560008, 10.28603406935999942 ) ) ;
#24045=CARTESIAN_POINT ( 'NONE',  ( -6.606276669070258123, -76.67304179486919224, -8.596475147758464885 ) ) ;
#24065=DIRECTION ( 'NONE',  ( 0.000000000000000000, -1.000000000000000000, 0.000000000000000000 ) ) ;
#24076=CARTESIAN_POINT ( 'NONE',  ( -6.938593657451757046, -77.16921983703690557, -8.210840360290770690 ) ) ;
#24078=EDGE_CURVE ( 'NONE', #2543, #36429, #24190, .T. ) ;
#24080=CARTESIAN_POINT ( 'NONE',  ( 6.536979956083999177, -79.37240013963898377, -10.09826910480999906 ) ) ;
#24084=CARTESIAN_POINT ( 'NONE',  ( -3.073538647258000189, -78.22768216442000266, -11.53207971834999945 ) ) ;
#24090=B_SPLINE_CURVE_WITH_KNOTS ( 'NONE', 3,
 ( #38370, #15942, #6795, #24802, #46686, #52250, #29504, #20660, #20376, #29214, #56392, #51688, #7368, #24510, #37495, #42237, #25368, #2943, #55516, #15063, #10658, #51106, #2095, #28636, #33931, #51969, #6206, #24220, #1802, #42526, #56105, #19799, #55813, #11526, #15366 ),
 .UNSPECIFIED., .F., .F.,
 ( 4, 1, 1, 1, 1, 1, 1, 1, 1, 1, 1, 1, 1, 1, 1, 1, 1, 1, 1, 1, 1, 1, 1, 1, 1, 1, 1, 1, 1, 1, 1, 1, 4 ),
 ( 0.000000000000000000, 0.01250039628656018226, 0.04500037037602738765, 0.07750034446551849754, 0.1100003185549878609, 0.1425002926444572382, 0.1750002667339483342, 0.2075002408234176976, 0.2400002149128653839, 0.2725001890023130424, 0.3050001630917607010, 0.3375001371814254636, 0.3700001112708732331, 0.4025000853603208917, 0.4350000594497685502, 0.4675000335392162087, 0.5000000076286638118, 0.5324999817181115258, 0.5649999558075591288, 0.5974999298972240025, 0.6299999039866716055, 0.6624998780761193196, 0.6949998521655670336, 0.7274998262550146366, 0.7599998003444622396, 0.7924997744339099537, 0.8249997485235747163, 0.8574997226130225414, 0.8899996967024700334, 0.9224996707919177474, 0.9549996448813654615, 0.9874996189708130645, 1.000000000000000000 ),
 .UNSPECIFIED. ) ;
#24092=CARTESIAN_POINT ( 'NONE',  ( 12.00000000000000000, -78.04999999999999716, 0.000000000000000000 ) ) ;
#24093=AXIS2_PLACEMENT_3D ( 'NONE', #53975, #39215, #30343 ) ;
#24100=CARTESIAN_POINT ( 'NONE',  ( -1.670138242175404297, -79.80000000000002558, -11.69453362392147433 ) ) ;
#24103=CARTESIAN_POINT ( 'NONE',  ( 3.066118473086494767, -78.59774452897278252, -10.39032512872745251 ) ) ;
#24104=CARTESIAN_POINT ( 'NONE',  ( 11.06808393496999976, -76.45976679461099934, 1.603559079323000125 ) ) ;
#24106=CARTESIAN_POINT ( 'NONE',  ( 2.217579703669401603, -76.45950790555878029, 10.54848845899178578 ) ) ;
#24117=CARTESIAN_POINT ( 'NONE',  ( -9.993906532420947286, -78.07006040395985735, 3.960656951342677257 ) ) ;
#24121=CARTESIAN_POINT ( 'NONE',  ( 3.140974612311326908, -79.25416666666664867, 11.68767212001979772 ) ) ;
#24133=ORIENTED_EDGE ( 'NONE', *, *, #2639, .T. ) ;
#24136=CARTESIAN_POINT ( 'NONE',  ( 3.275195660744999682, -81.06043981312450342, 10.80351508457999898 ) ) ;
#24144=CARTESIAN_POINT ( 'NONE',  ( 10.51823340019644526, -81.00000000000001421, -3.220802781544626292 ) ) ;
#24149=FACE_OUTER_BOUND ( 'NONE', #28944, .T. ) ;
#24157=ORIENTED_EDGE ( 'NONE', *, *, #19611, .T. ) ;
#24158=CARTESIAN_POINT ( 'NONE',  ( -10.42801618316999956, -78.71581739375498898, 6.264104809848999977 ) ) ;
#24165=CARTESIAN_POINT ( 'NONE',  ( -12.00000000000000355, -79.78958333333331154, 1.570796326794848596 ) ) ;
#24171=ORIENTED_EDGE ( 'NONE', *, *, #39337, .F. ) ;
#24181=DIRECTION ( 'NONE',  ( -1.000000000000000000, 0.000000000000000000, 0.000000000000000000 ) ) ;
#24187=CARTESIAN_POINT ( 'NONE',  ( 3.090997446795999970, -77.21135046416598868, -11.88544462247999967 ) ) ;
#24188=AXIS2_PLACEMENT_3D ( 'NONE', #8730, #31733, #4897 ) ;
#24190=CIRCLE ( 'NONE', #44924, 9.700000000000001066 ) ;
#24193=CARTESIAN_POINT ( 'NONE',  ( -4.019809786096000259, -79.15416738576453781, 10.47183077952999852 ) ) ;
#24195=VERTEX_POINT ( 'NONE', #10063 ) ;
#24202=CARTESIAN_POINT ( 'NONE',  ( -11.80948866808000020, -78.49294670917899452, 2.394107155543000243 ) ) ;
#24220=CARTESIAN_POINT ( 'NONE',  ( 5.380879925577582767, -76.18494410599546995, 9.804299052675480297 ) ) ;
#24221=DIRECTION ( 'NONE',  ( 3.552713678800000476E-14, 1.000000000000000000, -1.480997164338000095E-13 ) ) ;
#24236=AXIS2_PLACEMENT_3D ( 'NONE', #35374, #53399, #26820 ) ;
#24239=CARTESIAN_POINT ( 'NONE',  ( 6.955482170287579535, -78.78106476872730468, -8.196585751274280796 ) ) ;
#24242=VERTEX_POINT ( 'NONE', #646 ) ;
#24248=CARTESIAN_POINT ( 'NONE',  ( -11.92783303768075776, -77.55733137067235816, -1.116597677413008194 ) ) ;
#24249=CARTESIAN_POINT ( 'NONE',  ( -7.408849624938999234, -79.40147933624500354, -8.421820339245000397 ) ) ;
#24251=EDGE_LOOP ( 'NONE', ( #36779, #341, #50913, #51665 ) ) ;
#24255=CARTESIAN_POINT ( 'NONE',  ( -3.513492303797125071, -78.44955557553232950, -10.65255456408984180 ) ) ;
#24259=CARTESIAN_POINT ( 'NONE',  ( 10.48543666025110355, -78.60833333333330586, -6.043427764450775008 ) ) ;
#24267=CARTESIAN_POINT ( 'NONE',  ( 9.596002108778174389, -79.59791666666666288, -7.374560639698961140 ) ) ;
#24268=CARTESIAN_POINT ( 'NONE',  ( -5.918356417140000048, -76.19414720733000479, 9.991160380212999570 ) ) ;
#24269=CARTESIAN_POINT ( 'NONE',  ( 10.74991461791089264, -77.85495667263820962, 0.6503649595168488062 ) ) ;
#24270=CARTESIAN_POINT ( 'NONE',  ( -10.61596739836999959, -78.60444753118198946, -5.551333230057999835 ) ) ;
#24273=CARTESIAN_POINT ( 'NONE',  ( 9.662273249694312227, -78.88660371430214013, 4.763867255732987971 ) ) ;
#24278=CARTESIAN_POINT ( 'NONE',  ( 8.145694891731999121, -78.14996571856799790, -7.439717004853000581 ) ) ;
#24280=CARTESIAN_POINT ( 'NONE',  ( -10.89192327684000006, -80.52192009945389373, 0.6399950417793000002 ) ) ;
#24285=CARTESIAN_POINT ( 'NONE',  ( -10.74953850517756848, -80.58960968215087917, 1.406898149230603412 ) ) ;
#24286=CARTESIAN_POINT ( 'NONE',  ( -10.96060824219999930, -77.24906299167599855, 2.383941600041999731 ) ) ;
#24300=CARTESIAN_POINT ( 'NONE',  ( -8.763613300111000370, -76.72389978589799853, 6.838397221053000408 ) ) ;
#24303=CARTESIAN_POINT ( 'NONE',  ( -9.596002108778193929, -77.74791666666664014, 7.374560639698935383 ) ) ;
#24312=CARTESIAN_POINT ( 'NONE',  ( -6.285096537930999538, -78.96846735336799838, -9.206093747065001054 ) ) ;
#24313=CARTESIAN_POINT ( 'NONE',  ( 10.75000000000000000, -80.25000000000000000, -1.651583051307000043E-14 ) ) ;
#24326=CARTESIAN_POINT ( 'NONE',  ( 8.822637088635000069, -80.00128349074179823, 6.926713255916000733 ) ) ;
#24331=CARTESIAN_POINT ( 'NONE',  ( 0.000000000000000000, -75.15999999999999659, 0.000000000000000000 ) ) ;
#24347=CARTESIAN_POINT ( 'NONE',  ( -6.043427764450833628, -77.31666666666666288, 10.48543666025107335 ) ) ;
#24354=CARTESIAN_POINT ( 'NONE',  ( -7.835303970625000503, -78.25963867675800145, 8.089621514298000804 ) ) ;
#24363=CARTESIAN_POINT ( 'NONE',  ( -0.2916556773643344536, -79.47731085430962139, 10.74608969385784185 ) ) ;
#24377=CARTESIAN_POINT ( 'NONE',  ( -7.514905133372472790, -77.16340258555835874, -7.687053346723279112 ) ) ;
#24382=CARTESIAN_POINT ( 'NONE',  ( -11.95950202284999975, -79.12530980127799296, 1.295167635372999948 ) ) ;
#24385=VERTEX_POINT ( 'NONE', #38992 ) ;
#24386=CARTESIAN_POINT ( 'NONE',  ( 7.822091542723999424, -77.30528544001199975, -9.013910121987001034 ) ) ;
#24389=CARTESIAN_POINT ( 'NONE',  ( -2.813789756862300262, -78.89583333333334281, 10.47020627418438465 ) ) ;
#24398=CARTESIAN_POINT ( 'NONE',  ( -8.596418555780431348, -80.55208333333331439, -6.606377239730338857 ) ) ;
#24400=CARTESIAN_POINT ( 'NONE',  ( -7.384493003614710283, -79.80000000000001137, -9.307078043242871246 ) ) ;
#24405=CARTESIAN_POINT ( 'NONE',  ( 1.546553306619000256, -76.40214563794199876, -11.07619323537999989 ) ) ;
#24406=CARTESIAN_POINT ( 'NONE',  ( 10.82209551222215715, -76.35773650856198458, 0.9128778866761866340 ) ) ;
#24408=CARTESIAN_POINT ( 'NONE',  ( 5.198613046211999489, -76.66010485387299411, 9.952796194076000802 ) ) ;
#24415=CARTESIAN_POINT ( 'NONE',  ( 11.96908924566999843, -79.33756653719200358, 1.661418422374000059 ) ) ;
#24416=CARTESIAN_POINT ( 'NONE',  ( -8.939668861401381506, -78.05329775042086737, 5.970159216130292101 ) ) ;
#24417=VECTOR ( 'NONE', #29041, 1000.000000000000114 ) ;
#24426=CARTESIAN_POINT ( 'NONE',  ( 0.000000000000000000, -87.25000000009099210, 0.000000000000000000 ) ) ;
#24433=EDGE_CURVE ( 'NONE', #46988, #46084, #3559, .T. ) ;
#24435=CARTESIAN_POINT ( 'NONE',  ( -11.15592782356999990, -80.22109534903739814, -1.728406004469000168 ) ) ;
#24436=PRODUCT_DEFINITION_FORMATION_WITH_SPECIFIED_SOURCE ( 'ANY', '', #30452, .NOT_KNOWN. ) ;
#24439=CARTESIAN_POINT ( 'NONE',  ( 11.19180402071999936, -77.65700352824698882, 0.7494220128532999015 ) ) ;
#24454=CARTESIAN_POINT ( 'NONE',  ( 10.33787006668000075, -78.55304150121298790, 6.411783922571999916 ) ) ;
#24462=CARTESIAN_POINT ( 'NONE',  ( 8.596684946446202957, -77.79795771992381503, -6.606655141920929175 ) ) ;
#24466=CARTESIAN_POINT ( 'NONE',  ( 10.21235917355000034, -79.79466669503099752, -3.857859667932999947 ) ) ;
#24480=CARTESIAN_POINT ( 'NONE',  ( 8.174587033571999228, -77.25233320247099300, -8.440297792765999674 ) ) ;
#24484=CARTESIAN_POINT ( 'NONE',  ( 10.58946819037999987, -78.47325881071910203, -3.698823201301000285 ) ) ;
#24492=AXIS2_PLACEMENT_3D ( 'NONE', #17176, #87, #40193 ) ;
#24493=CARTESIAN_POINT ( 'NONE',  ( 1.659836960048000076, -78.80503006069899641, 11.81542141165000004 ) ) ;
#24497=CARTESIAN_POINT ( 'NONE',  ( -10.46946769381999864, -79.04944879618999209, -3.092832390908999862 ) ) ;
#24500=ADVANCED_FACE ( 'NONE', ( #12699 ), #4138, .F. ) ;
#24508=ORIENTED_EDGE ( 'NONE', *, *, #2518, .F. ) ;
#24509=CARTESIAN_POINT ( 'NONE',  ( 10.94267788024999888, -79.50759371423698951, -2.663036869319000299 ) ) ;
#24510=CARTESIAN_POINT ( 'NONE',  ( 7.778309126724593625, -76.53609129384345522, -8.035922781116632052 ) ) ;
#24511=CARTESIAN_POINT ( 'NONE',  ( 0.4924606920183405290, -79.42146225091693168, 11.76080498934809704 ) ) ;
#24522=CARTESIAN_POINT ( 'NONE',  ( 9.913660282387342093, -76.25821898709155278, 4.411731727441804196 ) ) ;
#24523=CARTESIAN_POINT ( 'NONE',  ( 1.407199643270103717, -78.46460707205700658, 10.68074055511154086 ) ) ;
#24528=CARTESIAN_POINT ( 'NONE',  ( 1.277940389835883872, -78.73453218978592361, -10.67965253657788516 ) ) ;
#24539=CARTESIAN_POINT ( 'NONE',  ( 3.632329907060999563, -80.25004305557349937, 10.45854222826000068 ) ) ;
#24545=CARTESIAN_POINT ( 'NONE',  ( -10.96076062099048976, -77.33286551245832641, 2.383974742557829707 ) ) ;
#24558=CARTESIAN_POINT ( 'NONE',  ( 7.685088506145000942, -78.69410935321799627, 9.438228493448001188 ) ) ;
#24561=CARTESIAN_POINT ( 'NONE',  ( 7.851705946354000432, -77.31577031326999361, -9.048036745432998629 ) ) ;
#24562=FACE_OUTER_BOUND ( 'NONE', #43612, .T. ) ;
#24568=CARTESIAN_POINT ( 'NONE',  ( 6.963658808075999573, -78.70794695701400201, -8.131364605499999954 ) ) ;
#24570=CARTESIAN_POINT ( 'NONE',  ( 5.346968534282000363, -80.36083398343220097, 9.510689753416999181 ) ) ;
#24578=EDGE_CURVE ( 'NONE', #9748, #2879, #3845, .T. ) ;
#24579=CARTESIAN_POINT ( 'NONE',  ( 8.282307197233999219, -77.95720790972299596, -7.564489280985000619 ) ) ;
#24583=CARTESIAN_POINT ( 'NONE',  ( -6.446612550560000265, -76.65709426284900019, -10.30178301210999869 ) ) ;
#24616=CARTESIAN_POINT ( 'NONE',  ( 4.782478426736999744, -79.53826565971098717, 10.14623135401999932 ) ) ;
#24634=CARTESIAN_POINT ( 'NONE',  ( 9.393545413109377407, -76.80849324769383202, -5.414107032282895915 ) ) ;
#24637=DIRECTION ( 'NONE',  ( 1.000000000000000000, 0.000000000000000000, 0.000000000000000000 ) ) ;
#24638=CARTESIAN_POINT ( 'NONE',  ( -12.00000000000000888, -78.38958333333333428, 1.570796326794847264 ) ) ;
#24640=CARTESIAN_POINT ( 'NONE',  ( 0.2665495375979000103, -78.45029307777100769, -11.25891151133000001 ) ) ;
#24644=DIRECTION ( 'NONE',  ( 1.000000000000000000, 0.000000000000000000, 0.000000000000000000 ) ) ;
#24651=CARTESIAN_POINT ( 'NONE',  ( -0.5544288313492085063, -79.47928052470416560, 10.73600753435132482 ) ) ;
#24652=B_SPLINE_CURVE_WITH_KNOTS ( 'NONE', 3,
 ( #40672, #27947, #263, #18245, #36234, #54257, #31791, #49833, #37982, #46583, #28535, #24989, #7275, #56294, #15262, #15557, #6985, #25277 ),
 .UNSPECIFIED., .F., .F.,
 ( 4, 2, 2, 2, 2, 2, 2, 2, 4 ),
 ( 0.000000000000000000, 0.1250000000000000555, 0.2500000000000001110, 0.3750000000000001665, 0.5000000000000002220, 0.6250000000000002220, 0.7500000000000002220, 0.8750000000000001110, 1.000000000000000000 ),
 .UNSPECIFIED. ) ;
#24667=CARTESIAN_POINT ( 'NONE',  ( 4.168617279563824773, -80.25678616003493460, -9.908796504410707584 ) ) ;
#24670=AXIS2_PLACEMENT_3D ( 'NONE', #55106, #1396, #19391 ) ;
#24671=CARTESIAN_POINT ( 'NONE',  ( -10.65106809510000119, -79.09542617043000234, 5.591232889670999739 ) ) ;
#24675=CARTESIAN_POINT ( 'NONE',  ( -10.23070583620000207, -78.58036326492899093, 6.145580569783000158 ) ) ;
#24686=CARTESIAN_POINT ( 'NONE',  ( -10.07979664880000037, -76.97175206120299151, 3.736335038366999761 ) ) ;
#24690=CARTESIAN_POINT ( 'NONE',  ( 10.62400023845289532, -79.79999999999999716, 5.163243916854518112 ) ) ;
#24694=CARTESIAN_POINT ( 'NONE',  ( -10.99972769911000015, -76.31944253928298849, 2.019869862886000345 ) ) ;
#24698=CARTESIAN_POINT ( 'NONE',  ( -7.942520732695999008, -76.51965762081900380, -7.609088033453000222 ) ) ;
#24705=CARTESIAN_POINT ( 'NONE',  ( -11.78732249294000134, -79.09425612125899363, -2.660533726555999845 ) ) ;
#24707=CARTESIAN_POINT ( 'NONE',  ( -8.337895600304513266, -78.04578102920540061, 6.785427785908417775 ) ) ;
#24728=CARTESIAN_POINT ( 'NONE',  ( -10.05535668103000191, -78.36514844629400045, 4.970705447719999448 ) ) ;
#24741=ORIENTED_EDGE ( 'NONE', *, *, #28233, .T. ) ;
#24742=CARTESIAN_POINT ( 'NONE',  ( 9.289757862025998847, -78.06471382358499511, 7.853848066408001038 ) ) ;
#24747=EDGE_CURVE ( 'NONE', #51603, #28435, #15035, .T. ) ;
#24751=CARTESIAN_POINT ( 'NONE',  ( 10.48543666025108401, -79.59166666666666856, 6.043427764450814976 ) ) ;
#24754=CARTESIAN_POINT ( 'NONE',  ( -8.065049863481000614, -78.51455857394600457, 7.357332172019000360 ) ) ;
#24756=CARTESIAN_POINT ( 'NONE',  ( 3.463448050014508173, -80.75108394742497353, -10.20029982960495651 ) ) ;
#24772=CARTESIAN_POINT ( 'NONE',  ( -12.17466003208999936, -76.55562665128699962, 1.612538369963999907 ) ) ;
#24775=CARTESIAN_POINT ( 'NONE',  ( -10.48543666025109111, -77.84166666666665435, -6.043427764450793660 ) ) ;
#24783=CARTESIAN_POINT ( 'NONE',  ( 10.85897810694999954, -78.15392649052799356, -5.483167429328999809 ) ) ;
#24791=AXIS2_PLACEMENT_3D ( 'NONE', #15038, #51944, #3212 ) ;
#24794=CARTESIAN_POINT ( 'NONE',  ( 2.269106295766999856E-14, -92.79999999999999716, -12.09999999998845865 ) ) ;
#24797=CARTESIAN_POINT ( 'NONE',  ( -1.570796326794884790, -78.01458333333333428, -12.00000000000000355 ) ) ;
#24800=CARTESIAN_POINT ( 'NONE',  ( -4.169330562119000660, -79.37141199922800183, -10.46186633551000078 ) ) ;
#24802=CARTESIAN_POINT ( 'NONE',  ( -7.860640992941333671, -76.78691071373445709, 7.955411750889882505 ) ) ;
#24817=CARTESIAN_POINT ( 'NONE',  ( 12.26182288558000089, -76.99428088996099007, -2.272484397021000024 ) ) ;
#24818=CARTESIAN_POINT ( 'NONE',  ( 5.974621249351785401, -78.77206790660797253, -8.936673600286241026 ) ) ;
#24824=CARTESIAN_POINT ( 'NONE',  ( 1.407207864692765265, -79.73543568848991470, -10.68080165316230001 ) ) ;
#24826=EDGE_CURVE ( 'NONE', #23344, #21820, #28307, .T. ) ;
#24828=CARTESIAN_POINT ( 'NONE',  ( 10.89876807034000095, -79.56489739425599339, -2.652350870517000025 ) ) ;
#24829=ORIENTED_EDGE ( 'NONE', *, *, #44536, .T. ) ;
#24835=CARTESIAN_POINT ( 'NONE',  ( -0.9512462306705773418, -78.23166483151833006, 11.17661574778309408 ) ) ;
#24844=CARTESIAN_POINT ( 'NONE',  ( 7.652056849481999379, -79.47013533719341183, 9.281873293285000770 ) ) ;
#24851=CARTESIAN_POINT ( 'NONE',  ( 6.606356555483213100, -79.27722184295002705, -8.596560213042563348 ) ) ;
#24852=CARTESIAN_POINT ( 'NONE',  ( 4.899854808515000215, -78.15684856197299268, -10.93194800986000104 ) ) ;
#24856=CARTESIAN_POINT ( 'NONE',  ( 10.24002203034363490, -80.87489730094399931, 3.274717220204576229 ) ) ;
#24859=CARTESIAN_POINT ( 'NONE',  ( 6.327673118679000730, -77.63247520153299774, -9.036718833993001354 ) ) ;
#24861=CARTESIAN_POINT ( 'NONE',  ( -8.965068030445999980, -80.97833076151569287, 6.218612530207000333 ) ) ;
#24866=CARTESIAN_POINT ( 'NONE',  ( -2.813754150119270658, -80.49592687992846152, 10.47067054086312332 ) ) ;
#24867=CARTESIAN_POINT ( 'NONE',  ( 7.199825537761999961, -77.08564493366499448, 8.601198917431998936 ) ) ;
#24881=DIRECTION ( 'NONE',  ( 0.000000000000000000, -1.000000000000000000, 0.000000000000000000 ) ) ;
#24892=EDGE_LOOP ( 'NONE', ( #39123, #22935, #14335, #7831 ) ) ;
#24896=CARTESIAN_POINT ( 'NONE',  ( 0.4065037703597895180, -80.99999999999997158, -10.96443877910777864 ) ) ;
#24897=CARTESIAN_POINT ( 'NONE',  ( -10.82730428396000022, -77.08360301469699039, -1.394578048285000094 ) ) ;
#24908=CARTESIAN_POINT ( 'NONE',  ( -12.00000000000000000, -76.89999999999999147, 0.000000000000000000 ) ) ;
#24914=CARTESIAN_POINT ( 'NONE',  ( 1.570796326794856590, -76.76458333333333428, 12.00000000000000711 ) ) ;
#24921=CARTESIAN_POINT ( 'NONE',  ( -11.68767212001980127, -77.37916666666666288, 3.140974612311317138 ) ) ;
#24926=CARTESIAN_POINT ( 'NONE',  ( 4.029831046159999985, -78.47752942077299565, -10.51637221458999960 ) ) ;
#24931=DIRECTION ( 'NONE',  ( 0.000000000000000000, -1.000000000000000000, 0.000000000000000000 ) ) ;
#24938=CYLINDRICAL_SURFACE ( 'NONE', #35762, 10.75000000000000000 ) ;
#24940=DIRECTION ( 'NONE',  ( 1.000000000000000000, 0.000000000000000000, 0.000000000000000000 ) ) ;
#24943=CARTESIAN_POINT ( 'NONE',  ( 6.327673118679000730, -77.31474813712100058, -9.036718833993001354 ) ) ;
#24953=CARTESIAN_POINT ( 'NONE',  ( 0.4713521909880000194, -78.93798672461099386, 12.02020425643999957 ) ) ;
#24973=CARTESIAN_POINT ( 'NONE',  ( -0.4686848344790195964, -79.80000000000002558, -11.78742881352508753 ) ) ;
#24974=CARTESIAN_POINT ( 'NONE',  ( -8.864498852882359614, -80.05242134712879931, 6.083669688407788101 ) ) ;
#24976=CARTESIAN_POINT ( 'NONE',  ( -8.075725583014000009, -76.39468836525099960, -7.736700848913999451 ) ) ;
#24980=CARTESIAN_POINT ( 'NONE',  ( -1.423492296534000001, -76.27635696248199793, 11.02239954532999988 ) ) ;
#24988=CARTESIAN_POINT ( 'NONE',  ( 10.24033359635999929, -79.30459810362600592, 6.632096080123999648 ) ) ;
#24989=CARTESIAN_POINT ( 'NONE',  ( 9.686447855663514517, -76.23750000000886473, 7.039619684793525067 ) ) ;
#25003=CARTESIAN_POINT ( 'NONE',  ( -5.052420809101000088E-14, -80.84999999994218456, -13.94999999993999928 ) ) ;
#25006=CARTESIAN_POINT ( 'NONE',  ( -0.3187246912203000049, -80.62725096977128203, 11.26088853021000169 ) ) ;
#25013=CARTESIAN_POINT ( 'NONE',  ( 3.891476699446599241, -79.94576739355758832, 10.02177961226664671 ) ) ;
#25020=ADVANCED_FACE ( 'NONE', ( #10918, #33900 ), #6470, .F. ) ;
#25023=AXIS2_PLACEMENT_3D ( 'NONE', #51826, #21091, #24940 ) ;
#25026=CARTESIAN_POINT ( 'NONE',  ( 12.06733228363000165, -78.49878287036499103, -1.536887159723000051 ) ) ;
#25028=VECTOR ( 'NONE', #53512, 1000.000000000000000 ) ;
#25036=CARTESIAN_POINT ( 'NONE',  ( -6.155296265070999695, -78.65074028895499225, -9.015968826447998907 ) ) ;
#25044=CARTESIAN_POINT ( 'NONE',  ( -9.211739516216143286, -80.80159234348433017, 6.389716016208851990 ) ) ;
#25045=CARTESIAN_POINT ( 'NONE',  ( 8.941518625654639507, -78.95754834277080647, 7.898890069118407631 ) ) ;
#25054=CARTESIAN_POINT ( 'NONE',  ( -6.018890980713000438, -75.98186831501799077, 10.70471907396000155 ) ) ;
#25066=CARTESIAN_POINT ( 'NONE',  ( -8.274737932560000786, -78.50660759103701025, -8.916907688993001457 ) ) ;
#25072=CARTESIAN_POINT ( 'NONE',  ( -9.961878266999939058, -79.56943413225670270, 4.040113604248548818 ) ) ;
#25077=CARTESIAN_POINT ( 'NONE',  ( 6.290942473662262557, -79.73124999999996021, 10.26217848164658264 ) ) ;
#25094=B_SPLINE_SURFACE_WITH_KNOTS ( 'NONE', 3, 3, ( 
 ( #10020, #27998, #41595, #1175, #19164, #46338, #24466, #42478, #34963, #37744, #26397, #15605, #33599, #48574, #28877, #26116, #52993, #2616, #39695, #57702, #20612, #44418, #38614, #15895, #20048, #12542, #30540, #19749, #51638, #8116, #2047, #44137, #3685, #21687, #29169, #38036, #30824, #56342, #17257, #51921, #35247, #53278, #12824, #48858, #11192, #8400, #56058, #47215, #25036, #55767, #6744, #15313, #33307, #24754, #56629, #51342, #47509, #42770, #10901, #46923, #6451, #2331, #20326, #16979, #38322, #33881, #11479 ),
 ( #29451, #7036, #43057, #21972, #49450, #57997, #8998, #26982, #13409, #49146, #45016, #3970, #39983, #17553, #35545, #53573, #13111, #31105, #8696, #26687, #4272, #35846, #44718, #22268, #53875, #40284, #58295, #17857, #31407, #57605, #35151, #26015, #44041, #7449, #57898, #48761, #44322, #3591, #48475, #39601, #52900, #13013, #25734, #56756, #3024, #3878, #8598, #26584, #53472, #29863, #39315, #21022, #22171, #39027, #34584, #34296, #31012, #57039, #30726, #57324, #53184, #49050, #16598, #35441, #52615, #8019, #25448 ),
 ( #44618, #12732, #16888, #21877, #26307, #17455, #12166, #7734, #3312, #4174, #8307, #21596, #16315, #52330, #39885, #34869, #17165, #11885, #47917, #30152, #43469, #48203, #43761, #21306, #12449, #30444, #72, #9771, #45803, #49642, #22466, #50516, #18344, #5338, #13899, #41357, #939, #27760, #23345, #31599, #14187, #44911, #4468, #45505, #18921, #40479, #36916, #54926, #45210, #41066, #14480, #9482, #27173, #28050, #50224, #8893, #32470, #10069, #18637, #36629, #46095, #54648, #36042, #32184, #26887, #36334, #5621 ),
 ( #18051, #40179, #58192, #17755, #4759, #35742, #53773, #13309, #31303, #49346, #54067, #23050, #13603, #9188, #22761, #40770, #364, #54359, #31892, #49937, #27469, #5052, #652, #46972, #24509, #2094, #51391, #10947, #32763, #24800, #15650, #11236, #28928, #15364, #6499, #19798, #38369, #10656, #23632, #5912, #47261, #33930, #51968, #20375, #55218, #6205, #23921, #47557, #1510, #19499, #19214, #56391, #37494, #33647, #1801, #51687, #15941, #28635, #2378, #46685, #33358, #37792, #37207, #29502, #55812, #41645, #6794 ) ),
 .UNSPECIFIED., .F., .F., .F.,
 ( 4, 4 ),
 ( 4, 1, 1, 1, 1, 1, 1, 1, 1, 1, 1, 1, 1, 1, 1, 1, 1, 1, 1, 1, 1, 1, 1, 1, 1, 1, 1, 1, 1, 1, 1, 1, 1, 1, 1, 1, 1, 1, 1, 1, 1, 1, 1, 1, 1, 1, 1, 1, 1, 1, 1, 1, 1, 1, 1, 1, 1, 1, 1, 1, 1, 1, 1, 1, 4 ),
 ( -0.1772706441294000235, 1.177270644128999955 ),
 ( -0.02000000000000000042, -0.003749999999999999861, 0.01250000000000000069, 0.02875000000000000125, 0.04499999999999999833, 0.06124999999999999889, 0.07749999999999999944, 0.09375000000000000000, 0.1100000000000000006, 0.1262500000000000011, 0.1424999999999999878, 0.1587500000000000022, 0.1749999999999999889, 0.1912500000000000033, 0.2074999999999999900, 0.2237500000000000044, 0.2399999999999999911, 0.2562499999999999778, 0.2725000000000000200, 0.2887500000000000067, 0.3049999999999999933, 0.3212499999999999800, 0.3375000000000000222, 0.3537500000000000089, 0.3699999999999999956, 0.3862499999999999822, 0.4025000000000000244, 0.4187500000000000111, 0.4349999999999999978, 0.4512499999999999845, 0.4675000000000000266, 0.4837500000000000133, 0.5000000000000000000, 0.5162499999999999867, 0.5324999999999999734, 0.5487499999999999600, 0.5649999999999999467, 0.5812500000000000444, 0.5975000000000000311, 0.6137500000000000178, 0.6300000000000000044, 0.6462499999999999911, 0.6624999999999999778, 0.6787499999999999645, 0.6949999999999999512, 0.7112500000000000488, 0.7275000000000000355, 0.7437500000000000222, 0.7600000000000000089, 0.7762499999999999956, 0.7924999999999999822, 0.8087499999999999689, 0.8249999999999999556, 0.8412500000000000533, 0.8575000000000000400, 0.8737500000000000266, 0.8900000000000000133, 0.9062500000000000000, 0.9224999999999999867, 0.9387499999999999734, 0.9549999999999999600, 0.9712499999999999467, 0.9875000000000000444, 1.003749999999999920, 1.020000000000000018 ),
 .UNSPECIFIED. ) ;
#25099=CARTESIAN_POINT ( 'NONE',  ( -0.6772390005816000258, -76.37953981538699111, -12.45222204340999994 ) ) ;
#25100=CARTESIAN_POINT ( 'NONE',  ( -4.695314103947369588, -78.68919620935585613, -9.670285998753380241 ) ) ;
#25112=CARTESIAN_POINT ( 'NONE',  ( 11.21665020278000036, -78.58438904619100640, 0.06973997782872000395 ) ) ;
#25120=CARTESIAN_POINT ( 'NONE',  ( 8.196767141791585942, -77.65970162848033453, 7.657324427439206715 ) ) ;
#25122=CARTESIAN_POINT ( 'NONE',  ( 0.000000000000000000, -75.15999999999999659, 0.000000000000000000 ) ) ;
#25123=CARTESIAN_POINT ( 'NONE',  ( 10.74999999999999645, -80.76041666666665719, 1.407171709420451666 ) ) ;
#25127=CARTESIAN_POINT ( 'NONE',  ( -12.02912753549999891, -79.64943712227855599, 0.08506824670321999626 ) ) ;
#25134=CARTESIAN_POINT ( 'NONE',  ( 8.770451247185000909, -78.80795213214298656, 8.160602927202999624 ) ) ;
#25141=EDGE_CURVE ( 'NONE', #24195, #51047, #29866, .T. ) ;
#25142=CARTESIAN_POINT ( 'NONE',  ( 9.605397716210999803, -77.23718443491598862, -5.187648860687999353 ) ) ;
#25149=DIRECTION ( 'NONE',  ( 0.000000000000000000, -1.000000000000000000, 0.000000000000000000 ) ) ;
#25150=CARTESIAN_POINT ( 'NONE',  ( 10.79417609527999922, -77.49419007869299492, -3.050225076229999832 ) ) ;
#25154=CARTESIAN_POINT ( 'NONE',  ( 9.236131044632999831, -76.77029247776400211, -7.898064948592000256 ) ) ;
#25157=ORIENTED_EDGE ( 'NONE', *, *, #37091, .F. ) ;
#25174=ORIENTED_EDGE ( 'NONE', *, *, #53262, .F. ) ;
#25175=VERTEX_POINT ( 'NONE', #57793 ) ;
#25179=CARTESIAN_POINT ( 'NONE',  ( -5.773354541636604331, -81.00000000000004263, -9.267588486114398449 ) ) ;
#25180=CARTESIAN_POINT ( 'NONE',  ( 6.261651594248000663, -77.24702107270799445, -8.942431733175999042 ) ) ;
#25186=B_SPLINE_CURVE_WITH_KNOTS ( 'NONE', 3,
 ( #17028, #11743, #43038, #38595, #30007, #47770, #16745, #20877, #34726, #38880, #56900, #16457, #48061, #44469, #17608, #9049, #31458, #50090, #48910, #26740, #4020, #54219, #14051, #53327, #53624, #13462, #9634, #22025, #27622, #36200, #45073, #22624, #230, #13753, #27035, #4624, #8451, #516, #49798, #45367, #40636, #4321, #44771, #58346, #9345, #49500, #40033, #32046, #18209, #30875, #31754, #45663, #58048, #4916, #22322, #35298, #27333, #22915, #5205, #40929, #18493, #17909, #23206, #35596, #36485, #57754, #54514, #17311, #12873, #13162, #26446, #31159, #40337, #49197, #8750, #35898, #53930, #37064, #50380, #50674, #29083, #19652, #28493, #801, #1960, #10808, #1369, #46544, #47128, #28788, #45955, #46834, #6361, #24076, #11103, #19365, #55964, #5486, #9927, #18784, #24377, #42389, #19953, #32621, #15218, #23491, #41504, #6068, #37942, #1089, #15515 ),
 .UNSPECIFIED., .F., .F.,
 ( 4, 2, 2, 2, 2, 2, 2, 2, 1, 1, 2, 2, 2, 2, 2, 2, 2, 2, 1, 1, 2, 2, 2, 2, 2, 2, 2, 1, 1, 1, 2, 2, 2, 2, 2, 2, 2, 1, 2, 2, 1, 1, 2, 2, 2, 2, 2, 2, 1, 2, 2, 2, 2, 1, 1, 1, 2, 1, 1, 1, 2, 2, 2, 4 ),
 ( 0.000000000000000000, 0.06250000000000904832, 0.1250000000000180966, 0.1562500000000226208, 0.1875000000000271450, 0.2187500000000316691, 0.2343750000000339173, 0.2421875000000350830, 0.2460937500000356937, 0.2480468750000359990, 0.2490234375000361655, 0.2500000000000363043, 0.2812500000000405231, 0.3125000000000447975, 0.3750000000000532352, 0.4375000000000616729, 0.4687500000000658917, 0.4843750000000680567, 0.4921875000000691669, 0.4960937500000696665, 0.4980468750000699441, 0.5000000000000701661, 0.5312500000000739409, 0.5625000000000774936, 0.5703125000000784928, 0.5712890625000786038, 0.5715332031250786038, 0.5717773437500787148, 0.5722656250000787148, 0.5742187500000786038, 0.5781250000000783817, 0.5937500000000774936, 0.6015625000000770495, 0.6054687500000769385, 0.6093750000000767164, 0.6250000000000760503, 0.6406250000000753841, 0.6425781250000753841, 0.6428222656250752731, 0.6430664062500752731, 0.6435546875000751621, 0.6445312500000749401, 0.6484375000000746070, 0.6562500000000736078, 0.6875000000000695000, 0.6953125000000685008, 0.6962890625000683897, 0.6972656250000682787, 0.6992187500000681677, 0.7031250000000677236, 0.7187500000000659472, 0.7226562500000655032, 0.7236328125000653921, 0.7246093750000651701, 0.7265625000000648370, 0.7343750000000638378, 0.7421875000000626166, 0.7460937500000620615, 0.7480468750000617284, 0.7490234375000617284, 0.7495117187500616174, 0.7500000000000616174, 0.8750000000000308642, 1.000000000000000000 ),
 .UNSPECIFIED. ) ;
#25197=CARTESIAN_POINT ( 'NONE',  ( -10.47020627418439354, -76.52083333333334281, -2.813789756862263847 ) ) ;
#25232=CARTESIAN_POINT ( 'NONE',  ( 2.837175473061999575, -78.06338377657900196, 10.77984396480000129 ) ) ;
#25237=CARTESIAN_POINT ( 'NONE',  ( 9.599999999916001059, -87.30000000008399752, -6.531555804621000072E-10 ) ) ;
#25240=CARTESIAN_POINT ( 'NONE',  ( 7.711227883964345331, -79.91167364451388266, 7.535872567873190597 ) ) ;
#25241=CARTESIAN_POINT ( 'NONE',  ( -1.780908991550280041, -79.96222016378874287, -11.07474478829885989 ) ) ;
#25242=CARTESIAN_POINT ( 'NONE',  ( 11.92746894621999942, -79.32647392562900279, 1.562891678063999867 ) ) ;
#25245=CARTESIAN_POINT ( 'NONE',  ( 6.793663275700000170, -79.49993983499498995, -8.982210410292001512 ) ) ;
#25262=CARTESIAN_POINT ( 'NONE',  ( -0.006799328100487733902, -79.79999999999998295, 11.99550372483783889 ) ) ;
#25264=CARTESIAN_POINT ( 'NONE',  ( -5.180360735014728490, -80.01521789024674547, 9.419592454460451236 ) ) ;
#25267=CARTESIAN_POINT ( 'NONE',  ( 5.177752511601999785, -76.67058972713098797, 9.912858493839999952 ) ) ;
#25270=CARTESIAN_POINT ( 'NONE',  ( 7.945797842061000260, -76.70274997629699953, 7.770709007203000063 ) ) ;
#25277=CARTESIAN_POINT ( 'NONE',  ( 11.90625000002000000, -76.20625000001498961, 3.701036097655999965E-09 ) ) ;
#25302=CARTESIAN_POINT ( 'NONE',  ( 5.221956912926488670, -79.93484039700992128, 9.402318417155663965 ) ) ;
#25305=LINE ( 'NONE', #43906, #8734 ) ;
#25313=CARTESIAN_POINT ( 'NONE',  ( 10.58601714202000110, -77.46786888426198914, -5.993221192758000804 ) ) ;
#25314=EDGE_LOOP ( 'NONE', ( #51998, #26296, #26035, #27340, #46704 ) ) ;
#25323=CARTESIAN_POINT ( 'NONE',  ( -5.413301372347584461, -80.68336512517144854, -9.391811118427879634 ) ) ;
#25330=CARTESIAN_POINT ( 'NONE',  ( -5.279679587742245772, -80.93583077350247379, -9.889870672231383608 ) ) ;
#25331=CARTESIAN_POINT ( 'NONE',  ( -4.743879332790999825, -78.74260081536296241, -11.00053059214000051 ) ) ;
#25346=CARTESIAN_POINT ( 'NONE',  ( 5.137083998358000336, -77.21100733245999947, -10.56753840748999984 ) ) ;
#25349=CARTESIAN_POINT ( 'NONE',  ( -1.863462560416999869, -77.82837470544299663, 12.02123279331999939 ) ) ;
#25355=CARTESIAN_POINT ( 'NONE',  ( 2.273403379124000026E-14, -92.33215535459000023, 0.000000000000000000 ) ) ;
#25357=CARTESIAN_POINT ( 'NONE',  ( 1.384588047529715649, -78.76581540243206803, 11.96733435986141991 ) ) ;
#25358=CARTESIAN_POINT ( 'NONE',  ( -9.480782379477998845, -79.31267994938899335, -7.608539354584999082 ) ) ;
#25365=CARTESIAN_POINT ( 'NONE',  ( -7.374560639698973574, -77.97291666666664867, -9.596002108778167283 ) ) ;
#25368=CARTESIAN_POINT ( 'NONE',  ( -1.963243971998659854, -76.46084546787545833, -11.01016897788577786 ) ) ;
#25370=CARTESIAN_POINT ( 'NONE',  ( 11.77866768790018703, -79.29209999548564269, -1.141178231376368091 ) ) ;
#25380=CARTESIAN_POINT ( 'NONE',  ( -9.393375537833518862, -78.55837579994272346, 5.413840788339419063 ) ) ;
#25384=CARTESIAN_POINT ( 'NONE',  ( 7.323687853406999793, -76.65218057132500462, 10.23897242151999976 ) ) ;
#25385=CARTESIAN_POINT ( 'NONE',  ( 2.100545712175502455, -78.74077999467331779, -10.54269051299135995 ) ) ;
#25390=CIRCLE ( 'NONE', #40487, 9.599999999999999645 ) ;
#25391=EDGE_CURVE ( 'NONE', #53569, #18786, #17612, .T. ) ;
#25397=CARTESIAN_POINT ( 'NONE',  ( 10.49311453041000064, -80.12294012156499434, -3.963918880051000126 ) ) ;
#25400=B_SPLINE_CURVE_WITH_KNOTS ( 'NONE', 3,
 ( #9556, #27248, #45288, #4835 ),
 .UNSPECIFIED., .F., .F.,
 ( 4, 4 ),
 ( 0.000000000000000000, 1.000000000000000000 ),
 .UNSPECIFIED. ) ;
#25402=EDGE_LOOP ( 'NONE', ( #42266, #33722, #16758, #48174 ) ) ;
#25407=CARTESIAN_POINT ( 'NONE',  ( 9.669078507277122370, -77.14221111144533438, 5.685994177280137230 ) ) ;
#25425=DIRECTION ( 'NONE',  ( -1.000000000000000000, 0.000000000000000000, 0.000000000000000000 ) ) ;
#25426=CARTESIAN_POINT ( 'NONE',  ( 9.789819849890999848, -78.69943487044800179, -6.904744247936999813 ) ) ;
#25433=CARTESIAN_POINT ( 'NONE',  ( 0.5327216036087999429, -77.15547540590999631, -10.90374125898999935 ) ) ;
#25438=CARTESIAN_POINT ( 'NONE',  ( 10.48155006022000002, -79.62010969142899341, 6.381341495520000073 ) ) ;
#25448=CARTESIAN_POINT ( 'NONE',  ( -1.448527388915000103, -78.25544952233700258, -10.72114852740000046 ) ) ;
#25462=ORIENTED_EDGE ( 'NONE', *, *, #47396, .F. ) ;
#25467=CARTESIAN_POINT ( 'NONE',  ( -8.044069603293324988, -81.00000000000001421, -7.290586178141345464 ) ) ;
#25468=CARTESIAN_POINT ( 'NONE',  ( -10.26277353288999983, -77.60109353173099578, -3.721672393288999903 ) ) ;
#25473=CARTESIAN_POINT ( 'NONE',  ( 10.49311453041000064, -79.91957446173628909, -3.963918880051000126 ) ) ;
#25476=ORIENTED_EDGE ( 'NONE', *, *, #19611, .F. ) ;
#25490=CARTESIAN_POINT ( 'NONE',  ( -8.885616033064000163, -78.14317969841199840, 8.035041515002001589 ) ) ;
#25500=CARTESIAN_POINT ( 'NONE',  ( -11.26188033092999952, -77.82385718872900782, -0.06337168221170999538 ) ) ;
#25503=ORIENTED_EDGE ( 'NONE', *, *, #20905, .F. ) ;
#25504=CARTESIAN_POINT ( 'NONE',  ( 10.75000000000000000, -80.25000000000000000, -1.651583051307000043E-14 ) ) ;
#25519=CARTESIAN_POINT ( 'NONE',  ( 10.90309719880000117, -76.87896664909099798, -1.680537371260999890 ) ) ;
#25524=CARTESIAN_POINT ( 'NONE',  ( -3.514441315269281940, -80.19895905850948736, -10.16027557698152428 ) ) ;
#25527=CARTESIAN_POINT ( 'NONE',  ( -10.71617508045257594, -79.82603844877975519, 3.314392947253207211 ) ) ;
#25529=CARTESIAN_POINT ( 'NONE',  ( 0.4713521909880000194, -78.87019817133499089, 12.02020425643999957 ) ) ;
#25531=CARTESIAN_POINT ( 'NONE',  ( 7.840078887343000069, -79.00968566096200618, -8.084993976410000727 ) ) ;
#25550=CARTESIAN_POINT ( 'NONE',  ( -10.18724605009749773, -80.07418096558578213, 3.432876765056549484 ) ) ;
#25553=CARTESIAN_POINT ( 'NONE',  ( -5.007180289739999068, -76.81362410637399307, 10.00009952528999868 ) ) ;
#25557=CARTESIAN_POINT ( 'NONE',  ( -10.67862928275000023, -76.94605063463400541, 1.734397297249000047 ) ) ;
#25564=CARTESIAN_POINT ( 'NONE',  ( -2.281880833369933193, -77.99216318363434652, 10.50503500748997254 ) ) ;
#25580=CARTESIAN_POINT ( 'NONE',  ( -5.059370734576000395, -80.83793477179669651, -10.06538451635999998 ) ) ;
#25588=DIRECTION ( 'NONE',  ( 0.000000000000000000, 1.000000000000000000, 0.000000000000000000 ) ) ;
#25590=EDGE_CURVE ( 'NONE', #36999, #35854, #40240, .T. ) ;
#25616=CARTESIAN_POINT ( 'NONE',  ( 11.59999999999999964, -87.70000000000000284, 0.000000000000000000 ) ) ;
#25618=CARTESIAN_POINT ( 'NONE',  ( -10.77837019794128182, -80.37202936742626491, -3.084047917684326290 ) ) ;
#25619=CARTESIAN_POINT ( 'NONE',  ( -8.148905501844001975, -78.71547149993911319, -8.781309899900000104 ) ) ;
#25627=CARTESIAN_POINT ( 'NONE',  ( -1.984586691443999795, -75.95454648948098964, 11.75553522549000007 ) ) ;
#25630=EDGE_CURVE ( 'NONE', #19148, #3745, #14777, .T. ) ;
#25634=CARTESIAN_POINT ( 'NONE',  ( 12.00000000000000000, -78.64999999999999147, 0.000000000000000000 ) ) ;
#25636=CARTESIAN_POINT ( 'NONE',  ( -7.209427067528999977, -77.43490340765200131, 9.655047023863000177 ) ) ;
#25641=CARTESIAN_POINT ( 'NONE',  ( -10.57143388931192263, -79.58561314518549068, 1.950965474043120151 ) ) ;
#25644=CARTESIAN_POINT ( 'NONE',  ( 1.328997109577999991, -79.39258084193100728, -12.08341310737000107 ) ) ;
#25646=CARTESIAN_POINT ( 'NONE',  ( 11.88845611680340220, -79.66250000000000853, 1.884907306722996445 ) ) ;
#25654=CARTESIAN_POINT ( 'NONE',  ( 7.065231863527838385, -79.37355030446100557, 9.414959857278416777 ) ) ;
#25666=AXIS2_PLACEMENT_3D ( 'NONE', #8828, #13242, #21811 ) ;
#25668=CARTESIAN_POINT ( 'NONE',  ( 10.47049206515227660, -78.37083834417222761, 2.813954660210043812 ) ) ;
#25673=CARTESIAN_POINT ( 'NONE',  ( -11.56560577205999962, -76.78936719843599690, -4.664037835044000602 ) ) ;
#25674=CARTESIAN_POINT ( 'NONE',  ( 4.240041242285670364, -78.75727277875573407, -9.878621513098671869 ) ) ;
#25680=PRODUCT_DEFINITION_CONTEXT ( 'detailed design', #52268, 'design' ) ;
#25684=CARTESIAN_POINT ( 'NONE',  ( -1.472820794058999905, -78.51599588445799327, -10.90095403661999995 ) ) ;
#25712=CARTESIAN_POINT ( 'NONE',  ( 4.374544387491000386, -77.22085244456999931, -11.15253550093999912 ) ) ;
#25715=CARTESIAN_POINT ( 'NONE',  ( -6.036864304657779456, -76.31631156611008748, 10.44601093413916537 ) ) ;
#25718=B_SPLINE_CURVE_WITH_KNOTS ( 'NONE', 3,
 ( #49733, #36714, #9570, #41147 ),
 .UNSPECIFIED., .F., .F.,
 ( 4, 4 ),
 ( 0.000000000000000000, 1.000000000000000000 ),
 .UNSPECIFIED. ) ;
#25719=CARTESIAN_POINT ( 'NONE',  ( -10.74996386890631328, -76.59758012670684479, 0.3350321142958054277 ) ) ;
#25727=LINE ( 'NONE', #3869, #56870 ) ;
#25729=CARTESIAN_POINT ( 'NONE',  ( 0.000000000000000000, -90.29999999999999716, 0.000000000000000000 ) ) ;
#25730=CARTESIAN_POINT ( 'NONE',  ( 8.322242302276999126, -76.25751096588899713, 9.174819693653001096 ) ) ;
#25734=CARTESIAN_POINT ( 'NONE',  ( 10.95738943370000129, -78.88188541137900245, -1.279590238973999927 ) ) ;
#25752=DIRECTION ( 'NONE',  ( 0.000000000000000000, 1.000000000000000000, 0.000000000000000000 ) ) ;
#25762=CARTESIAN_POINT ( 'NONE',  ( 0.2583767295277000220, -78.20029307777100769, -10.91369642039000176 ) ) ;
#25766=CARTESIAN_POINT ( 'NONE',  ( 2.315902194296999728, -78.33986656763099177, -10.97517055051999968 ) ) ;
#25771=FACE_OUTER_BOUND ( 'NONE', #20815, .T. ) ;
#25777=CARTESIAN_POINT ( 'NONE',  ( 0.000000000000000000, -87.64999999984398471, -9.649999999844000698 ) ) ;
#25781=EDGE_CURVE ( 'NONE', #26795, #2543, #43991, .T. ) ;
#25787=SURFACE_STYLE_FILL_AREA ( #39371 ) ;
#25788=CARTESIAN_POINT ( 'NONE',  ( -10.86494198988000015, -78.40907477017699989, -2.491513063939999828 ) ) ;
#25790=CARTESIAN_POINT ( 'NONE',  ( 5.504720026230000229, -80.98993105630589184, -9.574706785621000193 ) ) ;
#25808=CARTESIAN_POINT ( 'NONE',  ( 10.83471462526000018, -76.90620299209300015, 2.076220934837999632 ) ) ;
#25814=CARTESIAN_POINT ( 'NONE',  ( 0.08637108029348440630, -80.22590001772620383, -10.74954481972912745 ) ) ;
#25818=CARTESIAN_POINT ( 'NONE',  ( 4.847151869481000297, -78.90810309376399800, 11.00961342987999991 ) ) ;
#25820=CARTESIAN_POINT ( 'NONE',  ( -7.438698978239999704, -79.39099446298800444, -8.455750828251000328 ) ) ;
#25821=CARTESIAN_POINT ( 'NONE',  ( -3.463637548850266867, -77.50106921249592062, 10.20060348489307600 ) ) ;
#25835=ORIENTED_EDGE ( 'NONE', *, *, #47673, .F. ) ;
#25837=CARTESIAN_POINT ( 'NONE',  ( 9.148037756630525763, -79.79999999999999716, 7.522470651702480637 ) ) ;
#25839=CARTESIAN_POINT ( 'NONE',  ( -4.817876235597053913, -80.01207991527530794, 9.609839989271527827 ) ) ;
#25845=CARTESIAN_POINT ( 'NONE',  ( 8.187817122061000319, -76.13338407210200387, 7.683968774170000238 ) ) ;
#25870=CARTESIAN_POINT ( 'NONE',  ( 0.000000000000000000, -90.35000000009100063, 0.000000000000000000 ) ) ;
#25906=CARTESIAN_POINT ( 'NONE',  ( 10.69384760718000038, -78.36279039943012492, -5.399785902169999652 ) ) ;
#25923=CARTESIAN_POINT ( 'NONE',  ( -7.806617969149999503, -78.30323394950599436, 9.479055599837000301 ) ) ;
#25928=CARTESIAN_POINT ( 'NONE',  ( -8.375467055228931201, -79.54614502533394216, 6.744101667046974669 ) ) ;
#25930=CARTESIAN_POINT ( 'NONE',  ( -10.87922314793346068, -78.86468826379788766, 5.174618772388030585 ) ) ;
#25931=CARTESIAN_POINT ( 'NONE',  ( -12.04098616622999884, -79.19168562328098915, -0.08309486781487000762 ) ) ;
#25934=CARTESIAN_POINT ( 'NONE',  ( 8.512781221943589216, -79.71249999999999147, 8.510042318544764228 ) ) ;
#25946=EDGE_CURVE ( 'NONE', #55197, #20755, #14530, .T. ) ;
#25959=CARTESIAN_POINT ( 'NONE',  ( 11.30982802994000025, -76.54347076860699417, 5.253977129081000008 ) ) ;
#25966=CARTESIAN_POINT ( 'NONE',  ( 1.508420534579999917, -77.61426645450845285, 11.11497989571999767 ) ) ;
#25969=CARTESIAN_POINT ( 'NONE',  ( 11.21665020278000036, -78.65217759946699516, 0.06973997782872000395 ) ) ;
#25977=CARTESIAN_POINT ( 'NONE',  ( 6.252156853421744209, -77.06842338808830561, -10.30345392412948158 ) ) ;
#25988=CARTESIAN_POINT ( 'NONE',  ( -2.813789756862300262, -77.89583333333332860, 10.47020627418438465 ) ) ;
#25994=CARTESIAN_POINT ( 'NONE',  ( -0.08519377839585000334, -78.37388308536300485, 11.97951611939999950 ) ) ;
#25998=CARTESIAN_POINT ( 'NONE',  ( 6.013200962235000446, -77.90957020342199257, 10.30906962990999887 ) ) ;
#26006=CARTESIAN_POINT ( 'NONE',  ( 5.273774136544999713, -79.48694153719199562, -11.08023994795000000 ) ) ;
#26011=CARTESIAN_POINT ( 'NONE',  ( -2.510140451105999926, -77.04989847029199268, -12.13002842542999993 ) ) ;
#26015=CARTESIAN_POINT ( 'NONE',  ( -9.643902624173000149, -79.18148518439899419, -5.356946570292000054 ) ) ;
#26023=CARTESIAN_POINT ( 'NONE',  ( -12.15819904699000098, -78.83780308901600620, -1.724521706148000044 ) ) ;
#26026=CARTESIAN_POINT ( 'NONE',  ( -10.75000000000000000, -79.50000000000000000, 0.000000000000000000 ) ) ;
#26035=ORIENTED_EDGE ( 'NONE', *, *, #9718, .T. ) ;
#26038=CARTESIAN_POINT ( 'NONE',  ( -9.684478921172445354, -81.00000000000000000, -4.805145260639483773 ) ) ;
#26039=CARTESIAN_POINT ( 'NONE',  ( -10.66734455299000039, -77.05636667169498821, 2.320156498608999751 ) ) ;
#26043=CARTESIAN_POINT ( 'NONE',  ( 11.21485848424000054, -80.01459935801440793, -0.2123177049684000228 ) ) ;
#26045=ORIENTED_EDGE ( 'NONE', *, *, #50594, .F. ) ;
#26058=CARTESIAN_POINT ( 'NONE',  ( -9.608132404413000316, -79.02473885956399613, 7.328251847290000676 ) ) ;
#26059=DIRECTION ( 'NONE',  ( 1.000000000000000000, 0.000000000000000000, 0.000000000000000000 ) ) ;
#26060=CARTESIAN_POINT ( 'NONE',  ( 10.18066396183999878, -78.49586079892000612, 6.314281093748000728 ) ) ;
#26069=CARTESIAN_POINT ( 'NONE',  ( 9.909229536192000865, -77.03400324167699864, -5.351741263869000065 ) ) ;
#26071=CARTESIAN_POINT ( 'NONE',  ( -3.214200885120999995, -80.72145419626957619, 10.78715111662000048 ) ) ;
#26073=ADVANCED_FACE ( 'NONE', ( #14239 ), #53475, .F. ) ;
#26090=CARTESIAN_POINT ( 'NONE',  ( -5.822924921437000023, -77.62760228854999411, 9.505164171658000427 ) ) ;
#26097=CARTESIAN_POINT ( 'NONE',  ( 2.601259834223990097, -80.24469330578341442, -10.43116776099581244 ) ) ;
#26101=CARTESIAN_POINT ( 'NONE',  ( -8.850953919802000414, -79.55752168082800324, -8.146641040006999290 ) ) ;
#26103=CARTESIAN_POINT ( 'NONE',  ( 8.858182419534999852, -80.12637572403669139, 6.954620140474000678 ) ) ;
#26108=EDGE_CURVE ( 'NONE', #42165, #3688, #43111, .T. ) ;
#26116=CARTESIAN_POINT ( 'NONE',  ( -10.42930648941000094, -79.54953960801499591, 3.225667704544000092 ) ) ;
#26128=CARTESIAN_POINT ( 'NONE',  ( 7.720144650974280154, -79.79999999999998295, 9.058211719984365473 ) ) ;
#26129=CARTESIAN_POINT ( 'NONE',  ( -8.684598835271984285, -80.05006380143068156, 6.335413721204657733 ) ) ;
#26133=CARTESIAN_POINT ( 'NONE',  ( 8.154961773732001262, -76.21165749863600070, 7.653135223926000208 ) ) ;
#26136=CARTESIAN_POINT ( 'NONE',  ( 9.615022378355000399, -76.16851043297199908, -5.341629093326000444 ) ) ;
#26149=CARTESIAN_POINT ( 'NONE',  ( -6.606377239730343298, -80.07291666666665719, -8.596418555780429571 ) ) ;
#26168=CARTESIAN_POINT ( 'NONE',  ( 1.808012550523518946, -79.96190839373853976, 10.59665058875179788 ) ) ;
#26188=EDGE_LOOP ( 'NONE', ( #32353, #26320, #14289, #42556, #22325, #48218, #32866, #35651 ) ) ;
#26194=DIRECTION ( 'NONE',  ( 1.000000000000000000, 0.000000000000000000, 0.000000000000000000 ) ) ;
#26196=CARTESIAN_POINT ( 'NONE',  ( -3.097937178131073832, -80.45257242543718235, -10.77438633444702809 ) ) ;
#26203=AXIS2_PLACEMENT_3D ( 'NONE', #1159, #4697, #14697 ) ;
#26208=CARTESIAN_POINT ( 'NONE',  ( -8.866178467950035724, -78.14940218639688396, -6.303320502543174442 ) ) ;
#26213=CARTESIAN_POINT ( 'NONE',  ( 7.671012283914000029, -78.19471668781000062, 9.589126640163000204 ) ) ;
#26215=EDGE_CURVE ( 'NONE', #46084, #57578, #17524, .T. ) ;
#26219=CARTESIAN_POINT ( 'NONE',  ( -8.824274837635110558, -79.55161701906600058, 6.149812313655782070 ) ) ;
#26222=CARTESIAN_POINT ( 'NONE',  ( -9.391088595540001194, -79.24495288497600143, -7.536558092107000562 ) ) ;
#26223=ADVANCED_FACE ( 'NONE', ( #26485 ), #29762, .F. ) ;
#26224=CARTESIAN_POINT ( 'NONE',  ( -5.908174908109000256, -80.99493105630590151, 8.927771479942999022 ) ) ;
#26225=DIRECTION ( 'NONE',  ( -1.000000000000000000, 0.000000000000000000, 0.000000000000000000 ) ) ;
#26231=ORIENTED_EDGE ( 'NONE', *, *, #41232, .T. ) ;
#26250=CARTESIAN_POINT ( 'NONE',  ( -6.054010968653000369, -76.10689905944899181, 10.76718068125000016 ) ) ;
#26259=CARTESIAN_POINT ( 'NONE',  ( 3.113304451009999863, -78.39783470746900207, -10.55022916317000181 ) ) ;
#26262=CARTESIAN_POINT ( 'NONE',  ( 7.910349975595998728, -79.71439497653800288, 7.952639426948999279 ) ) ;
#26281=CARTESIAN_POINT ( 'NONE',  ( -10.75000000000000355, -77.98958333333328596, 1.407171709420384609 ) ) ;
#26286=CARTESIAN_POINT ( 'NONE',  ( -11.48784787867999846, -78.02120198485400238, -3.397854551190000016 ) ) ;
#26290=CARTESIAN_POINT ( 'NONE',  ( -3.073538647258000189, -78.18086335765900685, -11.53207971834999945 ) ) ;
#26296=ORIENTED_EDGE ( 'NONE', *, *, #56573, .T. ) ;
#26303=CARTESIAN_POINT ( 'NONE',  ( 4.699868689641999886, -76.59710561063300815, -11.46072718019999925 ) ) ;
#26307=CARTESIAN_POINT ( 'NONE',  ( 10.56933735542999919, -79.98459350986080096, 3.541701167072000445 ) ) ;
#26315=CARTESIAN_POINT ( 'NONE',  ( -12.03507225495000199, -78.81067377359200066, 2.439839133843999974 ) ) ;
#26320=ORIENTED_EDGE ( 'NONE', *, *, #40880, .T. ) ;
#26331=CARTESIAN_POINT ( 'NONE',  ( 10.58946819037999987, -78.42157559663600352, -3.698823201301000285 ) ) ;
#26342=EDGE_CURVE ( 'NONE', #54085, #40725, #4333, .T. ) ;
#26346=ADVANCED_FACE ( 'NONE', ( #35937 ), #2584, .F. ) ;
#26347=CARTESIAN_POINT ( 'NONE',  ( -0.4643318395057000059, -79.19853201380200858, -12.07492461931999905 ) ) ;
#26356=CARTESIAN_POINT ( 'NONE',  ( 6.355487164442999770, -78.15069330475100173, 9.297405415548999130 ) ) ;
#26358=CARTESIAN_POINT ( 'NONE',  ( 9.871112813097001393, -80.53352039424419218, -5.408775127089999302 ) ) ;
#26364=CARTESIAN_POINT ( 'NONE',  ( 6.329984427697000093, -78.02560107145599488, 9.260097609460000712 ) ) ;
#26372=DIRECTION ( 'NONE',  ( 0.000000000000000000, 1.000000000000000000, 0.000000000000000000 ) ) ;
#26374=CARTESIAN_POINT ( 'NONE',  ( 3.871217329169000188, -77.05563908551199859, 10.45314674924000009 ) ) ;
#26380=CARTESIAN_POINT ( 'NONE',  ( -5.959306489951042174, -80.17831636609369639, -8.946966000018207410 ) ) ;
#26386=CARTESIAN_POINT ( 'NONE',  ( -10.75919966670999983, -79.79953960801499591, 3.327699969971999572 ) ) ;
#26394=EDGE_CURVE ( 'NONE', #46546, #55386, #19118, .T. ) ;
#26397=CARTESIAN_POINT ( 'NONE',  ( -1.733234625524999961, -79.68572132302399780, -10.77827740047999860 ) ) ;
#26422=CARTESIAN_POINT ( 'NONE',  ( 3.399186938124000079, -81.00000000000000000, -10.46162167925000119 ) ) ;
#26436=ORIENTED_EDGE ( 'NONE', *, *, #12281, .T. ) ;
#26446=CARTESIAN_POINT ( 'NONE',  ( -4.671140612849559837, -77.18924933319441095, -9.682078454169923631 ) ) ;
#26455=VERTEX_POINT ( 'NONE', #55418 ) ;
#26456=CARTESIAN_POINT ( 'NONE',  ( 6.482586803565999922, -77.86134018205299867, -10.15735398655000132 ) ) ;
#26461=CARTESIAN_POINT ( 'NONE',  ( -12.00000000000000355, -78.78958333333331154, 1.570796326794848596 ) ) ;
#26465=CIRCLE ( 'NONE', #56670, 13.89999999999999858 ) ;
#26467=FACE_OUTER_BOUND ( 'NONE', #46780, .T. ) ;
#26485=FACE_OUTER_BOUND ( 'NONE', #54010, .T. ) ;
#26492=EDGE_CURVE ( 'NONE', #41938, #14498, #56494, .T. ) ;
#26493=CARTESIAN_POINT ( 'NONE',  ( -8.494907789873000326, -76.97389978589799853, 6.628721719457000283 ) ) ;
#26494=CARTESIAN_POINT ( 'NONE',  ( -11.33781659400000130, -77.84203558730200712, 4.716958136547999558 ) ) ;
#26501=CARTESIAN_POINT ( 'NONE',  ( 7.482400665469000067, -80.95774006270789869, 8.296818276455001140 ) ) ;
#26502=DIRECTION ( 'NONE',  ( -1.000000000000000000, 0.000000000000000000, 0.000000000000000000 ) ) ;
#26512=EDGE_CURVE ( 'NONE', #6742, #34745, #13493, .T. ) ;
#26519=VECTOR ( 'NONE', #26770, 1000.000000000000114 ) ;
#26530=CARTESIAN_POINT ( 'NONE',  ( 12.02981475616999951, -76.85882676113499201, -2.229486315987000200 ) ) ;
#26533=ORIENTED_EDGE ( 'NONE', *, *, #22959, .F. ) ;
#26538=CARTESIAN_POINT ( 'NONE',  ( -6.984027423103999155, -77.17848496647944501, 8.777327129872999123 ) ) ;
#26541=CARTESIAN_POINT ( 'NONE',  ( 10.93160348586000019, -79.16966811650100055, 2.513594203403000105 ) ) ;
#26551=CARTESIAN_POINT ( 'NONE',  ( 4.297951556683999641, -76.85513471105899441, -11.50435740523999861 ) ) ;
#26552=CARTESIAN_POINT ( 'NONE',  ( -9.599999999916001059, -90.40000000008399184, 6.531558194539000517E-10 ) ) ;
#26556=CARTESIAN_POINT ( 'NONE',  ( 9.393203674808285442, -79.70833333333332860, -5.413904038987152667 ) ) ;
#26557=CARTESIAN_POINT ( 'NONE',  ( 7.358951392786451606, -80.06693380409777205, 8.232011333706584111 ) ) ;
#26563=CARTESIAN_POINT ( 'NONE',  ( 11.81379047889000056, -77.26158115298899531, 1.987564636421000008 ) ) ;
#26566=CARTESIAN_POINT ( 'NONE',  ( 5.516244905679999810, -78.91335487410098892, 10.58329673088999989 ) ) ;
#26574=CARTESIAN_POINT ( 'NONE',  ( -8.960630775719000241, -79.88644599990469430, -8.384004251637000138 ) ) ;
#26577=CARTESIAN_POINT ( 'NONE',  ( -10.05535668103000191, -78.29735989301799748, 4.970705447719999448 ) ) ;
#26580=CARTESIAN_POINT ( 'NONE',  ( -12.36215275698000049, -76.44617465741299611, -0.7837170484252999891 ) ) ;
#26584=CARTESIAN_POINT ( 'NONE',  ( -2.801579282652000291, -78.74570369637000056, -10.67018687299000135 ) ) ;
#26592=CARTESIAN_POINT ( 'NONE',  ( 2.765208115035000080, -77.96966499545499119, -11.96450597650000169 ) ) ;
#26605=CARTESIAN_POINT ( 'NONE',  ( -10.41264997627000000, -77.61434791013999757, 3.643961423121000021 ) ) ;
#26609=VECTOR ( 'NONE', #40987, 1000.000000000000000 ) ;
#26610=CARTESIAN_POINT ( 'NONE',  ( -11.20683111097000051, -79.76947227099799420, -0.4743912329535999728 ) ) ;
#26612=EDGE_CURVE ( 'NONE', #31953, #18786, #19342, .T. ) ;
#26629=CARTESIAN_POINT ( 'NONE',  ( 7.613064433753999438, -78.76183641763000765, 9.349774124741999870 ) ) ;
#26631=CARTESIAN_POINT ( 'NONE',  ( -6.121609607564330702, -78.02338199628493953, 8.836716547392137855 ) ) ;
#26632=CARTESIAN_POINT ( 'NONE',  ( -11.06076315227999984, -78.10252046055900621, 4.601693484369000053 ) ) ;
#26640=CARTESIAN_POINT ( 'NONE',  ( -7.012165219465999577, -77.25189398569099808, 8.812689912465000219 ) ) ;
#26643=VERTEX_POINT ( 'NONE', #40902 ) ;
#26655=CYLINDRICAL_SURFACE ( 'NONE', #9407, 14.00000000000000000 ) ;
#26656=B_SPLINE_CURVE_WITH_KNOTS ( 'NONE', 3,
 ( #52261, #15951, #33070, #33941, #51981, #29225, #28351, #24522, #2677, #51115 ),
 .UNSPECIFIED., .F., .F.,
 ( 4, 2, 2, 2, 4 ),
 ( 0.000000000000000000, 0.2500000000000001665, 0.5000000000000002220, 0.7500000000000001110, 1.000000000000000000 ),
 .UNSPECIFIED. ) ;
#26661=CARTESIAN_POINT ( 'NONE',  ( -10.62993649278000063, -77.74980203896600983, 3.720001978191000092 ) ) ;
#26668=CARTESIAN_POINT ( 'NONE',  ( 0.9450957028779182201, -80.23244768896006462, -10.70949845984780957 ) ) ;
#26670=CARTESIAN_POINT ( 'NONE',  ( 11.14131185284651160, -79.09065718773078402, -1.301068469138584760 ) ) ;
#26675=DIRECTION ( 'NONE',  ( -1.000000000000000000, 0.000000000000000000, 0.000000000000000000 ) ) ;
#26676=CARTESIAN_POINT ( 'NONE',  ( -1.646570173782999857, -78.71008588794200023, 11.14103995232000166 ) ) ;
#26680=EDGE_CURVE ( 'NONE', #10296, #5424, #48635, .T. ) ;
#26682=ORIENTED_EDGE ( 'NONE', *, *, #17037, .T. ) ;
#26687=CARTESIAN_POINT ( 'NONE',  ( 1.081678475801000072, -79.50832130042100232, 10.97869327635999781 ) ) ;
#26688=CARTESIAN_POINT ( 'NONE',  ( 6.043427764450807871, -76.46666666664967238, -10.48543666025108934 ) ) ;
#26698=VECTOR ( 'NONE', #421, 1000.000000000000114 ) ;
#26710=CYLINDRICAL_SURFACE ( 'NONE', #52499, 11.59999999999999964 ) ;
#26716=CARTESIAN_POINT ( 'NONE',  ( -0.8496252788811309298, -80.98142198267933622, 10.71628590444292328 ) ) ;
#26717=CARTESIAN_POINT ( 'NONE',  ( 6.985849709488999970, -81.07991142482880775, -8.837815942395002011 ) ) ;
#26740=CARTESIAN_POINT ( 'NONE',  ( 7.631340703017165161, -77.28798361778574133, -7.571206356639036628 ) ) ;
#26746=VECTOR ( 'NONE', #44336, 1000.000000000000000 ) ;
#26748=CARTESIAN_POINT ( 'NONE',  ( -10.61206674237698522, -80.48532644614452636, 1.982131822504892060 ) ) ;
#26750=EDGE_CURVE ( 'NONE', #7386, #27557, #56519, .T. ) ;
#26751=CARTESIAN_POINT ( 'NONE',  ( -3.566334030200000171, -77.59004702781498963, 11.50986677841000017 ) ) ;
#26758=B_SPLINE_CURVE_WITH_KNOTS ( 'NONE', 3,
 ( #5125, #41129, #27244, #5691, #14254, #19284, #27535, #45283, #49715, #36403, #9259, #4831, #55288, #18700, #40842, #436, #50880, #54431 ),
 .UNSPECIFIED., .F., .F.,
 ( 4, 2, 2, 2, 2, 2, 2, 2, 4 ),
 ( 0.000000000000000000, 0.1249999999999999445, 0.2499999999999998890, 0.3749999999999998335, 0.4999999999999998890, 0.6249999999999998890, 0.7500000000000000000, 0.8750000000000000000, 1.000000000000000000 ),
 .UNSPECIFIED. ) ;
#26768=CIRCLE ( 'NONE', #33400, 12.00000000000000000 ) ;
#26770=DIRECTION ( 'NONE',  ( -1.186310310053999794E-10, -0.9999999999999998890, 1.114594443524999723E-08 ) ) ;
#26773=AXIS2_PLACEMENT_3D ( 'NONE', #29920, #48257, #29064 ) ;
#26788=CARTESIAN_POINT ( 'NONE',  ( 10.72166763895999964, -77.29165712091899820, 2.054558110510000368 ) ) ;
#26790=CARTESIAN_POINT ( 'NONE',  ( 11.98062200086999951, -77.17727113527298854, -2.108850158091000182 ) ) ;
#26795=VERTEX_POINT ( 'NONE', #7503 ) ;
#26799=CARTESIAN_POINT ( 'NONE',  ( 2.332976527971999836, -80.78287663268979202, -10.92616016422999969 ) ) ;
#26802=CARTESIAN_POINT ( 'NONE',  ( 10.29113596735999892, -77.61645131797199326, 4.462133020506000136 ) ) ;
#26820=DIRECTION ( 'NONE',  ( 0.000000000000000000, 0.000000000000000000, -1.000000000000000000 ) ) ;
#26825=ORIENTED_EDGE ( 'NONE', *, *, #2994, .F. ) ;
#26827=CARTESIAN_POINT ( 'NONE',  ( 5.491357861347999858, -76.35279548927898929, -11.06493742798000035 ) ) ;
#26828=ADVANCED_FACE ( 'NONE', ( #39656 ), #18706, .F. ) ;
#26829=CARTESIAN_POINT ( 'NONE',  ( -10.74991479005951511, -78.60500528859236624, -0.6569711721753703770 ) ) ;
#26837=CARTESIAN_POINT ( 'NONE',  ( 4.275724345439000373, -76.90612153646102911, -10.36997068233999997 ) ) ;
#26840=CARTESIAN_POINT ( 'NONE',  ( 7.808618912244999599, -79.08795908749598880, -8.052551227705000869 ) ) ;
#26851=CARTESIAN_POINT ( 'NONE',  ( 0.000000000000000000, -90.39999999999999147, 0.000000000000000000 ) ) ;
#26856=CARTESIAN_POINT ( 'NONE',  ( 10.75000000000000355, -79.73958333333332860, -1.407171709420407035 ) ) ;
#26865=CARTESIAN_POINT ( 'NONE',  ( 11.79843486695000010, -77.23445183756500398, -2.076781258317999868 ) ) ;
#26866=DIRECTION ( 'NONE',  ( 0.000000000000000000, -1.000000000000000000, 0.000000000000000000 ) ) ;
#26867=CARTESIAN_POINT ( 'NONE',  ( -7.587128856971000701, -78.50641514274398958, 9.212544607993001122 ) ) ;
#26872=CARTESIAN_POINT ( 'NONE',  ( 10.36875976864000037, -78.73659464476099856, 3.767035497191999927 ) ) ;
#26883=CARTESIAN_POINT ( 'NONE',  ( -2.577162953934999834, -76.40070350691199508, 11.99607385716000074 ) ) ;
#26887=CARTESIAN_POINT ( 'NONE',  ( 2.301467643382999917, -78.35041292975199667, -10.90676452780999917 ) ) ;
#26893=CARTESIAN_POINT ( 'NONE',  ( -4.392572548562998058, -76.40833333333333144, 9.875985572401290824 ) ) ;
#26895=CARTESIAN_POINT ( 'NONE',  ( 11.48873525783000105, -78.10531157257399570, 4.336443399433000501 ) ) ;
#26897=CARTESIAN_POINT ( 'NONE',  ( -1.407171709420465211, -78.38541666666665719, 10.74999999999999467 ) ) ;
#26898=CIRCLE ( 'NONE', #24093, 14.00000000000000000 ) ;
#26899=CARTESIAN_POINT ( 'NONE',  ( 11.99999999999999822, -77.06041666666665435, 1.570796326794923203 ) ) ;
#26902=LINE ( 'NONE', #35461, #26746 ) ;
#26911=CARTESIAN_POINT ( 'NONE',  ( 7.808618912244999599, -78.88459342766699933, -8.052551227705000869 ) ) ;
#26912=CARTESIAN_POINT ( 'NONE',  ( 1.218717449224264060, -80.99999999999998579, 10.73986708482796004 ) ) ;
#26920=EDGE_CURVE ( 'NONE', #2879, #55386, #42380, .T. ) ;
#26923=DIRECTION ( 'NONE',  ( -1.776356839400000238E-14, 1.000000000000000000, 0.000000000000000000 ) ) ;
#26929=CARTESIAN_POINT ( 'NONE',  ( 2.810698055981000198, -79.58445734768899626, -11.99191332196000026 ) ) ;
#26930=CARTESIAN_POINT ( 'NONE',  ( -3.256465705460000137, -76.60672286667698927, 11.02300886902000165 ) ) ;
#26931=CARTESIAN_POINT ( 'NONE',  ( -6.868574835607371476, -78.03023875518719876, 8.269499650932843338 ) ) ;
#26932=CARTESIAN_POINT ( 'NONE',  ( -3.085175050843000477, -78.23816703767799652, -11.57574012064000080 ) ) ;
#26938=CARTESIAN_POINT ( 'NONE',  ( -10.47919054151000040, -77.91882059614400191, -3.800153439748000128 ) ) ;
#26939=CARTESIAN_POINT ( 'NONE',  ( -11.68767212001979594, -78.27916666666664014, 3.140974612311315806 ) ) ;
#26940=CARTESIAN_POINT ( 'NONE',  ( -6.515767037275000284, -80.39928196422599171, -9.178153216127999059 ) ) ;
#26942=CARTESIAN_POINT ( 'NONE',  ( 3.066117107042321432, -78.29792545123773095, -10.39032517820746904 ) ) ;
#26947=CARTESIAN_POINT ( 'NONE',  ( -8.728447447808001414, -76.64562635936398749, 6.810956705545000212 ) ) ;
#26959=CARTESIAN_POINT ( 'NONE',  ( -4.503658352096000073, -77.30076617252800020, -10.19664954867000084 ) ) ;
#26965=CARTESIAN_POINT ( 'NONE',  ( -8.308818416638949600, -80.15545485398178016, -6.893652871022299067 ) ) ;
#26966=CARTESIAN_POINT ( 'NONE',  ( -10.75000000000000000, -77.00000000000000000, 0.000000000000000000 ) ) ;
#26967=CARTESIAN_POINT ( 'NONE',  ( -7.301296477453766087, -79.28131158874371920, 8.515437670024562422 ) ) ;
#26970=CARTESIAN_POINT ( 'NONE',  ( 8.767647372505999570, -80.19410278844959805, 6.883540450345000394 ) ) ;
#26982=CARTESIAN_POINT ( 'NONE',  ( 8.413030999918001740, -79.83515741644239938, -7.136010437995999212 ) ) ;
#27001=CARTESIAN_POINT ( 'NONE',  ( 5.039215783544999994, -76.86328604711199830, 9.647628555108001436 ) ) ;
#27006=CARTESIAN_POINT ( 'NONE',  ( 9.755626371838998168, -81.04222055755619181, -5.633583086437000453 ) ) ;
#27025=CARTESIAN_POINT ( 'NONE',  ( -9.700000000000001066, -87.70000000000000284, 0.000000000000000000 ) ) ;
#27035=CARTESIAN_POINT ( 'NONE',  ( 0.07998295410073143208, -77.22568207807030660, -10.74969477503664628 ) ) ;
#27039=CARTESIAN_POINT ( 'NONE',  ( -0.7406579117306999471, -79.58158555557200486, 12.00660533699000077 ) ) ;
#27041=CARTESIAN_POINT ( 'NONE',  ( -9.667451473995011924, -80.46331611536132300, 4.804704892540419436 ) ) ;
#27042=CONICAL_SURFACE ( 'NONE', #24236, 9.649999999909001147, 0.7853981633972997312 ) ;
#27044=CARTESIAN_POINT ( 'NONE',  ( 11.86727826211999925, -77.42727113527298854, -2.088899193827999934 ) ) ;
#27048=ORIENTED_EDGE ( 'NONE', *, *, #31274, .T. ) ;
#27050=CARTESIAN_POINT ( 'NONE',  ( -7.374560639699022424, -78.72708333333335418, 9.596002108778135309 ) ) ;
#27056=CARTESIAN_POINT ( 'NONE',  ( -11.79643810520695268, -79.79999999999996874, -2.072837582963935166 ) ) ;
#27077=CARTESIAN_POINT ( 'NONE',  ( -5.770029083771401446, -78.18019031253406581, -9.108371886169937426 ) ) ;
#27080=EDGE_CURVE ( 'NONE', #9151, #33152, #57104, .T. ) ;
#27085=CARTESIAN_POINT ( 'NONE',  ( -7.595061814885000651, -78.46281986999699143, 7.841581601742999119 ) ) ;
#27086=CARTESIAN_POINT ( 'NONE',  ( 10.43567240482000003, -78.16758737238698984, 6.472443173969999464 ) ) ;
#27092=ORIENTED_EDGE ( 'NONE', *, *, #27920, .F. ) ;
#27094=CARTESIAN_POINT ( 'NONE',  ( 11.65878804082999842, -79.39029486734300178, 2.511675558105000317 ) ) ;
#27095=CARTESIAN_POINT ( 'NONE',  ( 8.467741319088000651, -79.87580510418969482, 6.550495500029000162 ) ) ;
#27120=EDGE_LOOP ( 'NONE', ( #41016, #56520, #54378, #36199 ) ) ;
#27121=CARTESIAN_POINT ( 'NONE',  ( 12.31302258087999846, -76.43476096588899793, -0.9885975245223000973 ) ) ;
#27122=CARTESIAN_POINT ( 'NONE',  ( -9.562223587057937735, -78.63793111567514416, -4.911682745217511581 ) ) ;
#27124=ORIENTED_EDGE ( 'NONE', *, *, #14268, .T. ) ;
#27130=CARTESIAN_POINT ( 'NONE',  ( -4.531904799950999596, -77.34190302449002274, -10.26060180864999971 ) ) ;
#27142=CARTESIAN_POINT ( 'NONE',  ( -12.00000000000000000, -78.39999999999999147, 0.000000000000000000 ) ) ;
#27145=LINE ( 'NONE', #8567, #43626 ) ;
#27147=ORIENTED_EDGE ( 'NONE', *, *, #24826, .T. ) ;
#27152=CARTESIAN_POINT ( 'NONE',  ( -7.167604382870000457, -77.42435704553099640, 9.599037027053000770 ) ) ;
#27155=CARTESIAN_POINT ( 'NONE',  ( 11.49150497439000063, -78.80483761240600415, -3.221926464390000078 ) ) ;
#27160=CARTESIAN_POINT ( 'NONE',  ( -6.220196401501000061, -79.03619441778099031, -9.111031286755999048 ) ) ;
#27166=CARTESIAN_POINT ( 'NONE',  ( -5.413904038987206846, -77.41666666666665719, 9.393203674808249914 ) ) ;
#27169=CARTESIAN_POINT ( 'NONE',  ( -1.061497411238000010, -76.49164580791499191, -12.45902078201000052 ) ) ;
#27171=CARTESIAN_POINT ( 'NONE',  ( 10.53044221640268674, -76.76847933843360750, 2.496041332906649757 ) ) ;
#27173=CARTESIAN_POINT ( 'NONE',  ( -10.27879708628000088, -78.67724904577400480, 4.312879667924000238 ) ) ;
#27183=CARTESIAN_POINT ( 'NONE',  ( 8.596418555780418913, -79.30208333333332860, 6.606377239730356621 ) ) ;
#27185=CARTESIAN_POINT ( 'NONE',  ( 9.596002108778145967, -77.10208333333332575, 7.374560639699001996 ) ) ;
#27190=EDGE_LOOP ( 'NONE', ( #10401, #17613, #45651, #58060 ) ) ;
#27191=CARTESIAN_POINT ( 'NONE',  ( -10.99972769911000015, -76.23554795518754190, 2.019869862886000345 ) ) ;
#27195=CARTESIAN_POINT ( 'NONE',  ( -10.37098203719999923, -77.66882059614400191, -3.760912916518000415 ) ) ;
#27201=CARTESIAN_POINT ( 'NONE',  ( 7.808618912244999599, -78.95238198094399706, -8.052551227705000869 ) ) ;
#27202=CARTESIAN_POINT ( 'NONE',  ( 0.1719510004633373057, -81.00000000000000000, 10.80697498056500727 ) ) ;
#27208=CARTESIAN_POINT ( 'NONE',  ( 11.00000000000000000, -76.04999999999999716, -1.235097113410999977E-09 ) ) ;
#27219=ORIENTED_EDGE ( 'NONE', *, *, #6279, .F. ) ;
#27221=CARTESIAN_POINT ( 'NONE',  ( 4.777753054944000155, -79.09783651582300479, -11.35249243745999870 ) ) ;
#27222=CARTESIAN_POINT ( 'NONE',  ( -11.23528222893999917, -76.07829378204800719, -0.6904789760584999492 ) ) ;
#27223=CARTESIAN_POINT ( 'NONE',  ( -4.891664181267372236, -78.01261750250401406, 9.574615555345795670 ) ) ;
#27224=CARTESIAN_POINT ( 'NONE',  ( -7.167604382869000368, -77.62772270536000008, 9.599037027053000770 ) ) ;
#27227=CARTESIAN_POINT ( 'NONE',  ( -10.40634239505360092, -79.07933785801452586, 2.787274298367601766 ) ) ;
#27229=CARTESIAN_POINT ( 'NONE',  ( 1.614104026830686323, -80.96338606111143577, 10.62792533169992737 ) ) ;
#27231=CARTESIAN_POINT ( 'NONE',  ( 12.00000000000000000, -79.54999999999999716, 0.000000000000000000 ) ) ;
#27232=CARTESIAN_POINT ( 'NONE',  ( -7.755223252044999960, -78.32736574117099337, 8.006941543446998821 ) ) ;
#27234=CARTESIAN_POINT ( 'NONE',  ( 7.447355024223999642, -80.57439977265350706, -8.285777444469999864 ) ) ;
#27240=CARTESIAN_POINT ( 'NONE',  ( 3.895497176768000003, -77.04509272339099368, 10.51870773133999926 ) ) ;
#27244=CARTESIAN_POINT ( 'NONE',  ( 1.418935787216653033, -78.63551514851324953, -10.68838327614559347 ) ) ;
#27248=CARTESIAN_POINT ( 'NONE',  ( 5.209924070321410916, -77.41110552564472869, -10.71737987758433697 ) ) ;
#27250=CARTESIAN_POINT ( 'NONE',  ( 0.5439554104848000060, -76.83774834149699018, -11.13367472273999859 ) ) ;
#27257=CARTESIAN_POINT ( 'NONE',  ( -6.446809110249994923, -80.17411999622585483, -8.621120003473629723 ) ) ;
#27266=CARTESIAN_POINT ( 'NONE',  ( -10.38493632045999959, -78.79179491694800674, 4.357414620914999759 ) ) ;
#27295=CARTESIAN_POINT ( 'NONE',  ( -4.721011358650000211, -76.36916596888400477, 9.934480763307000473 ) ) ;
#27299=CARTESIAN_POINT ( 'NONE',  ( -2.612980907336999614, -80.30468973093108787, -10.95817168551000087 ) ) ;
#27309=CARTESIAN_POINT ( 'NONE',  ( 1.618170588614999961, -80.53815307676340751, -11.14857479085000058 ) ) ;
#27313=CARTESIAN_POINT ( 'NONE',  ( -10.47020627418439354, -80.02083333333330017, -2.813789756862258518 ) ) ;
#27319=CARTESIAN_POINT ( 'NONE',  ( -9.211339595762906285, -79.55700502563119869, 5.542666473294825202 ) ) ;
#27333=CARTESIAN_POINT ( 'NONE',  ( -3.167063118518172793, -77.20133984698613006, -10.27319447007710806 ) ) ;
#27340=ORIENTED_EDGE ( 'NONE', *, *, #24433, .T. ) ;
#27341=CARTESIAN_POINT ( 'NONE',  ( -9.747171129529000666, -78.24115059798600669, -7.084379058567000342 ) ) ;
#27358=CARTESIAN_POINT ( 'NONE',  ( 10.75000000000000000, -78.25000000000000000, 1.005550720961999908E-14 ) ) ;
#27361=CARTESIAN_POINT ( 'NONE',  ( -9.964549960865001665, -77.60316956756497575, 6.650098383618001208 ) ) ;
#27391=CARTESIAN_POINT ( 'NONE',  ( -11.54988438476000034, -79.60336391412299406, 2.972544889149000280 ) ) ;
#27392=CARTESIAN_POINT ( 'NONE',  ( 7.777826874032999882, -80.26050465022970570, -7.857352429981999009 ) ) ;
#27395=CARTESIAN_POINT ( 'NONE',  ( -6.884807209879999057, -78.47409381830098596, -8.855368954042999619 ) ) ;
#27413=ORIENTED_EDGE ( 'NONE', *, *, #6993, .T. ) ;
#27418=VERTEX_POINT ( 'NONE', #4679 ) ;
#27419=CARTESIAN_POINT ( 'NONE',  ( -4.913725554697999875, -76.59869191910898678, 11.33327627240999824 ) ) ;
#27450=CARTESIAN_POINT ( 'NONE',  ( 0.4826013546558999279, -77.44837184121800533, 11.92487309688999986 ) ) ;
#27454=CARTESIAN_POINT ( 'NONE',  ( 2.143349548760000278, -78.81830367376599611, 10.82163513946999878 ) ) ;
#27458=CARTESIAN_POINT ( 'NONE',  ( 5.929749634243999701, -79.92525345888189747, -10.35361343416000146 ) ) ;
#27463=CARTESIAN_POINT ( 'NONE',  ( 9.503324371801999959, -76.56711128452499793, -8.126549174466999759 ) ) ;
#27469=CARTESIAN_POINT ( 'NONE',  ( 4.801746450173999925, -79.61653908624499820, 10.18710928510000002 ) ) ;
#27471=CARTESIAN_POINT ( 'NONE',  ( 8.596418555780418913, -79.80208333333331439, 6.606377239730356621 ) ) ;
#27478=CARTESIAN_POINT ( 'NONE',  ( 10.74999999999999645, -78.26041666666667140, 1.407171709420451666 ) ) ;
#27483=CARTESIAN_POINT ( 'NONE',  ( 9.933944441255952995, -78.81885939776891803, -4.108317294789329388 ) ) ;
#27487=CARTESIAN_POINT ( 'NONE',  ( 8.899186938125001944, -76.04999999999999716, 6.465637775217000005 ) ) ;
#27489=CARTESIAN_POINT ( 'NONE',  ( -8.494907789873000326, -76.52071859265899434, 6.628721719457000283 ) ) ;
#27491=CARTESIAN_POINT ( 'NONE',  ( -11.74999252561975993, -76.05421570306441481, -0.7144598671462676354 ) ) ;
#27492=CARTESIAN_POINT ( 'NONE',  ( -5.261570549498088667, -77.63871931694440320, -10.76270721987074985 ) ) ;
#27493=CARTESIAN_POINT ( 'NONE',  ( -11.04065564778000130, -79.25198175396400302, 1.980412446595999798 ) ) ;
#27494=CARTESIAN_POINT ( 'NONE',  ( 7.219057816503211100, -81.00000000000001421, 8.170402670078926732 ) ) ;
#27502=DIRECTION ( 'NONE',  ( -1.000000000000000000, 0.000000000000000000, 0.000000000000000000 ) ) ;
#27513=CARTESIAN_POINT ( 'NONE',  ( 1.505038102365999997, -79.30638830090799729, 12.22460098059000089 ) ) ;
#27514=CARTESIAN_POINT ( 'NONE',  ( -4.507826919401000332, -76.16562155000400480, -10.31444853584999954 ) ) ;
#27515=CARTESIAN_POINT ( 'NONE',  ( -6.954863410765665499, -78.03105792949766339, 8.197110803945740543 ) ) ;
#27516=CARTESIAN_POINT ( 'NONE',  ( 1.634596122093999959, -78.99778786954298937, 11.63574645295999943 ) ) ;
#27519=CARTESIAN_POINT ( 'NONE',  ( -10.75000000000000000, -79.50000000000000000, 0.000000000000000000 ) ) ;
#27521=CARTESIAN_POINT ( 'NONE',  ( 7.971085775996931133, -80.90878701328509237, 7.212855077932124104 ) ) ;
#27524=CARTESIAN_POINT ( 'NONE',  ( 3.947457275559000500, -78.61298354959900792, -10.30140706531999939 ) ) ;
#27526=CARTESIAN_POINT ( 'NONE',  ( 0.5321997431402999412, -80.76233357467889107, 11.12807117834999993 ) ) ;
#27531=CARTESIAN_POINT ( 'NONE',  ( -9.524774638983998898, -77.15403809539800761, 5.924253427062000199 ) ) ;
#27533=CARTESIAN_POINT ( 'NONE',  ( 10.75000000000000000, -76.85000000000000853, 0.000000000000000000 ) ) ;
#27535=CARTESIAN_POINT ( 'NONE',  ( -3.518896154528292186, -78.59855647164599191, -10.19177539389869658 ) ) ;
#27542=CARTESIAN_POINT ( 'NONE',  ( -9.340344124447998553, -76.82376637690499876, -6.292213870087999261 ) ) ;
#27555=CARTESIAN_POINT ( 'NONE',  ( -6.167563198928999846, -79.81279398642419665, 9.285244464097999639 ) ) ;
#27557=VERTEX_POINT ( 'NONE', #52106 ) ;
#27573=ORIENTED_EDGE ( 'NONE', *, *, #22764, .T. ) ;
#27587=CARTESIAN_POINT ( 'NONE',  ( 10.78853149093999875, -80.49286902822179002, -3.242959171380999983 ) ) ;
#27595=CARTESIAN_POINT ( 'NONE',  ( 8.440675369999999234, -80.20707853072349280, 7.053722371789000967 ) ) ;
#27606=CARTESIAN_POINT ( 'NONE',  ( -4.854729178351636421, -79.51242566855798088, 9.591276152018627599 ) ) ;
#27608=CARTESIAN_POINT ( 'NONE',  ( -10.75000000000000000, -76.59999999999999432, 0.000000000000000000 ) ) ;
#27622=CARTESIAN_POINT ( 'NONE',  ( 1.333500915678079490, -77.23504576798873700, -10.67566761252578011 ) ) ;
#27628=CARTESIAN_POINT ( 'NONE',  ( 4.766258734843114908, -80.33859090758983257, 9.686463997712579044 ) ) ;
#27630=CARTESIAN_POINT ( 'NONE',  ( -0.08569088068254999968, -78.56670238307098941, 12.04941611642000154 ) ) ;
#27636=CARTESIAN_POINT ( 'NONE',  ( -10.41501344424586151, -76.44116683086167541, -6.014273019200089720 ) ) ;
#27641=ORIENTED_EDGE ( 'NONE', *, *, #33229, .F. ) ;
#27646=CYLINDRICAL_SURFACE ( 'NONE', #53823, 9.599999999999999645 ) ;
#27647=CARTESIAN_POINT ( 'NONE',  ( -5.279550234765999939, -76.35198175396399733, -9.859017853534000508 ) ) ;
#27651=CARTESIAN_POINT ( 'NONE',  ( -7.892176027305001007, -76.76043262182999172, 7.987326983142001069 ) ) ;
#27671=CARTESIAN_POINT ( 'NONE',  ( -5.393290222407999934, -77.46222517136899910, -11.03214393298000040 ) ) ;
#27680=CARTESIAN_POINT ( 'NONE',  ( 11.83689625619999930, -79.36366123649499116, -1.457305633747999929 ) ) ;
#27681=CARTESIAN_POINT ( 'NONE',  ( -10.32512362061000033, -80.67574026708460622, 4.564420309708999923 ) ) ;
#27687=CARTESIAN_POINT ( 'NONE',  ( 11.55824937009300868, -79.80000000000001137, -2.451020469013467817 ) ) ;
#27688=CLOSED_SHELL ( 'NONE', ( #8698, #37315, #12420, #1371, #56624, #26073, #26346, #3095, #28658, #9343, #28734, #34152, #13633, #44629, #35839, #5604, #56697, #23541, #52166, #23218, #35341, #48609, #31185, #52956, #28115, #11544, #35324, #7646, #26828, #16092, #57761, #1985, #22767, #43642, #7940, #55312, #32074, #26223, #6255, #20341, #51716, #29414, #36185, #50176, #34872, #33638, #13136, #29595, #4304, #16642, #21961, #47442, #49177, #14901, #45622, #80, #33876, #33, #29702, #32044, #13191, #16840, #18319, #41242, #1737, #30386, #24500, #7287, #40922, #46863, #54351, #1702, #55017, #47661, #9322, #34053, #25020, #34024, #9826, #29705, #41772, #27898, #19190, #42132, #45687, #37233, #30863, #51647, #44420, #47724, #58280, #49434, #29394, #39554, #41948, #15439, #3977, #7106, #42183, #33909, #13804, #34759, #58223, #335, #12739, #12705 ) ) ;
#27689=CARTESIAN_POINT ( 'NONE',  ( -10.70506908183094197, -76.16458333332448660, 2.279133419649182368 ) ) ;
#27706=AXIS2_PLACEMENT_3D ( 'NONE', #3475, #21480, #26194 ) ;
#27716=CARTESIAN_POINT ( 'NONE',  ( 11.68767212001979594, -79.02916666666666856, -3.140974612311341563 ) ) ;
#27728=CARTESIAN_POINT ( 'NONE',  ( 11.61133755414000035, -76.97808292597399316, 3.999933378912999604 ) ) ;
#27733=CARTESIAN_POINT ( 'NONE',  ( 10.49311453041000064, -79.97125767581903233, -3.963918880051000126 ) ) ;
#27735=DIRECTION ( 'NONE',  ( 0.000000000000000000, 1.000000000000000000, 0.000000000000000000 ) ) ;
#27740=CARTESIAN_POINT ( 'NONE',  ( 9.505630310840999186, -77.70619656188999613, -7.405319984134000499 ) ) ;
#27743=CARTESIAN_POINT ( 'NONE',  ( -5.182070223403000497, -78.87277635977000045, 9.738987759633999985 ) ) ;
#27751=EDGE_CURVE ( 'NONE', #38434, #13166, #26758, .T. ) ;
#27754=CARTESIAN_POINT ( 'NONE',  ( 12.42265170273000052, -76.11431842486598498, -1.425377385046999956 ) ) ;
#27760=CARTESIAN_POINT ( 'NONE',  ( -0.2704138798119000153, -79.08579419080099626, 11.14367429999999892 ) ) ;
#27762=CARTESIAN_POINT ( 'NONE',  ( -11.66814978394733338, -79.56040689563938884, -1.554668868100800738 ) ) ;
#27777=CARTESIAN_POINT ( 'NONE',  ( 7.708894260666084186, -78.78865531770708230, -7.492582358052589875 ) ) ;
#27782=CARTESIAN_POINT ( 'NONE',  ( 4.543288497605388443, -76.89401257029606995, 11.32213107881294789 ) ) ;
#27783=CARTESIAN_POINT ( 'NONE',  ( 4.458804082352973097, -77.39455547813037128, 11.11931012016017917 ) ) ;
#27784=CARTESIAN_POINT ( 'NONE',  ( 10.58946819037999987, -78.48936414991298705, -3.698823201301000285 ) ) ;
#27785=CARTESIAN_POINT ( 'NONE',  ( 2.475061660928486784, -81.00000000000001421, 10.54437239986970809 ) ) ;
#27795=CARTESIAN_POINT ( 'NONE',  ( 1.570796326794910547, -77.53541666666666288, -11.99999999999999822 ) ) ;
#27796=CARTESIAN_POINT ( 'NONE',  ( -7.374560639698973574, -78.47291666666666288, -9.596002108778167283 ) ) ;
#27804=CARTESIAN_POINT ( 'NONE',  ( -11.90098819343999992, -79.02652905684600171, -2.686189377354999852 ) ) ;
#27805=CARTESIAN_POINT ( 'NONE',  ( -10.47968562137999982, -76.74722307105399466, 4.029083465249000184 ) ) ;
#27806=CARTESIAN_POINT ( 'NONE',  ( 10.45204020799386946, -77.86881889335130325, 2.513295852507721584 ) ) ;
#27807=CARTESIAN_POINT ( 'NONE',  ( -10.61596739836999959, -78.67223608445800664, -5.551333230057999835 ) ) ;
#27814=CARTESIAN_POINT ( 'NONE',  ( 5.230327773973000305, -78.05500231115298959, -9.843691987646998598 ) ) ;
#27815=CARTESIAN_POINT ( 'NONE',  ( -4.885220488697999741, -76.55755186839822102, 11.26753068192000029 ) ) ;
#27816=CARTESIAN_POINT ( 'NONE',  ( -10.23652643648999927, -80.92341969070069752, -4.396672205467000438 ) ) ;
#27817=ORIENTED_EDGE ( 'NONE', *, *, #18492, .F. ) ;
#27822=CARTESIAN_POINT ( 'NONE',  ( -10.96060824219999930, -77.18127443839999557, 2.383941600041999731 ) ) ;
#27840=CARTESIAN_POINT ( 'NONE',  ( -9.719853332338134422, -80.13579794343719698, -4.669139681347004078 ) ) ;
#27845=CARTESIAN_POINT ( 'NONE',  ( 1.081678475801000072, -79.82604836483349686, 10.97869327635999781 ) ) ;
#27856=CARTESIAN_POINT ( 'NONE',  ( 9.596002108778172612, -76.49791666665605305, -7.374560639698962028 ) ) ;
#27859=ORIENTED_EDGE ( 'NONE', *, *, #44633, .F. ) ;
#27861=LINE ( 'NONE', #472, #21577 ) ;
#27872=AXIS2_PLACEMENT_3D ( 'NONE', #55275, #42294, #32527 ) ;
#27876=CARTESIAN_POINT ( 'NONE',  ( -4.454457568640999732, -80.67345514424359010, 10.34731867136000005 ) ) ;
#27893=CARTESIAN_POINT ( 'NONE',  ( 5.512944058422025506, -79.43216301949462377, 9.240081554467723279 ) ) ;
#27898=ADVANCED_FACE ( 'NONE', ( #2446 ), #35125, .F. ) ;
#27902=EDGE_CURVE ( 'NONE', #28197, #7888, #14760, .T. ) ;
#27908=DIRECTION ( 'NONE',  ( 0.000000000000000000, -1.000000000000000000, -2.483745111066999960E-13 ) ) ;
#27911=CARTESIAN_POINT ( 'NONE',  ( 3.714552462503000196, -79.55170192472400004, 11.44155784250999908 ) ) ;
#27912=CARTESIAN_POINT ( 'NONE',  ( -3.093366010725773219, -76.11510416600961548, -11.50726245973735473 ) ) ;
#27920=EDGE_CURVE ( 'NONE', #22076, #12674, #40907, .T. ) ;
#27924=DIRECTION ( 'NONE',  ( 0.000000000000000000, 0.000000000000000000, -1.000000000000000000 ) ) ;
#27935=CARTESIAN_POINT ( 'NONE',  ( -9.939389728518001732, -76.72821088380000276, 5.126617716248000001 ) ) ;
#27938=CARTESIAN_POINT ( 'NONE',  ( -8.108261698375999416, -76.38420349199300574, -7.767871074888999416 ) ) ;
#27947=CARTESIAN_POINT ( 'NONE',  ( -2.810647185591240049, -76.29609374999736815, 11.70020478678804565 ) ) ;
#27948=CARTESIAN_POINT ( 'NONE',  ( 2.813789756862274505, -79.64583333333330017, -10.47020627418438821 ) ) ;
#27951=CARTESIAN_POINT ( 'NONE',  ( -12.00000000000000000, -79.39999999999999147, 0.000000000000000000 ) ) ;
#27968=CARTESIAN_POINT ( 'NONE',  ( 6.901085230909000501, -80.95330344751930340, -9.080895641036999422 ) ) ;
#27972=CARTESIAN_POINT ( 'NONE',  ( 11.01642476345000077, -77.16674935421400505, 2.111041454437999842 ) ) ;
#27978=CARTESIAN_POINT ( 'NONE',  ( 8.225372035788822700, -81.00000000000000000, -7.395153854250120062 ) ) ;
#27987=ORIENTED_EDGE ( 'NONE', *, *, #48162, .T. ) ;
#27988=CARTESIAN_POINT ( 'NONE',  ( 4.023394881099000564, -78.67502719647299614, 11.60207191892000012 ) ) ;
#27998=CARTESIAN_POINT ( 'NONE',  ( 3.535142739574999915, -79.92176962903970150, 10.17871189313000002 ) ) ;
#28020=CARTESIAN_POINT ( 'NONE',  ( -11.94395460750000204, -77.04741951094599983, 2.857367593729999822 ) ) ;
#28025=CARTESIAN_POINT ( 'NONE',  ( -11.19989528650999944, -78.74562224073753214, 0.6168112860373000661 ) ) ;
#28028=CARTESIAN_POINT ( 'NONE',  ( 0.000000000000000000, -76.14999999999999147, 0.000000000000000000 ) ) ;
#28034=CARTESIAN_POINT ( 'NONE',  ( -7.660291894363999710, -78.43868807833099766, 9.301381605274000819 ) ) ;
#28037=CARTESIAN_POINT ( 'NONE',  ( 5.650974246042000715, -78.79106733076498870, 9.474609463724998903 ) ) ;
#28044=CARTESIAN_POINT ( 'NONE',  ( 11.70294133920999968, -76.15205116317100931, 4.403991283866000472 ) ) ;
#28050=CARTESIAN_POINT ( 'NONE',  ( -8.235122208958999934, -78.65001270277200263, 7.512480467459000444 ) ) ;
#28052=CARTESIAN_POINT ( 'NONE',  ( 1.407171709420391936, -79.86458333333330017, 10.75000000000000178 ) ) ;
#28067=CARTESIAN_POINT ( 'NONE',  ( 9.298325636522646320, -78.80826077773562588, -5.396105918537423385 ) ) ;
#28073=CARTESIAN_POINT ( 'NONE',  ( -11.51862140649527433, -76.07163159476074554, -3.285871775498967473 ) ) ;
#28075=CARTESIAN_POINT ( 'NONE',  ( 8.273086841016404236, -78.23556425626672706, -8.664642258571072730 ) ) ;
#28076=CARTESIAN_POINT ( 'NONE',  ( 10.12058791103999944, -79.55158152698399476, 4.836508133599999759 ) ) ;
#28091=EDGE_CURVE ( 'NONE', #15092, #42165, #38654, .T. ) ;
#28095=CARTESIAN_POINT ( 'NONE',  ( -5.688772062455999645, -78.96059218971498694, -11.05567345541000002 ) ) ;
#28096=CARTESIAN_POINT ( 'NONE',  ( 9.797622870535001027, -75.99542849098199326, 4.847984067100000516 ) ) ;
#28097=CARTESIAN_POINT ( 'NONE',  ( 4.872804577377794821, -77.93772164444546036, 9.582789123844438706 ) ) ;
#28098=CARTESIAN_POINT ( 'NONE',  ( 11.20799393363000007, -77.91261525259299958, 4.230477091134000389 ) ) ;
#28102=CARTESIAN_POINT ( 'NONE',  ( 10.75000000000000000, -76.75000000000000000, 0.000000000000000000 ) ) ;
#28105=CARTESIAN_POINT ( 'NONE',  ( -2.172168385828000314, -78.00052962514999422, -10.93326506925000174 ) ) ;
#28106=CARTESIAN_POINT ( 'NONE',  ( 5.459501886381000091, -76.31165543856863565, -11.00074850082999767 ) ) ;
#28107=CARTESIAN_POINT ( 'NONE',  ( 5.392198052114999918, -81.12538518513179042, -9.378990218028999237 ) ) ;
#28111=CARTESIAN_POINT ( 'NONE',  ( 9.144378690012999300, -77.39916518241399501, -6.496033325431000094 ) ) ;
#28115=ADVANCED_FACE ( 'NONE', ( #52245 ), #51386, .F. ) ;
#28122=CARTESIAN_POINT ( 'NONE',  ( 11.06080859785000037, -77.04165712091899820, 2.119546583493000291 ) ) ;
#28125=DIRECTION ( 'NONE',  ( 1.000000000000000000, 0.000000000000000000, 0.000000000000000000 ) ) ;
#28134=CARTESIAN_POINT ( 'NONE',  ( 6.654794014482000364, -79.63539396382098801, -8.798605060253001042 ) ) ;
#28148=CARTESIAN_POINT ( 'NONE',  ( 10.47020627418439531, -78.22916666666665719, -2.813789756862242974 ) ) ;
#28150=EDGE_CURVE ( 'NONE', #25175, #7399, #41168, .T. ) ;
#28153=CARTESIAN_POINT ( 'NONE',  ( 1.387435826181646847, -77.03417277704993182, -11.96237581351085488 ) ) ;
#28166=CARTESIAN_POINT ( 'NONE',  ( 1.328862289696999932, -80.13169679617828933, 11.18676134159000135 ) ) ;
#28168=CARTESIAN_POINT ( 'NONE',  ( 12.00000000000000000, -77.16041666666669130, 1.570796326794922093 ) ) ;
#28170=CARTESIAN_POINT ( 'NONE',  ( 5.137083998358000336, -77.21100733245999947, -10.56753840748999984 ) ) ;
#28179=DIRECTION ( 'NONE',  ( 1.000000000000000000, 0.000000000000000000, -1.156375342703997101E-13 ) ) ;
#28182=CARTESIAN_POINT ( 'NONE',  ( 8.488409410023923130, -79.40273845399939034, 6.622596058701640587 ) ) ;
#28197=VERTEX_POINT ( 'NONE', #35068 ) ;
#28198=CARTESIAN_POINT ( 'NONE',  ( -12.02912753549999891, -79.63333152568600326, 0.08506824670321999626 ) ) ;
#28199=DIRECTION ( 'NONE',  ( 1.000000000000000000, 0.000000000000000000, 0.000000000000000000 ) ) ;
#28203=CARTESIAN_POINT ( 'NONE',  ( 1.714448272638999793, -77.26006991430598703, -11.65560625356000024 ) ) ;
#28216=CARTESIAN_POINT ( 'NONE',  ( -1.407171709420418138, -80.61458333333331439, -10.75000000000000000 ) ) ;
#28223=CARTESIAN_POINT ( 'NONE',  ( -1.432420283025999996, -76.15132621805099689, 11.09153081809999897 ) ) ;
#28233=EDGE_CURVE ( 'NONE', #41078, #43698, #49864, .T. ) ;
#28240=CARTESIAN_POINT ( 'NONE',  ( -3.140974612311405512, -79.29583333333334849, 11.68767212001977640 ) ) ;
#28256=CARTESIAN_POINT ( 'NONE',  ( -10.71935382865999919, -80.11839559862080762, 3.149475271190000036 ) ) ;
#28259=CARTESIAN_POINT ( 'NONE',  ( -11.16975252231999960, -76.89438592419598706, 1.027088271520000040 ) ) ;
#28265=CARTESIAN_POINT ( 'NONE',  ( 7.390111938209032338, -76.06041666666433798, 8.214641434548898502 ) ) ;
#28270=CARTESIAN_POINT ( 'NONE',  ( 6.985849709488999970, -80.87654576500008829, -8.837815942395002011 ) ) ;
#28272=VERTEX_POINT ( 'NONE', #4974 ) ;
#28278=CARTESIAN_POINT ( 'NONE',  ( 0.4965625967630000193, -77.69837184121800533, 12.26984941905000071 ) ) ;
#28289=VECTOR ( 'NONE', #36817, 1000.000000000000000 ) ;
#28306=CARTESIAN_POINT ( 'NONE',  ( 5.459501886381000091, -76.29555329812299647, -11.00074850082999767 ) ) ;
#28307=LINE ( 'NONE', #41613, #2540 ) ;
#28312=FACE_OUTER_BOUND ( 'NONE', #43920, .T. ) ;
#28317=CARTESIAN_POINT ( 'NONE',  ( -0.08569088068253999380, -78.38442944748399555, 12.04941611642000154 ) ) ;
#28321=CARTESIAN_POINT ( 'NONE',  ( -3.912255148455999976, -79.43075759821599036, 10.19164489391000217 ) ) ;
#28326=CARTESIAN_POINT ( 'NONE',  ( -5.655986146074000409, -79.84535256633930089, -10.76033745225999994 ) ) ;
#28329=B_SPLINE_CURVE_WITH_KNOTS ( 'NONE', 3,
 ( #30132, #7714, #25715, #43741, #3294, #21286, #51739, #17147, #12996, #35134 ),
 .UNSPECIFIED., .F., .F.,
 ( 4, 2, 2, 2, 4 ),
 ( 0.000000000000000000, 0.07142685916348760766, 0.1428537183269752153, 0.2142805774904628369, 0.2857074366539503751 ),
 .UNSPECIFIED. ) ;
#28332=CARTESIAN_POINT ( 'NONE',  ( 3.140974612311326908, -77.75416666666663446, 11.68767212001979772 ) ) ;
#28336=ORIENTED_EDGE ( 'NONE', *, *, #58364, .F. ) ;
#28338=CARTESIAN_POINT ( 'NONE',  ( -11.12012002604264893, -79.52207733847474458, 4.052612807419244234 ) ) ;
#28345=CARTESIAN_POINT ( 'NONE',  ( 3.507204654865230697, -79.19960255973779795, 10.65462925082876922 ) ) ;
#28351=CARTESIAN_POINT ( 'NONE',  ( 10.65280642239534181, -76.21655266097438641, 2.270707054235461264 ) ) ;
#28359=CARTESIAN_POINT ( 'NONE',  ( 7.031078451151031139, -78.78178807021924968, -8.132049469059730029 ) ) ;
#28364=CARTESIAN_POINT ( 'NONE',  ( 11.86917441439930521, -76.78081435538106803, -2.820429242449539853 ) ) ;
#28366=CARTESIAN_POINT ( 'NONE',  ( 0.9627606596332135558, -78.18130562541935547, -11.94123457856478510 ) ) ;
#28367=CARTESIAN_POINT ( 'NONE',  ( -4.019809786096000259, -79.17027272495799650, 10.47183077952999852 ) ) ;
#28386=CARTESIAN_POINT ( 'NONE',  ( 9.218059003579000432, -79.06486808225800189, -8.343706100361000466 ) ) ;
#28389=CARTESIAN_POINT ( 'NONE',  ( 9.954879088412631916, -77.88099781617175665, 4.068718871676561655 ) ) ;
#28390=CARTESIAN_POINT ( 'NONE',  ( 10.69384760718000038, -78.27889574609699253, -5.399785902169999652 ) ) ;
#28395=CARTESIAN_POINT ( 'NONE',  ( 9.474936504858838759, -80.88936561845106610, 5.078570178447623817 ) ) ;
#28399=CARTESIAN_POINT ( 'NONE',  ( 6.035973157159999936, -78.69886817601300777, -8.925829823522999362 ) ) ;
#28400=CARTESIAN_POINT ( 'NONE',  ( -11.94395460750000204, -77.13131020466720145, 2.857367593729999822 ) ) ;
#28401=CARTESIAN_POINT ( 'NONE',  ( -3.148499409464999843, -80.85690832509547477, 10.56665097621000093 ) ) ;
#28403=CARTESIAN_POINT ( 'NONE',  ( 6.233047529871999615, -78.88050366622999832, 9.960502923565000444 ) ) ;
#28404=CARTESIAN_POINT ( 'NONE',  ( -10.46965315338386482, -80.57920048190398177, 2.813976240919467298 ) ) ;
#28405=CARTESIAN_POINT ( 'NONE',  ( 6.201912463541000342, -78.50617185603199744, -9.171216270948999494 ) ) ;
#28416=CARTESIAN_POINT ( 'NONE',  ( 9.181220278661999856, -77.47743860894799184, -6.522205052974000772 ) ) ;
#28418=CARTESIAN_POINT ( 'NONE',  ( -12.00000000000000000, -76.79999999999999716, 1.164316068523999942E-14 ) ) ;
#28430=CARTESIAN_POINT ( 'NONE',  ( 10.71899861749000138, -79.68986664982399759, -2.608601736514999825 ) ) ;
#28432=EDGE_LOOP ( 'NONE', ( #47782, #37728, #23909 ) ) ;
#28435=VERTEX_POINT ( 'NONE', #20055 ) ;
#28443=CARTESIAN_POINT ( 'NONE',  ( 12.00000000000000000, -76.54999999999999716, 0.000000000000000000 ) ) ;
#28449=CARTESIAN_POINT ( 'NONE',  ( -10.00716890277074356, -76.94696047196750044, -6.699252482692386934 ) ) ;
#28452=CARTESIAN_POINT ( 'NONE',  ( -5.051502324002999760E-14, -80.79999999999999716, 0.000000000000000000 ) ) ;
#28456=CARTESIAN_POINT ( 'NONE',  ( -11.87139580924456439, -77.31341727770499972, -2.023209039049734148 ) ) ;
#28463=CARTESIAN_POINT ( 'NONE',  ( -10.47023603244697121, -76.62094508224406297, -2.813753789789203541 ) ) ;
#28479=CARTESIAN_POINT ( 'NONE',  ( 10.75000000000000000, -79.35000000000000853, 0.000000000000000000 ) ) ;
#28489=LINE ( 'NONE', #15213, #37676 ) ;
#28493=CARTESIAN_POINT ( 'NONE',  ( -6.217716982067981846, -77.17607982036621195, -8.769278404477413247 ) ) ;
#28498=CARTESIAN_POINT ( 'NONE',  ( -0.7406579117306999471, -79.51379700229598768, 12.00660533699000077 ) ) ;
#28499=DIRECTION ( 'NONE',  ( -1.000000000000000000, 0.000000000000000000, 0.000000000000000000 ) ) ;
#28503=CARTESIAN_POINT ( 'NONE',  ( -11.81636186152999990, -78.63462189577700201, -1.676035442350999993 ) ) ;
#28506=CARTESIAN_POINT ( 'NONE',  ( 5.413904038987143785, -78.83333333333330017, 9.393203674808290771 ) ) ;
#28518=CARTESIAN_POINT ( 'NONE',  ( 1.035792215605076949, -79.80000000000001137, -11.73450628681306718 ) ) ;
#28519=CARTESIAN_POINT ( 'NONE',  ( -10.62888400727746863, -80.08839518812462188, 1.609190229725424803 ) ) ;
#28522=CARTESIAN_POINT ( 'NONE',  ( -5.007180289739999068, -76.61025844654599837, 10.00009952528999868 ) ) ;
#28523=CARTESIAN_POINT ( 'NONE',  ( 7.550822941564469204, -76.41427617356011126, 7.692254321527583372 ) ) ;
#28525=CARTESIAN_POINT ( 'NONE',  ( -10.90146613631999983, -76.81059650580800735, 1.770589923316999936 ) ) ;
#28535=CARTESIAN_POINT ( 'NONE',  ( 8.474185241649847100, -76.24531250000731575, 8.471026285512541776 ) ) ;
#28540=CARTESIAN_POINT ( 'NONE',  ( 1.570796326794856590, -79.26458333333330586, 12.00000000000000711 ) ) ;
#28549=CARTESIAN_POINT ( 'NONE',  ( 0.4965625967630000193, -77.24519064797900114, 12.26984941905000071 ) ) ;
#28554=CARTESIAN_POINT ( 'NONE',  ( -7.478374335766999614, -80.70849464549387164, 8.611710654069998583 ) ) ;
#28558=CARTESIAN_POINT ( 'NONE',  ( -6.659967121051000305, -76.97609495320099882, -9.025682433062998555 ) ) ;
#28564=CARTESIAN_POINT ( 'NONE',  ( -10.87500000000999911, -76.17499999999400018, 1.221063213659000093E-09 ) ) ;
#28567=CARTESIAN_POINT ( 'NONE',  ( 10.24999999991999999, -82.10000000007899246, -6.817370023903000320E-10 ) ) ;
#28575=CARTESIAN_POINT ( 'NONE',  ( 7.024610939158000278, -78.93285191714500115, -9.931634882699999167 ) ) ;
#28583=CARTESIAN_POINT ( 'NONE',  ( -9.392812284823671476, -77.64167586065022419, -5.413627597448644302 ) ) ;
#28603=CARTESIAN_POINT ( 'NONE',  ( -11.38972971424999869, -76.66439794286800691, -4.593112662244999811 ) ) ;
#28608=CARTESIAN_POINT ( 'NONE',  ( -1.639962962630000076, -78.63667686873010609, 11.09633417262999977 ) ) ;
#28617=CARTESIAN_POINT ( 'NONE',  ( -1.845833107322000011, -77.89610176985598855, 11.90750485256000069 ) ) ;
#28625=CARTESIAN_POINT ( 'NONE',  ( -11.77263653225999995, -79.73881804294899212, 3.029873667130000392 ) ) ;
#28635=CARTESIAN_POINT ( 'NONE',  ( 5.768896245881999896, -78.60879439517700007, 9.672321370914000127 ) ) ;
#28636=CARTESIAN_POINT ( 'NONE',  ( -7.695151247652856519, -76.28527187395242493, 8.115589632975689582 ) ) ;
#28642=CARTESIAN_POINT ( 'NONE',  ( 10.93175546140675003, -79.11789353073278619, 2.513629148400740032 ) ) ;
#28647=CARTESIAN_POINT ( 'NONE',  ( 12.00000000000000000, -78.54999999999999716, 0.000000000000000000 ) ) ;
#28650=CARTESIAN_POINT ( 'NONE',  ( -9.596002108778193929, -77.24791666666666856, 7.374560639698935383 ) ) ;
#28654=CARTESIAN_POINT ( 'NONE',  ( 7.210467705727123366, -78.78352963214712190, -7.974047016889574735 ) ) ;
#28658=ADVANCED_FACE ( 'NONE', ( #53067 ), #35492, .T. ) ;
#28662=CARTESIAN_POINT ( 'NONE',  ( 4.628805853411431137, -76.70534887877106200, -11.28743898164479553 ) ) ;
#28663=CARTESIAN_POINT ( 'NONE',  ( -10.61611263540728700, -78.58824535677541689, -5.551409177842876019 ) ) ;
#28664=CARTESIAN_POINT ( 'NONE',  ( -2.710423231297999891, -79.72831545226699745, 10.88447134676999895 ) ) ;
#28669=CARTESIAN_POINT ( 'NONE',  ( 2.976905979876097952, -77.49628357046933047, -10.81478801228704079 ) ) ;
#28672=CARTESIAN_POINT ( 'NONE',  ( 7.374560639698994002, -78.57708333333330586, -9.596002108778151296 ) ) ;
#28682=CARTESIAN_POINT ( 'NONE',  ( -11.59066951726000028, -76.28147497528598819, -0.7123197670545999838 ) ) ;
#28683=CARTESIAN_POINT ( 'NONE',  ( 10.47042279852835200, -77.86824023481268853, 2.435997539233151876 ) ) ;
#28684=CARTESIAN_POINT ( 'NONE',  ( 0.4844284812283000119, -77.50567552123600024, 11.97002061314999999 ) ) ;
#28692=CARTESIAN_POINT ( 'NONE',  ( -8.585712843602999911, -77.90483863155199629, 6.927284413728999724 ) ) ;
#28694=CARTESIAN_POINT ( 'NONE',  ( 4.099300690538000502, -80.87094001750114103, 10.11134612214000050 ) ) ;
#28699=CARTESIAN_POINT ( 'NONE',  ( 9.662374122931806752, -80.38663027733564093, 4.763869651305610020 ) ) ;
#28700=CARTESIAN_POINT ( 'NONE',  ( 2.976864594307000011, -77.41248104968700261, -10.81463766284999828 ) ) ;
#28704=CARTESIAN_POINT ( 'NONE',  ( 4.525754325328000149, -76.92122343098399995, 11.27843493294999888 ) ) ;
#28711=CARTESIAN_POINT ( 'NONE',  ( -3.257558841711999609, -76.87823906290799414, -10.78064358917000121 ) ) ;
#28714=CARTESIAN_POINT ( 'NONE',  ( 7.374560639698954034, -77.62291666666666856, 9.596002108778181494 ) ) ;
#28717=ORIENTED_EDGE ( 'NONE', *, *, #563, .F. ) ;
#28723=CARTESIAN_POINT ( 'NONE',  ( -8.243938165231000426, -80.01670276584620467, -7.330703780023000604 ) ) ;
#28730=VERTEX_POINT ( 'NONE', #22048 ) ;
#28733=PRODUCT_CONTEXT ( 'NONE', #40183, 'mechanical' ) ;
#28734=ADVANCED_FACE ( 'NONE', ( #35322 ), #39391, .F. ) ;
#28746=CARTESIAN_POINT ( 'NONE',  ( -8.596418555780431348, -76.55208333333331439, -6.606377239730338857 ) ) ;
#28755=CARTESIAN_POINT ( 'NONE',  ( -7.374560639699019760, -77.32708333333330586, 9.596002108778129980 ) ) ;
#28759=DIRECTION ( 'NONE',  ( 1.000000000000000000, 0.000000000000000000, 0.000000000000000000 ) ) ;
#28762=CARTESIAN_POINT ( 'NONE',  ( -11.18527010467000160, -78.31411136276199159, 1.312896411821999898 ) ) ;
#28774=CARTESIAN_POINT ( 'NONE',  ( -0.0004935696944198294904, -79.47512061975739073, 10.74992982259620078 ) ) ;
#28777=CARTESIAN_POINT ( 'NONE',  ( 0.000000000000000000, -76.00000000000000000, -11.70000000000000107 ) ) ;
#28787=CARTESIAN_POINT ( 'NONE',  ( 5.169396783903556170, -80.26528074669050739, -9.426735840945569933 ) ) ;
#28788=CARTESIAN_POINT ( 'NONE',  ( -6.587136192994185180, -77.17264154318887392, -8.498578688690102467 ) ) ;
#28792=CARTESIAN_POINT ( 'NONE',  ( 11.66950233118999947, -79.36437884805799570, -2.920592611544999606 ) ) ;
#28796=CARTESIAN_POINT ( 'NONE',  ( 4.441925970415999458, -77.46806133255499560, 11.07721969470000190 ) ) ;
#28800=ORIENTED_EDGE ( 'NONE', *, *, #12317, .T. ) ;
#28803=EDGE_LOOP ( 'NONE', ( #33592, #29549, #24508, #54457 ) ) ;
#28808=CARTESIAN_POINT ( 'NONE',  ( 1.407171709420440342, -80.63541666666665719, -10.74999999999999822 ) ) ;
#28811=CARTESIAN_POINT ( 'NONE',  ( -10.61509443659918084, -80.08771556321305241, 1.696495127445934559 ) ) ;
#28814=CARTESIAN_POINT ( 'NONE',  ( 11.01994305158000031, -76.50247340589800160, -1.906499110313000234 ) ) ;
#28817=CARTESIAN_POINT ( 'NONE',  ( 4.923701317394000299, -76.48453125995000335, -10.09162495054999908 ) ) ;
#28824=CARTESIAN_POINT ( 'NONE',  ( 8.035052034801999810, -79.89370463075219675, 9.025357223237000071 ) ) ;
#28825=CARTESIAN_POINT ( 'NONE',  ( -9.232585280256000004, -78.05730742239006759, 5.508089239726199793 ) ) ;
#28829=CARTESIAN_POINT ( 'NONE',  ( 6.232755757386176043, -78.91383699956330133, 9.960036924250847079 ) ) ;
#28835=FACE_OUTER_BOUND ( 'NONE', #7469, .T. ) ;
#28843=CARTESIAN_POINT ( 'NONE',  ( -7.401941616262999624, -80.64076758108089393, 8.523694671541999668 ) ) ;
#28845=CARTESIAN_POINT ( 'NONE',  ( 2.273403379124000026E-14, -92.33215535459000023, 0.000000000000000000 ) ) ;
#28846=CARTESIAN_POINT ( 'NONE',  ( 2.854969924326999919, -78.25620307428700073, 10.84745395576000071 ) ) ;
#28864=AXIS2_PLACEMENT_3D ( 'NONE', #46879, #17813, #3928 ) ;
#28866=CARTESIAN_POINT ( 'NONE',  ( -4.148749056195000229, -78.66155876290798687, 11.43548913925000043 ) ) ;
#28868=CARTESIAN_POINT ( 'NONE',  ( -4.763776579928164168, -77.51148305309406794, 9.662172649054632245 ) ) ;
#28871=VERTEX_POINT ( 'NONE', #10768 ) ;
#28873=CARTESIAN_POINT ( 'NONE',  ( 7.374560639698954034, -79.62291666666662593, 9.596002108778181494 ) ) ;
#28877=CARTESIAN_POINT ( 'NONE',  ( -10.90697944550000109, -79.57677595101699808, -0.4616983494901999996 ) ) ;
#28892=CARTESIAN_POINT ( 'NONE',  ( 2.813789756862274505, -77.64583333333332860, -10.47020627418438821 ) ) ;
#28897=CARTESIAN_POINT ( 'NONE',  ( -0.6669403506045999963, -76.25457055981898691, -12.26286337364000012 ) ) ;
#28899=AXIS2_PLACEMENT_3D ( 'NONE', #53965, #53663, #57502 ) ;
#28903=EDGE_CURVE ( 'NONE', #56437, #12329, #37671, .T. ) ;
#28911=CARTESIAN_POINT ( 'NONE',  ( -3.566334030200000171, -77.40777409222799577, 11.50986677841000017 ) ) ;
#28912=DIRECTION ( 'NONE',  ( 1.000000000000000000, 0.000000000000000000, 0.000000000000000000 ) ) ;
#28915=CARTESIAN_POINT ( 'NONE',  ( 0.9322037676993999433, -79.15839416819699181, -10.87687281004000006 ) ) ;
#28917=VERTEX_POINT ( 'NONE', #21343 ) ;
#28921=CARTESIAN_POINT ( 'NONE',  ( -9.479345976290870723, -76.20104166681831259, -5.464528704362162870 ) ) ;
#28928=CARTESIAN_POINT ( 'NONE',  ( -11.10951737771999959, -79.28970297022300429, -1.847319190731999905 ) ) ;
#28930=CARTESIAN_POINT ( 'NONE',  ( 0.3533977571636973125, -79.17711132399134044, -11.83063463211526667 ) ) ;
#28943=CARTESIAN_POINT ( 'NONE',  ( -3.140974612311405512, -77.19583333333332575, 11.68767212001977640 ) ) ;
#28944=EDGE_LOOP ( 'NONE', ( #39239, #35026, #25476, #45209 ) ) ;
#28948=CARTESIAN_POINT ( 'NONE',  ( 2.172204358709288297, -78.74132774247185296, -10.52819538874959981 ) ) ;
#28957=CARTESIAN_POINT ( 'NONE',  ( 8.822637088635000069, -80.20464915057038979, 6.926713255916000733 ) ) ;
#28967=CARTESIAN_POINT ( 'NONE',  ( 7.374560639698994002, -77.57708333333330586, -9.596002108778151296 ) ) ;
#28981=CARTESIAN_POINT ( 'NONE',  ( 11.97742283006000186, -77.88548593716899404, 0.2395971301470999903 ) ) ;
#28984=CARTESIAN_POINT ( 'NONE',  ( 10.74974228399219633, -78.85534952883524795, 0.7036061753646287720 ) ) ;
#28986=CARTESIAN_POINT ( 'NONE',  ( 10.38076106766223461, -80.87128293744233076, 2.794622580891152452 ) ) ;
#28989=CARTESIAN_POINT ( 'NONE',  ( -8.584476293286000370, -76.90617272148499239, 6.698613553322000591 ) ) ;
#28991=CARTESIAN_POINT ( 'NONE',  ( 3.140974612311377090, -78.44583333333332575, -11.68767212001978528 ) ) ;
#28993=ORIENTED_EDGE ( 'NONE', *, *, #2452, .F. ) ;
#28998=CARTESIAN_POINT ( 'NONE',  ( -9.457500717944000712, -78.37906892202299503, -6.031068363571000290 ) ) ;
#29003=CARTESIAN_POINT ( 'NONE',  ( -11.21087884115999955, -76.05337044997000362, 3.367372065805000148 ) ) ;
#29014=CARTESIAN_POINT ( 'NONE',  ( 11.68767212001977995, -77.57083333333333997, 3.140974612311385972 ) ) ;
#29023=CARTESIAN_POINT ( 'NONE',  ( -8.833962032441000645, -79.90775739383900600, 6.607787011616999884 ) ) ;
#29026=ORIENTED_EDGE ( 'NONE', *, *, #14268, .F. ) ;
#29037=CARTESIAN_POINT ( 'NONE',  ( -6.206245474241999460, -79.61997468871599892, 9.343480492029000217 ) ) ;
#29041=DIRECTION ( 'NONE',  ( 0.7071067811865474617, 0.7071067811865474617, 6.606111637375445165E-09 ) ) ;
#29047=B_SPLINE_CURVE_WITH_KNOTS ( 'NONE', 3,
 ( #57458, #35002, #57166, #43602, #34715, #7581, #12583, #25580, #56599, #38870, #44179, #3727, #39735, #17301, #25006, #34428, #16159, #11447, #34136, #7292, #29426, #47478, #43027, #56890, #29996, #20586, #38583, #3163, #43312, #2869, #20867, #16446, #21153, #4906, #30864 ),
 .UNSPECIFIED., .F., .F.,
 ( 4, 1, 1, 1, 1, 1, 1, 1, 1, 1, 1, 1, 1, 1, 1, 1, 1, 1, 1, 1, 1, 1, 1, 1, 1, 1, 1, 1, 1, 1, 1, 1, 4 ),
 ( 0.000000000000000000, 0.01250080552085842261, 0.04500075182226595527, 0.07750069812385441959, 0.1100006444252618482, 0.1425005907268503125, 0.1750005370282577410, 0.2075004833298462192, 0.2400004296312538421, 0.2725003759328423203, 0.3050003222342497766, 0.3375002685358381993, 0.3700002148372456556, 0.4025001611388341338, 0.4350001074402415346, 0.4675000537418300128, 0.5000000000432374136, 0.5324999463446450365, 0.5649998926462335147, 0.5974998389476411376, 0.6299997852492296158, 0.6624997315506371276, 0.6949996778522256058, 0.7274996241536330066, 0.7599995704552214848, 0.7924995167566288856, 0.8249994630582173638, 0.8574994093596247646, 0.8899993556612132428, 0.9224993019626208657, 0.9549992482642093439, 0.9874991945656167447, 1.000000000000000000 ),
 .UNSPECIFIED. ) ;
#29053=CARTESIAN_POINT ( 'NONE',  ( -12.00000000000000888, -77.38958333333334849, 1.570796326794847264 ) ) ;
#29064=DIRECTION ( 'NONE',  ( -1.000000000000000000, 0.000000000000000000, -2.044813970925001362E-13 ) ) ;
#29068=CARTESIAN_POINT ( 'NONE',  ( 7.422208247548548243, -79.41434947898993357, 7.776989760925737905 ) ) ;
#29081=CARTESIAN_POINT ( 'NONE',  ( 5.173492352009886552, -77.16091037829299637, -10.64243289338730314 ) ) ;
#29082=CARTESIAN_POINT ( 'NONE',  ( 4.328681851349221787, -80.25812132654044717, -9.840240413715774181 ) ) ;
#29083=CARTESIAN_POINT ( 'NONE',  ( -6.194671355491903952, -77.17629026837472850, -8.785600045674199166 ) ) ;
#29085=CIRCLE ( 'NONE', #10255, 1.499999999999999556 ) ;
#29088=CARTESIAN_POINT ( 'NONE',  ( -5.246265831776000255, -79.65519386495199683, -10.82514862071000117 ) ) ;
#29093=ORIENTED_EDGE ( 'NONE', *, *, #48434, .T. ) ;
#29106=CARTESIAN_POINT ( 'NONE',  ( -4.907978555306589108, -79.79999999999999716, -10.78460461868905185 ) ) ;
#29108=AXIS2_PLACEMENT_3D ( 'NONE', #19839, #51437, #20135 ) ;
#29110=CARTESIAN_POINT ( 'NONE',  ( -10.07624512687999996, -76.43739497653800186, -4.852130239470000106 ) ) ;
#29113=CARTESIAN_POINT ( 'NONE',  ( -1.930828380988000248, -76.56982150479699101, -10.82837744324000084 ) ) ;
#29119=CARTESIAN_POINT ( 'NONE',  ( -3.735625875409999797, -79.47660106058199858, 11.49193229459999799 ) ) ;
#29120=CARTESIAN_POINT ( 'NONE',  ( -8.973499209047250957, -78.05374552803205290, 5.919245077633647156 ) ) ;
#29137=B_SPLINE_CURVE_WITH_KNOTS ( 'NONE', 3,
 ( #40786, #20322, #6740, #24751, #36644, #28873, #18360, #6157, #56338, #2326, #381, #2043, #55462, #49954, #33003, #29447, #24165, #672 ),
 .UNSPECIFIED., .F., .F.,
 ( 4, 2, 2, 2, 2, 2, 2, 2, 4 ),
 ( 0.000000000000000000, 0.1249999999999999722, 0.2499999999999999445, 0.3749999999999998890, 0.4999999999999998890, 0.6249999999999998890, 0.7499999999999997780, 0.8749999999999998890, 1.000000000000000000 ),
 .UNSPECIFIED. ) ;
#29142=CARTESIAN_POINT ( 'NONE',  ( -0.9512330062464999791, -78.28343941728898869, 11.17646036812999988 ) ) ;
#29157=CARTESIAN_POINT ( 'NONE',  ( 0.9776138843420000279, -78.39026560866999205, -12.12546088519999898 ) ) ;
#29169=CARTESIAN_POINT ( 'NONE',  ( -9.475123589965999571, -79.03204909097999575, 5.421936826000999687 ) ) ;
#29170=ORIENTED_EDGE ( 'NONE', *, *, #48808, .T. ) ;
#29181=CARTESIAN_POINT ( 'NONE',  ( 8.596418555780450887, -77.69791666666668561, -6.606377239730321982 ) ) ;
#29186=CARTESIAN_POINT ( 'NONE',  ( -9.801255020792000394, -76.58243246625799827, 7.399866681860999940 ) ) ;
#29189=CARTESIAN_POINT ( 'NONE',  ( -10.75729140709000120, -78.77285858373909377, -3.177859684494000359 ) ) ;
#29198=CARTESIAN_POINT ( 'NONE',  ( -10.93129665128000028, -77.54342066934700028, -5.069765792968000007 ) ) ;
#29212=LINE ( 'NONE', #48120, #12311 ) ;
#29214=CARTESIAN_POINT ( 'NONE',  ( 10.02591968313939752, -76.63641906179947227, 4.955712094219922648 ) ) ;
#29225=CARTESIAN_POINT ( 'NONE',  ( 10.85425666711977755, -76.19571949791584586, 1.138855506895539493 ) ) ;
#29226=DIRECTION ( 'NONE',  ( 0.000000000000000000, -1.000000000000000000, 0.000000000000000000 ) ) ;
#29231=CARTESIAN_POINT ( 'NONE',  ( -5.007587013623000516, -76.73414604793399008, 11.54976330113999872 ) ) ;
#29232=CARTESIAN_POINT ( 'NONE',  ( 2.099707639723427555, -78.74077357293465695, -10.54285705307466969 ) ) ;
#29243=CARTESIAN_POINT ( 'NONE',  ( -0.4146318973825999787, -79.45595202224899367, -11.20920117498000046 ) ) ;
#29252=DIRECTION ( 'NONE',  ( -1.000000000000000000, 0.000000000000000000, 0.000000000000000000 ) ) ;
#29257=CARTESIAN_POINT ( 'NONE',  ( -2.112861425255000203, -79.26094992126056127, -11.84242215301999934 ) ) ;
#29263=CARTESIAN_POINT ( 'NONE',  ( 0.000000000000000000, -75.15999999999999659, 0.000000000000000000 ) ) ;
#29264=CARTESIAN_POINT ( 'NONE',  ( -7.167604382869000368, -77.55993415208399711, 9.599037027053000770 ) ) ;
#29269=CARTESIAN_POINT ( 'NONE',  ( 9.779639049769572878, -80.88431169961586420, 4.483730783971120459 ) ) ;
#29272=CARTESIAN_POINT ( 'NONE',  ( -2.149738495732000043, -78.06825668956298614, -10.82036777477999934 ) ) ;
#29274=CARTESIAN_POINT ( 'NONE',  ( -5.230597743581999914, -80.44137704144308998, 9.575199762653999969 ) ) ;
#29281=CARTESIAN_POINT ( 'NONE',  ( 1.508420534579999917, -77.63037179370199681, 11.11497989572000122 ) ) ;
#29283=CARTESIAN_POINT ( 'NONE',  ( 6.586108526242999694, -80.07391735373440156, 8.810401493720998900 ) ) ;
#29285=CARTESIAN_POINT ( 'NONE',  ( 5.913823124159999445, -76.24203414149499736, -10.61660120017000075 ) ) ;
#29294=CARTESIAN_POINT ( 'NONE',  ( 10.48543666025110710, -77.00833333333332575, -6.043427764450776785 ) ) ;
#29295=CARTESIAN_POINT ( 'NONE',  ( 12.00000000000000000, -79.54999999999999716, 0.000000000000000000 ) ) ;
#29311=CARTESIAN_POINT ( 'NONE',  ( -10.84231296956000001, -78.06411136276199159, 1.272641041331999956 ) ) ;
#29319=CYLINDRICAL_SURFACE ( 'NONE', #32944, 11.70000000000000107 ) ;
#29320=CIRCLE ( 'NONE', #36865, 11.59999999999999964 ) ;
#29328=CARTESIAN_POINT ( 'NONE',  ( 6.606377239730347739, -76.67708333333331439, -8.596418555780422466 ) ) ;
#29329=CARTESIAN_POINT ( 'NONE',  ( -7.374560639699019760, -76.82708333333329165, 9.596002108778129980 ) ) ;
#29360=CARTESIAN_POINT ( 'NONE',  ( -10.94146508061000134, -77.15133007910999652, -1.409282183016999923 ) ) ;
#29369=DIRECTION ( 'NONE',  ( -4.277603912091000087E-12, 1.000000000000000000, 1.682670357362999898E-10 ) ) ;
#29371=CARTESIAN_POINT ( 'NONE',  ( -8.734850699938000673, -79.50577571071400484, 8.271005326623001253 ) ) ;
#29387=CARTESIAN_POINT ( 'NONE',  ( -10.75000000000000355, -76.99058402040098770, 1.271990410372850544 ) ) ;
#29392=CARTESIAN_POINT ( 'NONE',  ( -5.019662172184764515, -79.80000000000001137, -10.73459069481442185 ) ) ;
#29393=CARTESIAN_POINT ( 'NONE',  ( -6.472707105664965432, -80.02684928995590496, 8.585610045933069756 ) ) ;
#29394=ADVANCED_FACE ( 'NONE', ( #3143 ), #57441, .T. ) ;
#29396=CARTESIAN_POINT ( 'NONE',  ( 9.886069181790999139, -76.54518001718498965, -5.228720670581999741 ) ) ;
#29399=CARTESIAN_POINT ( 'NONE',  ( 8.104133543071000645, -76.20111113651499579, 7.605434776855999779 ) ) ;
#29402=CONICAL_SURFACE ( 'NONE', #36949, 10.93038838648999977, 1.373400766944759877 ) ;
#29406=CARTESIAN_POINT ( 'NONE',  ( -8.325889437744001143, -79.44363262701600092, 8.917886277098999059 ) ) ;
#29408=CARTESIAN_POINT ( 'NONE',  ( -8.943304019696144636, -78.05334570480560785, 5.964714355002641355 ) ) ;
#29410=CARTESIAN_POINT ( 'NONE',  ( -3.321932689530000093, -81.00000000000000000, 10.22385755016999909 ) ) ;
#29414=ADVANCED_FACE ( 'NONE', ( #6981 ), #22356, .T. ) ;
#29425=ORIENTED_EDGE ( 'NONE', *, *, #42508, .F. ) ;
#29426=CARTESIAN_POINT ( 'NONE',  ( 8.828526701892000617, -80.44666485374948195, -6.997593314318000246 ) ) ;
#29437=ORIENTED_EDGE ( 'NONE', *, *, #31744, .T. ) ;
#29441=CARTESIAN_POINT ( 'NONE',  ( 3.299676814977999584, -78.90572260172200458, -11.70874303878999889 ) ) ;
#29446=AXIS2_PLACEMENT_3D ( 'NONE', #33684, #42853, #29252 ) ;
#29447=CARTESIAN_POINT ( 'NONE',  ( -11.68767212001979594, -79.77916666666664014, 3.140974612311315806 ) ) ;
#29449=VERTEX_POINT ( 'NONE', #34112 ) ;
#29451=CARTESIAN_POINT ( 'NONE',  ( 2.368087569675000115, -79.99857547445330397, 10.55620284977000090 ) ) ;
#29463=CARTESIAN_POINT ( 'NONE',  ( 7.103405556168159940, -78.97354755707108609, 9.415197073630089619 ) ) ;
#29470=CARTESIAN_POINT ( 'NONE',  ( -10.51110168222999874, -76.02285105332299509, 6.351495789100000344 ) ) ;
#29482=CARTESIAN_POINT ( 'NONE',  ( 5.622631719431000263, -78.77790074527499087, 10.78740717875000144 ) ) ;
#29494=CARTESIAN_POINT ( 'NONE',  ( 2.853743189566999534E-14, -82.05000000008600125, -10.29999999990999981 ) ) ;
#29502=CARTESIAN_POINT ( 'NONE',  ( 5.888733633253000477, -78.44537633716700498, -9.599841314972998418 ) ) ;
#29504=CARTESIAN_POINT ( 'NONE',  ( 1.849768683728251428, -76.71166488776647441, 11.02980055127182624 ) ) ;
#29505=CARTESIAN_POINT ( 'NONE',  ( -11.79296105283189533, -79.04295787391396289, 0.9841517631264623533 ) ) ;
#29513=DIRECTION ( 'NONE',  ( 0.000000000000000000, -1.000000000000000000, 0.000000000000000000 ) ) ;
#29514=CARTESIAN_POINT ( 'NONE',  ( -10.75000000000000000, -78.60000000000000853, 0.000000000000000000 ) ) ;
#29516=ORIENTED_EDGE ( 'NONE', *, *, #37483, .F. ) ;
#29517=ORIENTED_EDGE ( 'NONE', *, *, #53542, .F. ) ;
#29518=CARTESIAN_POINT ( 'NONE',  ( -6.786191657256999576, -76.40628414149500713, -10.60285507971000030 ) ) ;
#29519=CARTESIAN_POINT ( 'NONE',  ( 4.486458642797829910, -78.75926223335113718, -9.769447897824372617 ) ) ;
#29530=CARTESIAN_POINT ( 'NONE',  ( 5.745747329289000227, -78.66609807519598974, 9.633509135241000720 ) ) ;
#29537=CARTESIAN_POINT ( 'NONE',  ( -10.54506146704257752, -77.87759237249433397, -3.824040745093859162 ) ) ;
#29546=CARTESIAN_POINT ( 'NONE',  ( -11.22206352832999876, -79.67932075312558027, -4.332716936452000844 ) ) ;
#29549=ORIENTED_EDGE ( 'NONE', *, *, #26512, .T. ) ;
#29554=CARTESIAN_POINT ( 'NONE',  ( 2.697636866285999968, -77.70918012219799209, -11.67213861177999945 ) ) ;
#29560=CARTESIAN_POINT ( 'NONE',  ( -10.47083672843175783, -76.58144398812963516, 2.512152686489665054 ) ) ;
#29561=CARTESIAN_POINT ( 'NONE',  ( -9.367668485852000515, -77.41458445751899831, 5.826535979523000286 ) ) ;
#29562=CARTESIAN_POINT ( 'NONE',  ( 9.393203674808285442, -79.20833333333332860, -5.413904038987152667 ) ) ;
#29569=CARTESIAN_POINT ( 'NONE',  ( -9.998780405325002008, -77.30353567768000289, -5.083552005986999411 ) ) ;
#29573=CARTESIAN_POINT ( 'NONE',  ( -11.10423584941000108, -77.10988712250798471, -4.937773032316999711 ) ) ;
#29589=CARTESIAN_POINT ( 'NONE',  ( 0.000000000000000000, -87.70000000000000284, 0.000000000000000000 ) ) ;
#29590=ORIENTED_EDGE ( 'NONE', *, *, #14177, .F. ) ;
#29595=ADVANCED_FACE ( 'NONE', ( #8719 ), #26710, .F. ) ;
#29597=CARTESIAN_POINT ( 'NONE',  ( -0.9257816722924000485, -77.95516599075499187, 10.87742130684000053 ) ) ;
#29603=CARTESIAN_POINT ( 'NONE',  ( -2.047671225339077468E-06, -76.25353340279926329, -10.79679441329301959 ) ) ;
#29617=EDGE_CURVE ( 'NONE', #42760, #28272, #17168, .T. ) ;
#29620=EDGE_CURVE ( 'NONE', #24195, #10296, #1343, .T. ) ;
#29623=CARTESIAN_POINT ( 'NONE',  ( 9.450487096927000508, -77.89901585959799490, -7.362360902974999455 ) ) ;
#29629=CARTESIAN_POINT ( 'NONE',  ( -12.00000000000000000, -79.29999999999999716, 0.000000000000000000 ) ) ;
#29638=CARTESIAN_POINT ( 'NONE',  ( 2.814035350851149087, -76.95432989093133358, 10.47073005108091692 ) ) ;
#29646=CARTESIAN_POINT ( 'NONE',  ( -8.675294248905000671, -77.65483863155199629, 6.999562148146999618 ) ) ;
#29655=CARTESIAN_POINT ( 'NONE',  ( 8.554245750310725427, -80.04392919279416674, -7.255790090871102826 ) ) ;
#29656=CARTESIAN_POINT ( 'NONE',  ( -2.112861425255000203, -79.10926721811499363, -11.84242215301999934 ) ) ;
#29660=CARTESIAN_POINT ( 'NONE',  ( -7.330610599118999815, -79.25481274797898834, 8.549626471514999437 ) ) ;
#29664=ORIENTED_EDGE ( 'NONE', *, *, #5634, .F. ) ;
#29677=CARTESIAN_POINT ( 'NONE',  ( 9.290912487798001607, -79.80000000000001137, 7.341183704965414947 ) ) ;
#29678=CARTESIAN_POINT ( 'NONE',  ( -9.805087678983213095, -80.06653000188077840, 4.415917898387408336 ) ) ;
#29681=CARTESIAN_POINT ( 'NONE',  ( -1.660522255173999984, -76.72075361110900360, 11.05968181062000077 ) ) ;
#29693=CARTESIAN_POINT ( 'NONE',  ( -8.948369457197285826, -78.05341261098192263, 5.957113593040013200 ) ) ;
#29694=DIRECTION ( 'NONE',  ( -1.000000000000000000, 0.000000000000000000, 0.000000000000000000 ) ) ;
#29699=CIRCLE ( 'NONE', #4259, 11.70000000000000107 ) ;
#29702=ADVANCED_FACE ( 'NONE', ( #1525 ), #42146, .F. ) ;
#29705=ADVANCED_FACE ( 'NONE', ( #33076 ), #37081, .F. ) ;
#29717=CARTESIAN_POINT ( 'NONE',  ( 3.211701487445925984, -79.95131508034484114, 10.27501478995334949 ) ) ;
#29744=CARTESIAN_POINT ( 'NONE',  ( 6.205001111027785399, -80.17721126027063860, 9.095289649731126858 ) ) ;
#29745=CARTESIAN_POINT ( 'NONE',  ( 11.95248949435000085, -78.90537670790513403, 0.8087524912306001124 ) ) ;
#29754=CARTESIAN_POINT ( 'NONE',  ( -3.140974612311351777, -77.90416666666665435, -11.68767212001978884 ) ) ;
#29762=CONICAL_SURFACE ( 'NONE', #51604, 10.93038838648999977, 1.373400766944759877 ) ;
#29763=CARTESIAN_POINT ( 'NONE',  ( -3.132815200277000223, -78.04540922883299459, -11.75448848339000030 ) ) ;
#29772=CARTESIAN_POINT ( 'NONE',  ( 2.198909403236999793, -79.76316569920798827, -11.72178803194999830 ) ) ;
#29776=DIRECTION ( 'NONE',  ( 0.000000000000000000, -1.000000000000000000, 0.000000000000000000 ) ) ;
#29781=CARTESIAN_POINT ( 'NONE',  ( 9.699999999837999098, -87.69999999983798489, 3.624870943809000214E-09 ) ) ;
#29782=CARTESIAN_POINT ( 'NONE',  ( 9.458574655020427713, -79.24897924367529356, -7.006660078105245937 ) ) ;
#29798=CARTESIAN_POINT ( 'NONE',  ( 0.03331989244325999494, -76.20137044996999975, 12.04427157219000044 ) ) ;
#29799=CARTESIAN_POINT ( 'NONE',  ( -7.103738426970670261, -78.66783617555775265, -8.098733187644580056 ) ) ;
#29813=CARTESIAN_POINT ( 'NONE',  ( 2.407803015296000382, -80.25912183657409571, 10.73324203768999929 ) ) ;
#29824=CARTESIAN_POINT ( 'NONE',  ( 5.151396044562439158, -77.68693797148132774, 9.964172206255058839 ) ) ;
#29826=LINE ( 'NONE', #47301, #32269 ) ;
#29839=CARTESIAN_POINT ( 'NONE',  ( 10.42503750987000011, -77.27511107541700142, -5.902083371034000159 ) ) ;
#29846=CARTESIAN_POINT ( 'NONE',  ( 1.468061006981000061, -77.89085666695899590, 10.81758581523999929 ) ) ;
#29852=CARTESIAN_POINT ( 'NONE',  ( -1.824767972787999959, -79.93971326159969237, -12.13485939589000040 ) ) ;
#29854=CARTESIAN_POINT ( 'NONE',  ( -8.729704736439998669, -77.77986937598299733, 7.043462628994999974 ) ) ;
#29863=CARTESIAN_POINT ( 'NONE',  ( -8.917244775899000331, -78.69123101036599621, -6.494958043606000153 ) ) ;
#29866=CIRCLE ( 'NONE', #28899, 10.25000000000000000 ) ;
#29868=CARTESIAN_POINT ( 'NONE',  ( 11.68767212001979594, -77.02916666666669698, -3.140974612311341563 ) ) ;
#29881=ORIENTED_EDGE ( 'NONE', *, *, #26750, .T. ) ;
#29886=CARTESIAN_POINT ( 'NONE',  ( 1.694996965211734263, -76.26093750039238728, -10.68870303814569311 ) ) ;
#29889=ORIENTED_EDGE ( 'NONE', *, *, #45937, .T. ) ;
#29902=AXIS2_PLACEMENT_3D ( 'NONE', #9198, #13908, #48484 ) ;
#29905=CARTESIAN_POINT ( 'NONE',  ( 8.272973658470998970, -78.38734353722499293, -8.664523719228998999 ) ) ;
#29914=CARTESIAN_POINT ( 'NONE',  ( 7.110505486850000167, -78.57249282818800395, -8.302835368086999068 ) ) ;
#29920=CARTESIAN_POINT ( 'NONE',  ( -12.50000000000000000, -91.29999999999999716, -2.556024836231000547E-12 ) ) ;
#29924=CARTESIAN_POINT ( 'NONE',  ( -10.74976571963693317, -77.09494490966720548, 0.7036152397608054221 ) ) ;
#29932=CARTESIAN_POINT ( 'NONE',  ( 0.2638252682412000061, -78.33574720659700574, -11.14383981435000059 ) ) ;
#29938=CARTESIAN_POINT ( 'NONE',  ( 7.235888310811381174, -80.28381975494082212, -7.950577990028921960 ) ) ;
#29940=CARTESIAN_POINT ( 'NONE',  ( -5.394504329618741600, -79.93498382078693965, -9.834680065944747085 ) ) ;
#29941=CARTESIAN_POINT ( 'NONE',  ( -11.95950202284999975, -79.05752124800099523, 1.295167635372999948 ) ) ;
#29944=CARTESIAN_POINT ( 'NONE',  ( 11.20174477810000013, -79.58164886400000171, 1.163992476170999879 ) ) ;
#29946=CARTESIAN_POINT ( 'NONE',  ( 1.407258332515630483, -77.46462077040253291, 10.74994165454338635 ) ) ;
#29951=ORIENTED_EDGE ( 'NONE', *, *, #22959, .T. ) ;
#29957=ORIENTED_EDGE ( 'NONE', *, *, #46553, .T. ) ;
#29964=FACE_OUTER_BOUND ( 'NONE', #12821, .T. ) ;
#29966=PRODUCT_DEFINITION_SHAPE ( 'NONE', 'NONE',  #55670 ) ;
#29967=CARTESIAN_POINT ( 'NONE',  ( -6.634760531095161618, -80.02836359101850405, 8.459757256220747479 ) ) ;
#29970=CARTESIAN_POINT ( 'NONE',  ( -5.007180289739999068, -76.74583555309799010, 10.00009952528999868 ) ) ;
#29973=CARTESIAN_POINT ( 'NONE',  ( 11.02958081164000070, -76.15094725253700858, 1.366722674935999970 ) ) ;
#29979=CARTESIAN_POINT ( 'NONE',  ( -2.672184218513227627, -77.99512583853751835, 10.41389279075909791 ) ) ;
#29986=CARTESIAN_POINT ( 'NONE',  ( -0.7446082967701639355, -79.17994009691294366, 12.02413132939186724 ) ) ;
#29988=DIRECTION ( 'NONE',  ( 1.000000000000000000, 0.000000000000000000, 0.000000000000000000 ) ) ;
#29996=CARTESIAN_POINT ( 'NONE',  ( -6.474781754604000739, -80.32627410973498172, -9.218806710208998112 ) ) ;
#30004=CARTESIAN_POINT ( 'NONE',  ( 0.9032081954762855025, -79.96855000297721006, 10.71863955025375148 ) ) ;
#30007=CARTESIAN_POINT ( 'NONE',  ( 10.66187250086873561, -77.33868385048562288, -1.541903100460451537 ) ) ;
#30016=CARTESIAN_POINT ( 'NONE',  ( 10.63100742340999894, -77.54925683053299679, 5.913054471243999188 ) ) ;
#30033=CARTESIAN_POINT ( 'NONE',  ( -10.30095950721840481, -80.88213540149526182, -4.424346738711788518 ) ) ;
#30042=CARTESIAN_POINT ( 'NONE',  ( -8.598496321198998871, -77.06159643427999129, -8.768570137950998600 ) ) ;
#30052=CARTESIAN_POINT ( 'NONE',  ( 11.38106369370999893, -77.71985744374799765, 4.295802577524999499 ) ) ;
#30058=DIRECTION ( 'NONE',  ( 1.000000000000000000, 0.000000000000000000, 3.332461511940999929E-11 ) ) ;
#30062=CARTESIAN_POINT ( 'NONE',  ( 10.38331776012999974, -79.55238262701600149, 6.321536042210999184 ) ) ;
#30064=CARTESIAN_POINT ( 'NONE',  ( 11.44842197274081030, -79.67499999999999716, 3.717781425818833529 ) ) ;
#30065=CARTESIAN_POINT ( 'NONE',  ( -8.669743459559573040, -76.20755208352487386, -6.663793442645963516 ) ) ;
#30073=CARTESIAN_POINT ( 'NONE',  ( 6.233047529871999615, -78.88050366622999832, 9.960502923565000444 ) ) ;
#30077=B_SPLINE_CURVE_WITH_KNOTS ( 'NONE', 3,
 ( #6946, #7235, #25240, #43259, #38816, #56833, #16389, #52407, #49729, #18428 ),
 .UNSPECIFIED., .F., .F.,
 ( 4, 2, 2, 2, 4 ),
 ( 0.000000000000000000, 0.2500000000000000000, 0.5000000000000000000, 0.7500000000000000000, 1.000000000000000000 ),
 .UNSPECIFIED. ) ;
#30086=CARTESIAN_POINT ( 'NONE',  ( 2.612329186234000122, -77.18495616928899494, 12.31457248274999827 ) ) ;
#30088=CARTESIAN_POINT ( 'NONE',  ( 5.336354586632489294, -78.76643638245003842, -9.332050835440680814 ) ) ;
#30098=CARTESIAN_POINT ( 'NONE',  ( 5.413930304708984842, -79.76668259678613992, -9.393115503636845887 ) ) ;
#30101=CARTESIAN_POINT ( 'NONE',  ( 10.58946819037999987, -78.62494125646499299, -3.698823201301000285 ) ) ;
#30110=VECTOR ( 'NONE', #6868, 1000.000000000000227 ) ;
#30116=CARTESIAN_POINT ( 'NONE',  ( -5.413904038987206846, -80.91666666666667140, 9.393203674808249914 ) ) ;
#30123=DIRECTION ( 'NONE',  ( 0.000000000000000000, -1.000000000000000000, 0.000000000000000000 ) ) ;
#30124=CARTESIAN_POINT ( 'NONE',  ( 0.000000000000000000, -92.13603921945998820, 0.000000000000000000 ) ) ;
#30128=DIRECTION ( 'NONE',  ( 0.000000000000000000, -1.000000000000000000, 0.000000000000000000 ) ) ;
#30129=CARTESIAN_POINT ( 'NONE',  ( 0.4844284812283000119, -77.43788696795999726, 11.97002061314999999 ) ) ;
#30132=CARTESIAN_POINT ( 'NONE',  ( -3.708203932498999933, -76.29999999999999716, 11.41267819554000162 ) ) ;
#30135=CARTESIAN_POINT ( 'NONE',  ( -10.30489194730139602, -76.57673360226559112, 3.128758578913356292 ) ) ;
#30139=EDGE_CURVE ( 'NONE', #4324, #20196, #36930, .T. ) ;
#30148=CARTESIAN_POINT ( 'NONE',  ( 8.243508989658998587, -76.32523803030200327, 9.088020496884999133 ) ) ;
#30152=CARTESIAN_POINT ( 'NONE',  ( 1.092964466808999946, -79.57604836483399424, 11.09324250366999998 ) ) ;
#30164=ORIENTED_EDGE ( 'NONE', *, *, #58029, .T. ) ;
#30174=CARTESIAN_POINT ( 'NONE',  ( 1.711430185772882417, -81.00000000000000000, -10.87976356598724159 ) ) ;
#30197=CARTESIAN_POINT ( 'NONE',  ( -11.48784787867999846, -78.22456764468299184, -3.397854551190000016 ) ) ;
#30199=VECTOR ( 'NONE', #6511, 1000.000000000000000 ) ;
#30206=CARTESIAN_POINT ( 'NONE',  ( 3.988644160859999399, -78.54525648518600178, -10.40888963995999994 ) ) ;
#30210=DIRECTION ( 'NONE',  ( 0.000000000000000000, 1.000000000000000000, 0.000000000000000000 ) ) ;
#30216=CARTESIAN_POINT ( 'NONE',  ( -10.20081059776443944, -77.07411305503957522, 3.463749923433618871 ) ) ;
#30225=EDGE_CURVE ( 'NONE', #49519, #54390, #10185, .T. ) ;
#30228=CARTESIAN_POINT ( 'NONE',  ( -10.77981876821000107, -77.12409373610799435, 2.344619735928000104 ) ) ;
#30234=CARTESIAN_POINT ( 'NONE',  ( -4.104898415690168889, -80.19419946738641158, -9.935154032304627236 ) ) ;
#30236=CARTESIAN_POINT ( 'NONE',  ( -8.982242211535060861, -79.79880210577779565, 6.718700307134141347 ) ) ;
#30237=CARTESIAN_POINT ( 'NONE',  ( -5.246265831776000255, -79.58740531167599386, -10.82514862071000117 ) ) ;
#30239=CARTESIAN_POINT ( 'NONE',  ( -11.08513710546999853, -79.30928543398199793, 1.988391287278999942 ) ) ;
#30240=CARTESIAN_POINT ( 'NONE',  ( -10.47050256948984526, -77.57917301698132917, 2.813946892465741367 ) ) ;
#30256=DIRECTION ( 'NONE',  ( 0.000000000000000000, -1.000000000000000000, 0.000000000000000000 ) ) ;
#30258=CARTESIAN_POINT ( 'NONE',  ( -9.166035821854576326, -80.05650656212442584, 5.627461772928610273 ) ) ;
#30261=CARTESIAN_POINT ( 'NONE',  ( 5.380788203752000065, -76.16895088734899844, 9.804131929786001010 ) ) ;
#30264=CARTESIAN_POINT ( 'NONE',  ( 4.823055945868000016, -76.61998538877500664, -9.885342059496000644 ) ) ;
#30296=CARTESIAN_POINT ( 'NONE',  ( 4.190783791506424549, -79.94328038420290738, 9.899395638210270576 ) ) ;
#30307=CARTESIAN_POINT ( 'NONE',  ( 8.042137835475001495, -77.57638614595698812, 9.127242153301999394 ) ) ;
#30315=ORIENTED_EDGE ( 'NONE', *, *, #54871, .F. ) ;
#30321=B_SPLINE_CURVE_WITH_KNOTS ( 'NONE', 3,
 ( #35018, #9641, #26748, #22632, #27041, #4921, #40346, #5491, #31762, #40937, #4631, #41512, #45377, #45080, #31464, #27628, #22922, #524 ),
 .UNSPECIFIED., .F., .F.,
 ( 4, 2, 2, 2, 2, 2, 2, 2, 4 ),
 ( 0.000000000000000000, 0.1249999999999999445, 0.2499999999999998890, 0.3749999999999998335, 0.4999999999999998890, 0.6249999999999998890, 0.7500000000000000000, 0.8750000000000000000, 1.000000000000000000 ),
 .UNSPECIFIED. ) ;
#30325=CARTESIAN_POINT ( 'NONE',  ( 3.925078296951999501, -78.49843697654912944, 11.31856107452000337 ) ) ;
#30340=CARTESIAN_POINT ( 'NONE',  ( 3.113245456484129203, -78.43116804080246141, -10.55002948983070610 ) ) ;
#30342=CARTESIAN_POINT ( 'NONE',  ( 9.596418076563999477, -77.63846949747699000, -7.476047798475000228 ) ) ;
#30343=DIRECTION ( 'NONE',  ( -1.000000000000000000, 0.000000000000000000, 0.000000000000000000 ) ) ;
#30344=CARTESIAN_POINT ( 'NONE',  ( 5.413904038987179312, -79.16666666666662877, -9.393203674808262349 ) ) ;
#30348=CARTESIAN_POINT ( 'NONE',  ( -4.868526683403212374, -79.51253823190735659, 9.584316550000758994 ) ) ;
#30351=CARTESIAN_POINT ( 'NONE',  ( 4.729501432732000410, -79.84864851751980552, -10.91094243975000033 ) ) ;
#30361=VERTEX_POINT ( 'NONE', #31933 ) ;
#30362=CARTESIAN_POINT ( 'NONE',  ( -14.00000000000000000, -91.29999999999999716, 0.000000000000000000 ) ) ;
#30371=CARTESIAN_POINT ( 'NONE',  ( -10.07979664880000037, -76.57175206120300004, 3.736335038366999761 ) ) ;
#30379=EDGE_LOOP ( 'NONE', ( #37823, #12196, #10527, #53326, #36075, #34457 ) ) ;
#30380=ORIENTED_EDGE ( 'NONE', *, *, #25590, .T. ) ;
#30381=CARTESIAN_POINT ( 'NONE',  ( -8.731271169595000714, -77.32214279640000143, -8.903971204279999441 ) ) ;
#30382=CARTESIAN_POINT ( 'NONE',  ( -9.574728980326261407, -78.63772619795470575, -4.887204237426289843 ) ) ;
#30386=ADVANCED_FACE ( 'NONE', ( #13645 ), #31640, .F. ) ;
#30394=CARTESIAN_POINT ( 'NONE',  ( -0.2291600886666000092, -78.52507466545799275, -11.06898422383999936 ) ) ;
#30403=CARTESIAN_POINT ( 'NONE',  ( 11.22546153480763564, -77.12033577748668733, -4.386301564758396054 ) ) ;
#30422=CARTESIAN_POINT ( 'NONE',  ( -7.615853692923001184, -78.42814171621100172, 9.247423260715999405 ) ) ;
#30430=VERTEX_POINT ( 'NONE', #40811 ) ;
#30435=CYLINDRICAL_SURFACE ( 'NONE', #48403, 10.75000000000000000 ) ;
#30439=EDGE_CURVE ( 'NONE', #21876, #8361, #18676, .T. ) ;
#30441=CARTESIAN_POINT ( 'NONE',  ( 0.4218791420769999467, -76.06884727436400340, -12.37978857546999834 ) ) ;
#30444=CARTESIAN_POINT ( 'NONE',  ( 9.317996701405999005, -79.41263030682299018, -6.117968457212000111 ) ) ;
#30452=PRODUCT ( 'Push Button Case', 'Push Button Case', '', ( #28733 ) ) ;
#30453=CARTESIAN_POINT ( 'NONE',  ( 10.03503830778000072, -79.02770829698199861, -7.077696433220999950 ) ) ;
#30467=CARTESIAN_POINT ( 'NONE',  ( -1.539492778512501880, -81.00000000000001421, -10.83296861242082443 ) ) ;
#30470=CARTESIAN_POINT ( 'NONE',  ( 6.160618408503998999, -77.90069330475100173, 9.012333039518999556 ) ) ;
#30475=CARTESIAN_POINT ( 'NONE',  ( 5.622824352109999424, -79.93289032900889879, -9.705769245306999693 ) ) ;
#30490=CARTESIAN_POINT ( 'NONE',  ( 8.112534416287001449, -79.82597756633930430, 9.112389163837999462 ) ) ;
#30492=CARTESIAN_POINT ( 'NONE',  ( 9.789819849890999848, -78.90280053027699125, -6.904744247936999813 ) ) ;
#30498=CARTESIAN_POINT ( 'NONE',  ( -10.87500000000999911, -76.17499999999400018, 1.221063213659000093E-09 ) ) ;
#30499=CARTESIAN_POINT ( 'NONE',  ( 11.06080859785000037, -77.08847592767999402, 2.119546583493000291 ) ) ;
#30501=CARTESIAN_POINT ( 'NONE',  ( -11.23644965357999936, -80.31873890621510270, 0.6602389571347000441 ) ) ;
#30518=CARTESIAN_POINT ( 'NONE',  ( -9.992683672509999226, -78.17232914858600168, 4.939724043997999914 ) ) ;
#30524=CARTESIAN_POINT ( 'NONE',  ( 2.099527108784107199, -80.24101286911570696, -10.54274609721885092 ) ) ;
#30528=CARTESIAN_POINT ( 'NONE',  ( -11.15966350340000091, -79.46787078828600670, 4.490997254915999548 ) ) ;
#30533=ORIENTED_EDGE ( 'NONE', *, *, #15522, .F. ) ;
#30540=CARTESIAN_POINT ( 'NONE',  ( 6.585359383873000461, -79.24993983499498995, -8.706802385234000852 ) ) ;
#30545=CARTESIAN_POINT ( 'NONE',  ( 8.899186938125001944, -76.04999999999999716, 6.465637775217000005 ) ) ;
#30551=CARTESIAN_POINT ( 'NONE',  ( -10.41537882044915264, -80.08004720311535607, 2.677681550047262604 ) ) ;
#30552=FACE_OUTER_BOUND ( 'NONE', #54803, .T. ) ;
#30559=CARTESIAN_POINT ( 'NONE',  ( -9.806643590720000248, -76.56230274324299501, -4.722305910095999870 ) ) ;
#30562=CARTESIAN_POINT ( 'NONE',  ( 6.043427764450761686, -76.63333333333329733, 10.48543666025110888 ) ) ;
#30570=CARTESIAN_POINT ( 'NONE',  ( -1.407171709420443895, -80.11458333333332860, -10.74999999999999645 ) ) ;
#30588=CARTESIAN_POINT ( 'NONE',  ( 5.777098977877974662, -79.93015161712408201, 9.071507582019696869 ) ) ;
#30591=CARTESIAN_POINT ( 'NONE',  ( 9.599999999916001059, -90.40000000008399184, -6.531555804621000072E-10 ) ) ;
#30594=EDGE_LOOP ( 'NONE', ( #16210, #8326, #38034, #16767, #26045 ) ) ;
#30600=VERTEX_POINT ( 'NONE', #13728 ) ;
#30602=EDGE_CURVE ( 'NONE', #17785, #38899, #53037, .T. ) ;
#30605=AXIS2_PLACEMENT_3D ( 'NONE', #22216, #44665, #26059 ) ;
#30634=CARTESIAN_POINT ( 'NONE',  ( -8.689305806348999184, -77.50282292035799969, -8.513430283325000403 ) ) ;
#30639=CARTESIAN_POINT ( 'NONE',  ( -4.456894928553262858, -79.50918558175608553, 9.783918442212431898 ) ) ;
#30642=CARTESIAN_POINT ( 'NONE',  ( -12.00003092673000005, -79.69772460938399661, -0.9957469300414000246 ) ) ;
#30644=CARTESIAN_POINT ( 'NONE',  ( 11.11995425589478081, -79.68125000000000568, 4.608132131667403542 ) ) ;
#30647=DIRECTION ( 'NONE',  ( 0.000000000000000000, 1.000000000000000000, 0.000000000000000000 ) ) ;
#30657=ORIENTED_EDGE ( 'NONE', *, *, #44288, .T. ) ;
#30665=ORIENTED_EDGE ( 'NONE', *, *, #18523, .F. ) ;
#30666=ORIENTED_EDGE ( 'NONE', *, *, #4331, .F. ) ;
#30667=CARTESIAN_POINT ( 'NONE',  ( -10.91969632658999956, -76.22984727436399055, -5.774793620716000220 ) ) ;
#30694=DIRECTION ( 'NONE',  ( -1.000000000000000000, 0.000000000000000000, 0.000000000000000000 ) ) ;
#30704=CARTESIAN_POINT ( 'NONE',  ( 10.99419336675999936, -78.78082281672000420, 4.758540471090999979 ) ) ;
#30710=CARTESIAN_POINT ( 'NONE',  ( 10.48543666025110710, -78.50833333333332575, -6.043427764450776785 ) ) ;
#30718=CARTESIAN_POINT ( 'NONE',  ( -10.58728162385000005, -77.80710571898499950, 3.705074683290000337 ) ) ;
#30721=CARTESIAN_POINT ( 'NONE',  ( 6.695644564036999924, -77.11278636746699533, -10.05404869174999938 ) ) ;
#30726=CARTESIAN_POINT ( 'NONE',  ( 8.503062319121001522, -78.44610392334999460, 7.028489548493999983 ) ) ;
#30731=B_SPLINE_CURVE_WITH_KNOTS ( 'NONE', 3,
 ( #29603, #47659, #29886, #20192, #43206, #2765, #20763, #38186, #16343, #47944 ),
 .UNSPECIFIED., .F., .F.,
 ( 4, 2, 2, 2, 4 ),
 ( 0.6250000037914531514, 0.7187500028435899191, 0.8125000018957265757, 0.9062500009478633434, 1.000000000000000000 ),
 .UNSPECIFIED. ) ;
#30732=CARTESIAN_POINT ( 'NONE',  ( 5.407950800604435670, -76.33333333333332860, 9.358624512123000727 ) ) ;
#30734=CARTESIAN_POINT ( 'NONE',  ( 12.25187917533000004, -79.08196692782999548, 0.8290103756198000662 ) ) ;
#30736=EDGE_LOOP ( 'NONE', ( #44523, #14054, #12891 ) ) ;
#30750=CARTESIAN_POINT ( 'NONE',  ( 10.17013595917000046, -77.85947499715699394, -4.274350120612000481 ) ) ;
#30753=CARTESIAN_POINT ( 'NONE',  ( -6.324515969367999979, -78.77564805565999961, -9.263833350438000380 ) ) ;
#30770=CARTESIAN_POINT ( 'NONE',  ( -6.443880121360000324, -79.99798052329479958, 9.772379853565000829 ) ) ;
#30772=CARTESIAN_POINT ( 'NONE',  ( -4.743879332790999825, -78.79428326858199227, -11.00053059214000051 ) ) ;
#30781=CARTESIAN_POINT ( 'NONE',  ( 11.13061814830999907, -77.06123958467900081, -1.715606072514000102 ) ) ;
#30783=CARTESIAN_POINT ( 'NONE',  ( 2.063852278220999814, -80.96308337030230007, -11.06498607923999877 ) ) ;
#30791=FACE_OUTER_BOUND ( 'NONE', #15885, .T. ) ;
#30792=CONICAL_SURFACE ( 'NONE', #9114, 13.94999999993999928, 0.7853981633972997312 ) ;
#30801=CARTESIAN_POINT ( 'NONE',  ( -10.79885705035999877, -76.72880296949000467, -2.763914921897999921 ) ) ;
#30807=CARTESIAN_POINT ( 'NONE',  ( 0.1721334691643799375, -80.22656007235991638, -10.74864075682200593 ) ) ;
#30814=CARTESIAN_POINT ( 'NONE',  ( 10.75000000000000355, -78.74148622562242394, -1.150112874675813579 ) ) ;
#30824=CARTESIAN_POINT ( 'NONE',  ( -3.912255148455999976, -78.97757640497698617, 10.19164489391000217 ) ) ;
#30839=CARTESIAN_POINT ( 'NONE',  ( 8.332845033087998843, -76.09460843601999613, -7.273191856730000460 ) ) ;
#30842=FACE_OUTER_BOUND ( 'NONE', #36762, .T. ) ;
#30849=CARTESIAN_POINT ( 'NONE',  ( -6.711381441964999972, -80.25968072146179111, 9.048015653393999713 ) ) ;
#30859=AXIS2_PLACEMENT_3D ( 'NONE', #13347, #694, #44659 ) ;
#30863=ADVANCED_FACE ( 'NONE', ( #24562 ), #46438, .T. ) ;
#30864=CARTESIAN_POINT ( 'NONE',  ( 6.586108526242999694, -80.07391735373440156, 8.810401493720998900 ) ) ;
#30868=CARTESIAN_POINT ( 'NONE',  ( -6.043427764450784778, -78.98333333333332007, -10.48543666025109822 ) ) ;
#30872=CARTESIAN_POINT ( 'NONE',  ( 1.612132099153596565, -79.96332688086813789, 10.62905773014771071 ) ) ;
#30875=CARTESIAN_POINT ( 'NONE',  ( -2.397279086078224708, -77.20726813167010505, -10.47917899088556126 ) ) ;
#30886=CARTESIAN_POINT ( 'NONE',  ( 11.99621472858000004, -77.52212751510998601, 2.018255885614000267 ) ) ;
#30892=ORIENTED_EDGE ( 'NONE', *, *, #56411, .F. ) ;
#30897=CARTESIAN_POINT ( 'NONE',  ( -12.00000000000000000, -77.89999999999999147, -2.795183092923000262E-14 ) ) ;
#30917=CARTESIAN_POINT ( 'NONE',  ( -8.496131438301000927, -77.97256569596500242, 6.855006679309999740 ) ) ;
#30918=CARTESIAN_POINT ( 'NONE',  ( -11.03570087982000025, -77.47569360493399415, -5.118186854384000561 ) ) ;
#30920=CARTESIAN_POINT ( 'NONE',  ( 6.585791278903703194, -80.14058402040107865, 8.809977328666299456 ) ) ;
#30925=CARTESIAN_POINT ( 'NONE',  ( 7.303865428629999990, -79.08185514870999100, 9.528096774331999086 ) ) ;
#30926=CARTESIAN_POINT ( 'NONE',  ( 3.207556080690000311, -80.92498568429859063, 10.58040010179999868 ) ) ;
#30927=CARTESIAN_POINT ( 'NONE',  ( 11.70000000000000107, -76.00000000000000000, 0.000000000000000000 ) ) ;
#30928=CARTESIAN_POINT ( 'NONE',  ( -4.531904799951000484, -77.42579691695999600, -10.26060180864999971 ) ) ;
#30946=EDGE_LOOP ( 'NONE', ( #41999, #39615, #30657, #23884, #17205 ) ) ;
#30952=CARTESIAN_POINT ( 'NONE',  ( 10.22898553533000054, -76.39377822758400782, -6.925005706880000389 ) ) ;
#30956=EDGE_CURVE ( 'NONE', #2822, #15288, #40052, .T. ) ;
#30962=CARTESIAN_POINT ( 'NONE',  ( -0.8253947190444999027, -77.36913936749189702, -11.18645762290999990 ) ) ;
#30965=CARTESIAN_POINT ( 'NONE',  ( 6.879576957522999692, -79.22414080250499069, 8.859431780707000215 ) ) ;
#30981=CARTESIAN_POINT ( 'NONE',  ( 0.4713521909880000194, -79.02188087448040221, 12.02020425643999957 ) ) ;
#30989=CARTESIAN_POINT ( 'NONE',  ( 0.000000000000000000, -75.15999999999999659, 0.000000000000000000 ) ) ;
#31008=CARTESIAN_POINT ( 'NONE',  ( 12.05139359237000107, -76.67257108724299997, -2.863729330572000187 ) ) ;
#31010=CARTESIAN_POINT ( 'NONE',  ( 7.444278262535061863, -76.81467768451751965, 7.855135693196025670 ) ) ;
#31012=CARTESIAN_POINT ( 'NONE',  ( 2.143349548760000278, -78.50057660935300419, 10.82163513946999878 ) ) ;
#31020=CARTESIAN_POINT ( 'NONE',  ( 11.65296779515999859, -78.05105294172599883, -3.873515295708999773 ) ) ;
#31023=DIRECTION ( 'NONE',  ( 0.000000000000000000, -1.000000000000000000, 0.000000000000000000 ) ) ;
#31034=CARTESIAN_POINT ( 'NONE',  ( -6.771245932390999478, -78.21354745617999527, -8.709304295962999376 ) ) ;
#31038=CARTESIAN_POINT ( 'NONE',  ( 11.14115696400000033, -78.93906611367098947, -1.301050381412999890 ) ) ;
#31040=ORIENTED_EDGE ( 'NONE', *, *, #3026, .F. ) ;
#31041=VERTEX_POINT ( 'NONE', #43739 ) ;
#31055=VERTEX_POINT ( 'NONE', #39004 ) ;
#31056=CARTESIAN_POINT ( 'NONE',  ( 11.41978910860999896, -79.65576480666599934, 4.917167810709999642 ) ) ;
#31058=CARTESIAN_POINT ( 'NONE',  ( -2.132471413802949467, -77.99102497083757157, 10.53628444161482847 ) ) ;
#31059=CARTESIAN_POINT ( 'NONE',  ( 10.18066396183999878, -78.42807224564398894, 6.314281093748000728 ) ) ;
#31066=CARTESIAN_POINT ( 'NONE',  ( -5.774605976465999824, -77.90556621773498591, -9.668913608825000949 ) ) ;
#31068=CARTESIAN_POINT ( 'NONE',  ( 7.473878879214000293, -80.13975433285759209, 8.225614977841999576 ) ) ;
#31085=CARTESIAN_POINT ( 'NONE',  ( 0.2665495375979999859, -78.40347427100999766, -11.25891151133000001 ) ) ;
#31091=CARTESIAN_POINT ( 'NONE',  ( 2.105548162849785854, -80.24105674942582311, -10.54154672537324267 ) ) ;
#31093=CARTESIAN_POINT ( 'NONE',  ( 10.05842956770407604, -79.06342084472876763, -4.964836713854746009 ) ) ;
#31095=CARTESIAN_POINT ( 'NONE',  ( 0.000000000000000000, -79.79999999999999716, 0.000000000000000000 ) ) ;
#31096=CARTESIAN_POINT ( 'NONE',  ( -9.674930971187000850, -79.34977615539300189, 5.536272326541999078 ) ) ;
#31098=VERTEX_POINT ( 'NONE', #43160 ) ;
#31099=VERTEX_POINT ( 'NONE', #57877 ) ;
#31105=CARTESIAN_POINT ( 'NONE',  ( -6.103876716051000351, -79.56279398642399769, 9.189364690594999274 ) ) ;
#31159=CARTESIAN_POINT ( 'NONE',  ( -4.684264787344456948, -77.18914283860964076, -9.675737980290284312 ) ) ;
#31160=CARTESIAN_POINT ( 'NONE',  ( 9.404538367153106648, -79.10366911081999319, 7.521839627124906613 ) ) ;
#31166=CARTESIAN_POINT ( 'NONE',  ( -11.45718701969090070, -76.06302083320471752, -3.078158446385449665 ) ) ;
#31169=CARTESIAN_POINT ( 'NONE',  ( 2.713377469415999776, -77.83421086662899313, -11.74024507335000145 ) ) ;
#31174=CARTESIAN_POINT ( 'NONE',  ( -12.00166164432143923, -76.40995231629973716, -1.570587690725778085 ) ) ;
#31185=ADVANCED_FACE ( 'NONE', ( #40158 ), #58170, .F. ) ;
#31187=CARTESIAN_POINT ( 'NONE',  ( -8.557169117579000783, -77.71168682925997473, -8.383968101560002495 ) ) ;
#31188=CARTESIAN_POINT ( 'NONE',  ( 9.599999999916001059, -87.30000000008399752, -6.531555804621000072E-10 ) ) ;
#31190=CARTESIAN_POINT ( 'NONE',  ( -10.23602166438972638, -76.87166118683381910, 3.794243155524493982 ) ) ;
#31206=CARTESIAN_POINT ( 'NONE',  ( -2.127308605635999772, -78.13598375397499751, -10.70747048031000048 ) ) ;
#31207=CARTESIAN_POINT ( 'NONE',  ( 8.990136242696999958, -78.68304436543799341, 8.365012251980999736 ) ) ;
#31209=CARTESIAN_POINT ( 'NONE',  ( -9.393203674808267678, -79.04166666666665719, -5.413904038987171319 ) ) ;
#31216=CARTESIAN_POINT ( 'NONE',  ( -2.822678701150000080, -79.01742403547800109, 11.58741885751999945 ) ) ;
#31217=CARTESIAN_POINT ( 'NONE',  ( 9.902297125457000249, -80.85282200469704605, -5.173806094917000387 ) ) ;
#31220=CARTESIAN_POINT ( 'NONE',  ( -7.849238557987999521, -76.77212468491599395, 7.706455349885999340 ) ) ;
#31241=( NAMED_UNIT ( * ) PLANE_ANGLE_UNIT ( ) SI_UNIT ( $, .RADIAN. ) );
#31245=CARTESIAN_POINT ( 'NONE',  ( -12.12874067409000034, -76.61293033130499452, 1.606456333463999853 ) ) ;
#31253=CARTESIAN_POINT ( 'NONE',  ( 2.854969924326999919, -78.10452062854089661, 10.84745395575999893 ) ) ;
#31257=CARTESIAN_POINT ( 'NONE',  ( -8.286771986066998608, -78.84283200047998719, 7.559597915363999832 ) ) ;
#31267=CARTESIAN_POINT ( 'NONE',  ( -7.650089724727000551, -76.77316923444898578, -9.607224057717001386 ) ) ;
#31274=EDGE_CURVE ( 'NONE', #28197, #26455, #21347, .T. ) ;
#31281=CARTESIAN_POINT ( 'NONE',  ( -10.86788298907000083, -77.53287430722599538, -5.040355520269000245 ) ) ;
#31284=CARTESIAN_POINT ( 'NONE',  ( -0.08487245167304000026, -78.45215651189698747, 11.93433278878999992 ) ) ;
#31288=CARTESIAN_POINT ( 'NONE',  ( -3.953505135776000046, -79.36303053380299843, 10.29910343295999908 ) ) ;
#31292=CARTESIAN_POINT ( 'NONE',  ( 8.342172210693000522, -79.14070433617399658, 8.687562991252999467 ) ) ;
#31299=CARTESIAN_POINT ( 'NONE',  ( -9.719066392145998989, -76.06110886216698930, -7.489235019707000340 ) ) ;
#31301=CARTESIAN_POINT ( 'NONE',  ( -9.645974121302039350, -76.96251239198622329, 4.906691233381782702 ) ) ;
#31303=CARTESIAN_POINT ( 'NONE',  ( 5.645478026989999343, -79.94337520226639526, -9.744872608167998607 ) ) ;
#31309=CARTESIAN_POINT ( 'NONE',  ( -9.358624512123094874, -76.45833333333334281, 5.407950800604276687 ) ) ;
#31310=FACE_OUTER_BOUND ( 'NONE', #21325, .T. ) ;
#31315=( LENGTH_UNIT ( ) NAMED_UNIT ( * ) SI_UNIT ( .MILLI., .METRE. ) );
#31330=CARTESIAN_POINT ( 'NONE',  ( -9.066796825632000179, -78.74841171265799744, -6.603885667862000375 ) ) ;
#31352=CARTESIAN_POINT ( 'NONE',  ( -5.714083337146000474, -78.85452609989098960, 10.91123161796000041 ) ) ;
#31353=CARTESIAN_POINT ( 'NONE',  ( -10.37257800205000180, -76.67949600664098853, 3.987904220598999405 ) ) ;
#31354=CARTESIAN_POINT ( 'NONE',  ( -6.916021889377625520, -78.03068784888290566, 8.229964326230533089 ) ) ;
#31355=CARTESIAN_POINT ( 'NONE',  ( -5.687706977064000746, -78.04826182971200410, 10.54353137130999940 ) ) ;
#31361=CARTESIAN_POINT ( 'NONE',  ( -7.800315838420999626, -76.82936687607200099, 7.658422569234000221 ) ) ;
#31362=CARTESIAN_POINT ( 'NONE',  ( 7.374560639698954034, -78.12291666666664014, 9.596002108778181494 ) ) ;
#31369=CARTESIAN_POINT ( 'NONE',  ( 7.508079800428999917, -76.88167466538000383, -8.333477563431999968 ) ) ;
#31377=CYLINDRICAL_SURFACE ( 'NONE', #11269, 10.75000000000000000 ) ;
#31382=CARTESIAN_POINT ( 'NONE',  ( -8.674044796698000326, -76.65617272148499239, 6.768505387188000988 ) ) ;
#31388=CARTESIAN_POINT ( 'NONE',  ( -3.353102485753966633, -80.20021897257370824, -10.21483153731809068 ) ) ;
#31391=CARTESIAN_POINT ( 'NONE',  ( 10.89891958939809413, -79.58091136176375358, -2.652387744565959160 ) ) ;
#31394=CARTESIAN_POINT ( 'NONE',  ( 12.00000000000000000, -77.64999999999999147, 0.000000000000000000 ) ) ;
#31396=CARTESIAN_POINT ( 'NONE',  ( 9.317996701405999005, -79.59490324240999826, -6.117968457212000111 ) ) ;
#31401=ORIENTED_EDGE ( 'NONE', *, *, #7408, .F. ) ;
#31406=DIRECTION ( 'NONE',  ( 0.000000000000000000, 0.000000000000000000, -1.000000000000000000 ) ) ;
#31407=CARTESIAN_POINT ( 'NONE',  ( -0.4077927620925000385, -79.26319421340399174, -11.02431129116999919 ) ) ;
#31412=CARTESIAN_POINT ( 'NONE',  ( 10.75000000000000000, -78.35000000000000853, 1.923335087985999915E-14 ) ) ;
#31417=CARTESIAN_POINT ( 'NONE',  ( -4.582365512893316506, -76.99392094393498098, -11.13666644834476038 ) ) ;
#31430=CARTESIAN_POINT ( 'NONE',  ( 10.07210119001000059, -80.55306440022908987, 5.045985883512999592 ) ) ;
#31451=CARTESIAN_POINT ( 'NONE',  ( -1.570796326794884790, -79.01458333333329165, -12.00000000000000355 ) ) ;
#31456=ORIENTED_EDGE ( 'NONE', *, *, #26680, .F. ) ;
#31458=CARTESIAN_POINT ( 'NONE',  ( 7.807927427423821065, -77.28985569457718441, -7.389794798826798683 ) ) ;
#31463=CARTESIAN_POINT ( 'NONE',  ( -5.092641036025000290, -79.61146918641900072, 10.89826376711000044 ) ) ;
#31464=CARTESIAN_POINT ( 'NONE',  ( 2.914848389051019506, -80.35326446144532042, 10.39463640418927248 ) ) ;
#31466=CARTESIAN_POINT ( 'NONE',  ( 11.49150497439000063, -78.85165641916699997, -3.221926464390000078 ) ) ;
#31471=CARTESIAN_POINT ( 'NONE',  ( 11.99957818660027442, -76.64406117551696696, -0.7855671627053041339 ) ) ;
#31476=CYLINDRICAL_SURFACE ( 'NONE', #45030, 12.00000000000000000 ) ;
#31479=DIRECTION ( 'NONE',  ( 0.000000000000000000, 0.000000000000000000, -1.000000000000000000 ) ) ;
#31481=CARTESIAN_POINT ( 'NONE',  ( 6.436424241555000592, -79.92391735373439587, 8.610165096135999008 ) ) ;
#31483=CARTESIAN_POINT ( 'NONE',  ( 11.36821324764999908, -77.87446272180213214, -3.778861202892000559 ) ) ;
#31495=DIRECTION ( 'NONE',  ( 0.000000000000000000, 1.000000000000000000, 0.000000000000000000 ) ) ;
#31500=B_SPLINE_CURVE_WITH_KNOTS ( 'NONE', 3,
 ( #48087, #29463, #25045, #38908, #29745, #34177, #7330, #38330, #47797, #57207, #25331, #25619, #43643, #3201, #16775, #34755, #38624, #12336, #56354, #30325, #7905, #15905, #43068, #2627, #25906, #56641, #43929, #20624, #16199, #2905, #3477, #40060, #35926, #22946, #44497, #45398, #4654, #8777, #35327, #13492, #4049, #36226, #31483, #48650, #18238, #8194, #17338, #54247, #31187, #22051, #546, #40662, #27361, #53652, #13781, #36515, #9075, #49529, #40956, #31782, #49825, #9371, #58076, #22652, #17636 ),
 .UNSPECIFIED., .F., .F.,
 ( 4, 1, 1, 1, 1, 1, 1, 1, 1, 1, 1, 1, 1, 1, 1, 1, 1, 1, 1, 1, 1, 1, 1, 1, 1, 1, 1, 1, 1, 1, 1, 1, 1, 1, 1, 1, 1, 1, 1, 1, 1, 1, 1, 1, 1, 1, 1, 1, 1, 1, 1, 1, 1, 1, 1, 1, 1, 1, 1, 1, 1, 1, 4 ),
 ( 0.000000000000000000, 0.01249978000642217729, 0.02874978733919649962, 0.04499979467197081501, 0.06124980200474514080, 0.07749980933751947354, 0.09374981667029379240, 0.1099998240030681113, 0.1262498313358424162, 0.1424998386686167351, 0.1587498460013910540, 0.1749998533341653728, 0.1912498606669397194, 0.2074998679997140105, 0.2237498753324883571, 0.2399998826652626760, 0.2562498899980369949, 0.2724998973308113137, 0.2887499046635856326, 0.3049999119963599514, 0.3212499193291342703, 0.3374999266619086447, 0.3537499339946829635, 0.3699999413274572269, 0.3862499486602315457, 0.4024999559930059201, 0.4187499633257802389, 0.4349999706585545578, 0.4512499779913288211, 0.4674999853241031955, 0.4837499926568775144, 0.4999999999896518332, 0.5162500073224260966, 0.5325000146552004709, 0.5487500219879747343, 0.5650000293207491087, 0.5812500366535234830, 0.5975000439862977464, 0.6137500513190721207, 0.6300000586518463841, 0.6462500659846207585, 0.6625000733173950218, 0.6787500806501692852, 0.6950000879829436595, 0.7112500953157180339, 0.7275001026484924083, 0.7437501099812666716, 0.7600001173140410460, 0.7762501246468153093, 0.7925001319795895727, 0.8087501393123639470, 0.8250001466451382104, 0.8412501539779126958, 0.8575001613106869591, 0.8737501686434612225, 0.8900001759762355968, 0.9062501833090098602, 0.9225001906417842346, 0.9387501979745584979, 0.9550002053073327613, 0.9712502126401071356, 0.9875002199728815100, 1.000000000000000000 ),
 .UNSPECIFIED. ) ;
#31504=CONICAL_SURFACE ( 'NONE', #51322, 10.29999999990999981, 0.7853981633972997312 ) ;
#31505=CARTESIAN_POINT ( 'NONE',  ( -9.204454400623999888, -78.57176524200400536, -5.869700187727000085 ) ) ;
#31506=CARTESIAN_POINT ( 'NONE',  ( -4.862705500402999981, -78.46600984204799545, -11.27607530993000040 ) ) ;
#31514=CARTESIAN_POINT ( 'NONE',  ( 3.241375870716999508, -80.99271274871159676, 10.69195759319000061 ) ) ;
#31520=CARTESIAN_POINT ( 'NONE',  ( 11.75000000000000000, -79.79999999999999716, -4.009019365174000020E-13 ) ) ;
#31544=CARTESIAN_POINT ( 'NONE',  ( 2.538881527327999876, -76.98177497604999076, 11.96833873699999984 ) ) ;
#31551=CARTESIAN_POINT ( 'NONE',  ( -10.54491486739000017, -77.77768451251904480, -3.823987582478999947 ) ) ;
#31553=CARTESIAN_POINT ( 'NONE',  ( 3.042547531669000271, -78.64783470746900207, -10.31045122763999977 ) ) ;
#31564=CARTESIAN_POINT ( 'NONE',  ( 0.03250568004163000707, -76.07646268326499239, 11.74995503739000036 ) ) ;
#31568=CARTESIAN_POINT ( 'NONE',  ( 9.376438147752001129, -79.45376715878452956, -6.156339679782000474 ) ) ;
#31581=EDGE_CURVE ( 'NONE', #30600, #20755, #33997, .T. ) ;
#31583=CARTESIAN_POINT ( 'NONE',  ( -2.801579282652000291, -79.06343076078299248, -10.67018687299000135 ) ) ;
#31591=CARTESIAN_POINT ( 'NONE',  ( -10.47020627418440242, -77.47916666666667140, 2.813789756862221214 ) ) ;
#31595=CARTESIAN_POINT ( 'NONE',  ( 4.656680505379999779, -76.71804223774499576, 11.60471035503999992 ) ) ;
#31599=CARTESIAN_POINT ( 'NONE',  ( 6.836697942985000331, -79.03132150479699192, 8.804212730688998789 ) ) ;
#31614=COLOUR_RGB ( '', 0.40784314, 0.44705882, 0.49803922) ;
#31617=ORIENTED_EDGE ( 'NONE', *, *, #18449, .T. ) ;
#31620=CARTESIAN_POINT ( 'NONE',  ( -9.512960740429173612, -76.70695994172498899, 5.706843784427905852 ) ) ;
#31623=CARTESIAN_POINT ( 'NONE',  ( 5.176319218327999572, -77.80500231115298959, -9.742045664616000522 ) ) ;
#31628=CARTESIAN_POINT ( 'NONE',  ( -4.152600241220000044, -79.29313857269499977, -10.41988588363999924 ) ) ;
#31629=CARTESIAN_POINT ( 'NONE',  ( 8.826328960311670357, -81.00000000000001421, 6.438658266756784876 ) ) ;
#31631=CARTESIAN_POINT ( 'NONE',  ( -3.708203932498999933, -79.79999999999999716, 11.41267819554000162 ) ) ;
#31640=CYLINDRICAL_SURFACE ( 'NONE', #30859, 10.75000000000000000 ) ;
#31646=CARTESIAN_POINT ( 'NONE',  ( -11.53293850418999966, -79.34293712903799189, 4.645575608415999369 ) ) ;
#31647=CARTESIAN_POINT ( 'NONE',  ( -10.74259976513999959, -76.69405063463399586, 2.023095082799000188 ) ) ;
#31648=CARTESIAN_POINT ( 'NONE',  ( -7.284620157678814323, -78.03426350768698683, 7.905984289670053400 ) ) ;
#31649=CARTESIAN_POINT ( 'NONE',  ( 10.42503750987000011, -77.41068818197000212, -5.902083371034000159 ) ) ;
#31656=CARTESIAN_POINT ( 'NONE',  ( 11.01685767354999967, -77.12896664909099798, -1.698071721886999841 ) ) ;
#31658=CARTESIAN_POINT ( 'NONE',  ( -8.276171816746000331, -80.33277059862079739, 7.458027891273999899 ) ) ;
#31661=VECTOR ( 'NONE', #45718, 1000.000000000000000 ) ;
#31664=CARTESIAN_POINT ( 'NONE',  ( 6.433795189870999742, -77.37192883941298760, -9.188274595716000803 ) ) ;
#31672=DIRECTION ( 'NONE',  ( -1.000000000000000000, 0.000000000000000000, 0.000000000000000000 ) ) ;
#31676=CARTESIAN_POINT ( 'NONE',  ( 5.284336329618000150, -77.94045643997900186, -9.945338310677000138 ) ) ;
#31683=CARTESIAN_POINT ( 'NONE',  ( -5.413904038987160661, -77.08333333333334281, -9.393203674808278336 ) ) ;
#31686=DIRECTION ( 'NONE',  ( 0.000000000000000000, -1.000000000000000000, 0.000000000000000000 ) ) ;
#31687=EDGE_CURVE ( 'NONE', #30430, #1042, #15150, .T. ) ;
#31688=CARTESIAN_POINT ( 'NONE',  ( 11.07171638148000170, -79.13188541137900245, -1.292941197001999942 ) ) ;
#31691=ORIENTED_EDGE ( 'NONE', *, *, #14350, .T. ) ;
#31696=EDGE_LOOP ( 'NONE', ( #19968, #885, #27147, #34230 ) ) ;
#31703=CARTESIAN_POINT ( 'NONE',  ( 5.196088533839524182, -78.26493743760516963, -9.481230459712604031 ) ) ;
#31707=CARTESIAN_POINT ( 'NONE',  ( -1.649952397703835505, -77.01404686049248483, -11.92900123064598361 ) ) ;
#31714=VECTOR ( 'NONE', #334, 1000.000000000000000 ) ;
#31717=CARTESIAN_POINT ( 'NONE',  ( 10.79726974137000006, -76.19359237496099979, -2.097837960889999742 ) ) ;
#31722=CARTESIAN_POINT ( 'NONE',  ( -4.454457568640999732, -80.74124369751984887, 10.34731867136000005 ) ) ;
#31723=CARTESIAN_POINT ( 'NONE',  ( 7.374560639698954034, -76.62291666666664014, 9.596002108778181494 ) ) ;
#31728=CARTESIAN_POINT ( 'NONE',  ( -9.421357847594000745, -80.44786001875249326, -6.176342950743000770 ) ) ;
#31733=DIRECTION ( 'NONE',  ( 0.000000000000000000, -1.000000000000000000, 0.000000000000000000 ) ) ;
#31738=CARTESIAN_POINT ( 'NONE',  ( -9.447769977218822390, -79.56055520885148269, 5.131292296675055375 ) ) ;
#31744=EDGE_CURVE ( 'NONE', #20296, #1042, #18608, .T. ) ;
#31754=CARTESIAN_POINT ( 'NONE',  ( -2.404116552999463696, -77.20721653822319297, -10.47761388392037141 ) ) ;
#31757=AXIS2_PLACEMENT_3D ( 'NONE', #43356, #46945, #56651 ) ;
#31760=CARTESIAN_POINT ( 'NONE',  ( -10.29007107286421885, -76.07604166640594201, -5.929850701927606771 ) ) ;
#31762=CARTESIAN_POINT ( 'NONE',  ( -5.701258714434006336, -80.41929545379491628, 9.167358189660777867 ) ) ;
#31764=ORIENTED_EDGE ( 'NONE', *, *, #53025, .F. ) ;
#31765=CARTESIAN_POINT ( 'NONE',  ( -11.12530226251999999, -78.15976265171399007, 4.628544181647000322 ) ) ;
#31770=CARTESIAN_POINT ( 'NONE',  ( -3.140974612311405512, -78.69583333333332575, 11.68767212001977640 ) ) ;
#31771=CARTESIAN_POINT ( 'NONE',  ( 0.000000000000000000, -87.25000000009099210, 0.000000000000000000 ) ) ;
#31774=B_SPLINE_CURVE_WITH_KNOTS ( 'NONE', 3,
 ( #4977, #42164, #28265, #54580, #10580, #23559, #1155, #9700, #32694, #19141, #37136, #41866, #14120, #54857, #32116, #27689, #46318, #28564 ),
 .UNSPECIFIED., .F., .F.,
 ( 4, 2, 2, 2, 2, 2, 2, 2, 4 ),
 ( 0.000000000000000000, 0.1250000000000000000, 0.2500000000000000000, 0.3750000000000000000, 0.5000000000000000000, 0.6250000000000000000, 0.7500000000000000000, 0.8750000000000000000, 1.000000000000000000 ),
 .UNSPECIFIED. ) ;
#31777=CARTESIAN_POINT ( 'NONE',  ( -11.82602479988079303, -79.79999999999998295, -1.911466474616787536 ) ) ;
#31782=CARTESIAN_POINT ( 'NONE',  ( 11.81379047889000233, -77.41326435959814489, 1.987564636421000008 ) ) ;
#31791=CARTESIAN_POINT ( 'NONE',  ( 3.712057368508056676, -76.26875000000272564, 11.41729714079631819 ) ) ;
#31797=CARTESIAN_POINT ( 'NONE',  ( -5.045247388522612120, -78.18634793776142544, -9.528564678276634226 ) ) ;
#31805=CARTESIAN_POINT ( 'NONE',  ( 9.410240357728000049, -77.31889346392100038, 5.533781925607000218 ) ) ;
#31815=CARTESIAN_POINT ( 'NONE',  ( -11.92598335260000120, -79.12395855886799723, -0.08230123318516001374 ) ) ;
#31816=CARTESIAN_POINT ( 'NONE',  ( -2.537458031822000137, -80.74790394668615079, -10.88048998642999976 ) ) ;
#31817=EDGE_CURVE ( 'NONE', #10196, #26643, #5217, .T. ) ;
#31833=ORIENTED_EDGE ( 'NONE', *, *, #31817, .F. ) ;
#31838=VERTEX_POINT ( 'NONE', #6167 ) ;
#31843=CARTESIAN_POINT ( 'NONE',  ( -1.937110260509999904, -76.80360561063299940, -12.19981367617000068 ) ) ;
#31851=CARTESIAN_POINT ( 'NONE',  ( 9.596002108778172612, -78.99791666666665435, -7.374560639698962028 ) ) ;
#31864=CARTESIAN_POINT ( 'NONE',  ( -6.018890980713000438, -76.11744542156999671, 10.70471907396000155 ) ) ;
#31868=CARTESIAN_POINT ( 'NONE',  ( 10.63562707217000103, -80.02573036182266719, 3.563914325689000240 ) ) ;
#31874=CARTESIAN_POINT ( 'NONE',  ( 4.374544387491000386, -77.15306389129399633, -11.15253550093999912 ) ) ;
#31876=CARTESIAN_POINT ( 'NONE',  ( 11.66178877871000097, -78.34363925020198849, 2.537357863477000208 ) ) ;
#31881=CARTESIAN_POINT ( 'NONE',  ( -7.180765598437999664, -79.39026687680399164, 8.374863569145000852 ) ) ;
#31890=CARTESIAN_POINT ( 'NONE',  ( 10.75000000000000000, -76.75000000000000000, 0.000000000000000000 ) ) ;
#31892=CARTESIAN_POINT ( 'NONE',  ( -2.721343196572999723, -79.67101177224800779, 10.92832355692000057 ) ) ;
#31901=CARTESIAN_POINT ( 'NONE',  ( -5.407950800604208297, -76.41666666666667140, 9.358624512123132178 ) ) ;
#31906=CARTESIAN_POINT ( 'NONE',  ( -2.813789756862300262, -78.39583333333332860, 10.47020627418438465 ) ) ;
#31913=CARTESIAN_POINT ( 'NONE',  ( -4.800187936532999800, -76.16030212922053977, 10.10109298474000106 ) ) ;
#31920=CARTESIAN_POINT ( 'NONE',  ( -0.2291600886666000092, -78.38949755890598681, -11.06898422383999936 ) ) ;
#31931=CARTESIAN_POINT ( 'NONE',  ( -10.48543666025109289, -78.44166666666666288, -6.043427764450796325 ) ) ;
#31933=CARTESIAN_POINT ( 'NONE',  ( 0.000000000000000000, -87.20000000000000284, -9.699999999999976197 ) ) ;
#31940=CARTESIAN_POINT ( 'NONE',  ( 3.529477632267000065, -79.79300913277400298, 11.80040848444000012 ) ) ;
#31941=CARTESIAN_POINT ( 'NONE',  ( 11.23661113560000047, -76.47573121474299285, 2.418095604914000329 ) ) ;
#31942=CARTESIAN_POINT ( 'NONE',  ( -6.653298097564936953, -78.02821361607915662, 8.446342938638746745 ) ) ;
#31943=CARTESIAN_POINT ( 'NONE',  ( -11.61454496413000115, -77.68198133620698798, 2.935712811417999557 ) ) ;
#31947=CARTESIAN_POINT ( 'NONE',  ( 7.768420291617568196, -80.91093204606768552, 7.431500403707722135 ) ) ;
#31950=CARTESIAN_POINT ( 'NONE',  ( 4.249074618647000534, -77.04725762008598622, -10.30533674824999935 ) ) ;
#31951=CARTESIAN_POINT ( 'NONE',  ( -1.570796326794938524, -78.18541666666665435, 11.99999999999999645 ) ) ;
#31952=CARTESIAN_POINT ( 'NONE',  ( 1.917328231603999900, -80.31995460502288608, 10.85776984013000046 ) ) ;
#31953=VERTEX_POINT ( 'NONE', #53352 ) ;
#31955=B_SPLINE_CURVE_WITH_KNOTS ( 'NONE', 3,
 ( #15601, #33877, #46919, #15309, #24462, #19745, #47505, #42474, #15010, #20044, #36352, #54380, #13918, #9499, #10598, #37740, #28583, #46626, #55763, #33302 ),
 .UNSPECIFIED., .F., .F.,
 ( 4, 2, 2, 2, 2, 2, 2, 2, 2, 4 ),
 ( 0.000000000000000000, 0.1250000000000000555, 0.2500000000000001110, 0.3750000000000001665, 0.5000000000000002220, 0.5625000000000002220, 0.6250000000000002220, 0.7500000000000002220, 0.8750000000000001110, 1.000000000000000000 ),
 .UNSPECIFIED. ) ;
#31959=CARTESIAN_POINT ( 'NONE',  ( -2.185791986076000004, -77.80771032744199545, -11.00183730042999919 ) ) ;
#31967=CARTESIAN_POINT ( 'NONE',  ( -10.22919423528282046, -76.04999999999999716, 5.911015989525015613 ) ) ;
#31969=CARTESIAN_POINT ( 'NONE',  ( 11.12204776531999961, -77.46418423053899005, 0.7447510167176000229 ) ) ;
#31976=CARTESIAN_POINT ( 'NONE',  ( -8.864117045829161157, -80.14852009318845205, -6.142631186442469193 ) ) ;
#31982=FACE_OUTER_BOUND ( 'NONE', #42616, .T. ) ;
#31983=CARTESIAN_POINT ( 'NONE',  ( -10.97184146967999929, -79.37701249839500406, 1.968068935562000243 ) ) ;
#31986=VERTEX_POINT ( 'NONE', #25616 ) ;
#32014=CARTESIAN_POINT ( 'NONE',  ( -2.895922040489999905, -80.09400592890570181, 10.88681414971999928 ) ) ;
#32020=DIRECTION ( 'NONE',  ( 1.000000000000000000, 0.000000000000000000, 0.000000000000000000 ) ) ;
#32021=CARTESIAN_POINT ( 'NONE',  ( -9.421357847594000745, -80.38007146547629134, -6.176342950743000770 ) ) ;
#32024=ORIENTED_EDGE ( 'NONE', *, *, #17429, .F. ) ;
#32042=DIRECTION ( 'NONE',  ( 1.000000000000000000, 0.000000000000000000, 0.000000000000000000 ) ) ;
#32044=ADVANCED_FACE ( 'NONE', ( #3199, #21189 ), #57204, .F. ) ;
#32046=CARTESIAN_POINT ( 'NONE',  ( -2.388504738132872340, -77.20733432141381058, -10.48118357590753291 ) ) ;
#32052=DIRECTION ( 'NONE',  ( 0.000000000000000000, -1.000000000000000000, 0.000000000000000000 ) ) ;
#32055=CARTESIAN_POINT ( 'NONE',  ( -1.368150018649999966, -77.80708155120599656, -11.97179757597999838 ) ) ;
#32057=B_SPLINE_SURFACE_WITH_KNOTS ( 'NONE', 3, 3, ( 
 ( #54867, #16895, #14414, #4477, #877, #30734, #22179, #30453, #57907, #50458, #36855, #52907, #53782, #48771, #26023, #26315, #5561, #17461, #53193, #35449, #27988, #32413, #18863, #46037, #8903, #10010, #21884, #35159, #22476, #41294, #44328, #57613, #41585, #53481, #8027, #49058, #44052, #3600, #17173, #8316, #3883, #26895, #39892, #31020, #40187, #8606, #26592, #44628, #4182, #58201, #17764, #35751, #13317, #46620, #47496, #11181, #28278, #33869, #56334, #38022, #56045, #15886, #15594, #55455, #33589, #46329, #37732 ),
 ( #6440, #10591, #32997, #50752, #20034, #5853, #51910, #11470, #28575, #29441, #10297, #6149, #23859, #55756, #51627, #41875, #24158, #51044, #28866, #1452, #7023, #15300, #24454, #42175, #25026, #10889, #1743, #15001, #29157, #46912, #42468, #19446, #19737, #37439, #47206, #6736, #33295, #51332, #1164, #2035, #24742, #42757, #2321, #20317, #38313, #19151, #37147, #55159, #14705, #32704, #48347, #57764, #56910, #48633, #17321, #48071, #21465, #35307, #30307, #30016, #30886, #53050, #25313, #8459, #2608, #17038, #12604 ),
 ( #16465, #38603, #56618, #16177, #34446, #34156, #52195, #12037, #7600, #43620, #3183, #21173, #16756, #34735, #7886, #54804, #44480, #41222, #9354, #27630, #22924, #811, #22036, #22333, #40646, #36783, #49208, #18794, #4924, #13762, #49806, #27341, #40939, #54227, #31765, #35607, #45673, #18502, #14061, #45379, #18218, #526, #22634, #14345, #53939, #26456, #31169, #32055, #32342, #50390, #23214, #58059, #9060, #8759, #4030, #26751, #4330, #40042, #17619, #44780, #36497, #27044, #54524, #53634, #40348, #5212, #58356 ),
 ( #17918, #50099, #13172, #45082, #35907, #13470, #31466, #9643, #49510, #4633, #238, #36209, #10520, #46259, #28503, #20251, #24675, #51554, #38242, #1969, #47136, #6078, #42398, #1099, #55382, #1380, #37662, #14637, #56262, #24084, #15228, #37366, #15814, #19662, #19374, #5786, #19963, #55677, #33220, #32629, #37072, #42102, #14928, #32924, #46552, #37951, #1672, #50683, #42685, #51265, #41514, #10819, #33803, #10225, #55974, #50967, #45966, #28796, #46843, #2250, #15525, #33519, #6371, #24386, #9936, #28203, #6664 ) ),
 .UNSPECIFIED., .F., .F., .F.,
 ( 4, 4 ),
 ( 4, 1, 1, 1, 1, 1, 1, 1, 1, 1, 1, 1, 1, 1, 1, 1, 1, 1, 1, 1, 1, 1, 1, 1, 1, 1, 1, 1, 1, 1, 1, 1, 1, 1, 1, 1, 1, 1, 1, 1, 1, 1, 1, 1, 1, 1, 1, 1, 1, 1, 1, 1, 1, 1, 1, 1, 1, 1, 1, 1, 1, 1, 1, 1, 4 ),
 ( -0.1772706441294000235, 1.177270644128999955 ),
 ( -0.02000000000000000042, -0.003749999999999999861, 0.01250000000000000069, 0.02875000000000000125, 0.04499999999999999833, 0.06124999999999999889, 0.07749999999999999944, 0.09375000000000000000, 0.1100000000000000006, 0.1262500000000000011, 0.1424999999999999878, 0.1587500000000000022, 0.1749999999999999889, 0.1912500000000000033, 0.2074999999999999900, 0.2237500000000000044, 0.2399999999999999911, 0.2562499999999999778, 0.2725000000000000200, 0.2887500000000000067, 0.3049999999999999933, 0.3212499999999999800, 0.3375000000000000222, 0.3537500000000000089, 0.3699999999999999956, 0.3862499999999999822, 0.4025000000000000244, 0.4187500000000000111, 0.4349999999999999978, 0.4512499999999999845, 0.4675000000000000266, 0.4837500000000000133, 0.5000000000000000000, 0.5162499999999999867, 0.5324999999999999734, 0.5487499999999999600, 0.5649999999999999467, 0.5812500000000000444, 0.5975000000000000311, 0.6137500000000000178, 0.6300000000000000044, 0.6462499999999999911, 0.6624999999999999778, 0.6787499999999999645, 0.6949999999999999512, 0.7112500000000000488, 0.7275000000000000355, 0.7437500000000000222, 0.7600000000000000089, 0.7762499999999999956, 0.7924999999999999822, 0.8087499999999999689, 0.8249999999999999556, 0.8412500000000000533, 0.8575000000000000400, 0.8737500000000000266, 0.8900000000000000133, 0.9062500000000000000, 0.9224999999999999867, 0.9387499999999999734, 0.9549999999999999600, 0.9712499999999999467, 0.9875000000000000444, 1.003749999999999920, 1.020000000000000018 ),
 .UNSPECIFIED. ) ;
#32063=CARTESIAN_POINT ( 'NONE',  ( -12.00000000000000000, -78.79999999999999716, 0.000000000000000000 ) ) ;
#32066=VERTEX_POINT ( 'NONE', #9659 ) ;
#32068=EDGE_LOOP ( 'NONE', ( #18953, #53378, #46777, #43112, #40867, #54513, #5156, #22722 ) ) ;
#32071=DIRECTION ( 'NONE',  ( -3.552713678801000121E-14, 1.000000000000000000, 3.403984144012999683E-13 ) ) ;
#32072=CARTESIAN_POINT ( 'NONE',  ( -7.860507001410999450, -76.70312894181100205, 7.955276143908999842 ) ) ;
#32074=ADVANCED_FACE ( 'NONE', ( #45985, #9073 ), #41239, .T. ) ;
#32076=CARTESIAN_POINT ( 'NONE',  ( 8.027846440818999341, -76.63502291188399340, 7.850949632255998623 ) ) ;
#32086=FACE_OUTER_BOUND ( 'NONE', #21466, .T. ) ;
#32100=CARTESIAN_POINT ( 'NONE',  ( -3.634457760627999523, -77.27231996340199771, 11.72972702006000034 ) ) ;
#32107=CARTESIAN_POINT ( 'NONE',  ( 4.140345854158000272, -79.47019575988599627, 11.18451558619000075 ) ) ;
#32108=CARTESIAN_POINT ( 'NONE',  ( -10.60751049107999933, -80.05066853420788675, 3.116614351438999897 ) ) ;
#32111=CARTESIAN_POINT ( 'NONE',  ( -9.998780405325002008, -77.37132423095599165, -5.083552005986999411 ) ) ;
#32116=CARTESIAN_POINT ( 'NONE',  ( -10.01013066307207744, -76.15416666665846890, 4.451642991118897719 ) ) ;
#32124=VERTEX_POINT ( 'NONE', #27358 ) ;
#32125=CIRCLE ( 'NONE', #6692, 11.05000000000000071 ) ;
#32134=DIRECTION ( 'NONE',  ( 1.000000000000000000, 0.000000000000000000, 0.000000000000000000 ) ) ;
#32158=CARTESIAN_POINT ( 'NONE',  ( 2.039250879084999912, -79.88954864681358004, -11.02993955029000084 ) ) ;
#32166=CARTESIAN_POINT ( 'NONE',  ( -10.82689242272999941, -77.61114773376000642, -5.021344731552000340 ) ) ;
#32169=CARTESIAN_POINT ( 'NONE',  ( 9.125560752801000319, -79.73035737123599631, -5.991619725684000031 ) ) ;
#32178=CARTESIAN_POINT ( 'NONE',  ( 9.441578396167999543, -76.68030949943998564, 8.198205470971000608 ) ) ;
#32184=CARTESIAN_POINT ( 'NONE',  ( 5.828547835402000388, -78.37764927275399884, -9.501726143737000640 ) ) ;
#32186=CARTESIAN_POINT ( 'NONE',  ( -7.763928192766062608, -79.61790123138683839, -8.933202951673855807 ) ) ;
#32196=CARTESIAN_POINT ( 'NONE',  ( 1.570796326794857478, -77.16458333333332575, 12.00000000000000533 ) ) ;
#32201=CARTESIAN_POINT ( 'NONE',  ( 8.337885974442610149, -78.79578023353073490, -6.785440158440498415 ) ) ;
#32202=B_SPLINE_CURVE_WITH_KNOTS ( 'NONE', 3,
 ( #23735, #754, #28148, #46788, #10171, #46200, #5725, #19026, #50910, #19602, #45904, #18733, #10458, #46494, #50326, #41456, #54463, #40875 ),
 .UNSPECIFIED., .F., .F.,
 ( 4, 2, 2, 2, 2, 2, 2, 2, 4 ),
 ( 0.000000000000000000, 0.1250000000000000000, 0.2499999999999999722, 0.3750000000000000000, 0.5000000000000000000, 0.6250000000000000000, 0.7500000000000000000, 0.8750000000000000000, 1.000000000000000000 ),
 .UNSPECIFIED. ) ;
#32204=CARTESIAN_POINT ( 'NONE',  ( -1.660522255173999984, -76.63685902701352859, 11.05968181062000077 ) ) ;
#32208=CARTESIAN_POINT ( 'NONE',  ( -8.557286188203086397, -77.61159000152036924, -8.384082802621019681 ) ) ;
#32209=CARTESIAN_POINT ( 'NONE',  ( 5.622824352109999424, -80.00067888228510071, -9.705769245306999693 ) ) ;
#32221=CARTESIAN_POINT ( 'NONE',  ( -10.75000000000000355, -80.98958333333331439, 1.407171709420384609 ) ) ;
#32230=CARTESIAN_POINT ( 'NONE',  ( 4.696081959528999761, -78.78500883819499734, 11.38644304057999967 ) ) ;
#32231=CARTESIAN_POINT ( 'NONE',  ( 10.73633472751000006, -76.36434026635200212, -3.758393515045000299 ) ) ;
#32232=CARTESIAN_POINT ( 'NONE',  ( 9.586126626853495480, -77.88753870104096677, 4.864810896429621501 ) ) ;
#32239=CARTESIAN_POINT ( 'NONE',  ( -2.295071999339000079, -77.78263888113500002, 10.90812747857000176 ) ) ;
#32240=CARTESIAN_POINT ( 'NONE',  ( -3.630949683904999947, -76.04999999999999716, 11.17491406647000041 ) ) ;
#32241=CARTESIAN_POINT ( 'NONE',  ( -8.119375762549999820, -81.01799444111729542, -7.459417917149000488 ) ) ;
#32245=CARTESIAN_POINT ( 'NONE',  ( -7.849238557987999521, -76.63654757836398801, 7.706455349885999340 ) ) ;
#32259=CARTESIAN_POINT ( 'NONE',  ( 9.596002108778145967, -77.60208333333332575, 7.374560639699001996 ) ) ;
#32261=CIRCLE ( 'NONE', #23804, 11.05000000000000071 ) ;
#32263=CARTESIAN_POINT ( 'NONE',  ( -7.599813437125216176, -80.16297796562771794, -7.602572481944763538 ) ) ;
#32269=VECTOR ( 'NONE', #20413, 1000.000000000000000 ) ;
#32270=CARTESIAN_POINT ( 'NONE',  ( -5.360806944915999850, -79.97621204443510123, -9.773246618612999370 ) ) ;
#32277=CARTESIAN_POINT ( 'NONE',  ( 10.75000000000000000, -77.35000000000000853, 0.000000000000000000 ) ) ;
#32286=CARTESIAN_POINT ( 'NONE',  ( 5.246383657897999875, -77.06100733245999379, -10.79237965019999912 ) ) ;
#32297=CARTESIAN_POINT ( 'NONE',  ( 5.620590082324000036, -80.43267365621458964, -9.763102121971000358 ) ) ;
#32303=CARTESIAN_POINT ( 'NONE',  ( 9.579193661067588295, -77.49808761060164386, -7.313663711862211869 ) ) ;
#32314=CARTESIAN_POINT ( 'NONE',  ( -6.658246499064939705, -79.52821171827558544, 8.443780454546217840 ) ) ;
#32337=EDGE_CURVE ( 'NONE', #20296, #54955, #12322, .T. ) ;
#32342=CARTESIAN_POINT ( 'NONE',  ( -5.292199200464000164, -77.77995223578199102, -10.82535908394999957 ) ) ;
#32343=AXIS2_PLACEMENT_3D ( 'NONE', #56370, #48100, #37772 ) ;
#32353=ORIENTED_EDGE ( 'NONE', *, *, #15329, .T. ) ;
#32356=CARTESIAN_POINT ( 'NONE',  ( -9.393203674808267678, -80.54166666666665719, -5.413904038987171319 ) ) ;
#32358=CARTESIAN_POINT ( 'NONE',  ( -11.87945358116625094, -79.79999999999999716, -1.588021400056299548 ) ) ;
#32362=CARTESIAN_POINT ( 'NONE',  ( -10.67244467921999984, -76.74493217846000448, 2.904229794498999873 ) ) ;
#32375=CARTESIAN_POINT ( 'NONE',  ( -11.95950202284999975, -79.14141539787040358, 1.295167635372999948 ) ) ;
#32394=CARTESIAN_POINT ( 'NONE',  ( 3.309015450773000300, -81.12816687753750955, 10.91507257597000091 ) ) ;
#32397=CARTESIAN_POINT ( 'NONE',  ( -7.712695008784000272, -77.46634912723399680, -8.144473358846001432 ) ) ;
#32401=CARTESIAN_POINT ( 'NONE',  ( 7.909611445628718762, -79.80000000000001137, -8.777180137641350299 ) ) ;
#32404=CONICAL_SURFACE ( 'NONE', #39954, 11.84999999993000053, 0.7853981633972997312 ) ;
#32405=DIRECTION ( 'NONE',  ( 0.000000000000000000, 1.000000000000000000, 0.000000000000000000 ) ) ;
#32412=ORIENTED_EDGE ( 'NONE', *, *, #39411, .F. ) ;
#32413=CARTESIAN_POINT ( 'NONE',  ( 7.671012283914000029, -78.64789788104899060, 9.589126640163000204 ) ) ;
#32423=DIRECTION ( 'NONE',  ( 0.000000000000000000, 1.000000000000000000, 0.000000000000000000 ) ) ;
#32436=CARTESIAN_POINT ( 'NONE',  ( -2.813789756862251856, -77.60416666666665719, -10.47020627418439709 ) ) ;
#32441=CARTESIAN_POINT ( 'NONE',  ( 9.406806676749999596, -76.89611744936398452, -7.895227358184000899 ) ) ;
#32446=CARTESIAN_POINT ( 'NONE',  ( 3.371435477143000181, -79.39929447278066732, -10.69820234502000034 ) ) ;
#32453=CARTESIAN_POINT ( 'NONE',  ( 10.42985624311000059, -77.36698389494598871, 5.801172517007000096 ) ) ;
#32456=CARTESIAN_POINT ( 'NONE',  ( 3.535142739574999915, -80.37495082227849252, 10.17871189313000002 ) ) ;
#32462=CARTESIAN_POINT ( 'NONE',  ( 12.00000000000000000, -78.64999999999999147, 0.000000000000000000 ) ) ;
#32465=CARTESIAN_POINT ( 'NONE',  ( 8.400975614893999577, -76.18978390147600521, 9.261618890420999506 ) ) ;
#32470=CARTESIAN_POINT ( 'NONE',  ( 2.165712778014000417, -78.56830367376599611, 10.93454565734000106 ) ) ;
#32472=CARTESIAN_POINT ( 'NONE',  ( -10.75000000000000355, -79.98958333333332860, 1.407171709420384609 ) ) ;
#32482=CARTESIAN_POINT ( 'NONE',  ( 2.813789756862229652, -79.35416666666667140, 10.47020627418440064 ) ) ;
#32484=CARTESIAN_POINT ( 'NONE',  ( -7.374560639699022424, -77.22708333333333997, 9.596002108778135309 ) ) ;
#32489=CARTESIAN_POINT ( 'NONE',  ( 8.939664771278220456, -78.80329824956528739, -5.970164743213411285 ) ) ;
#32495=CARTESIAN_POINT ( 'NONE',  ( 7.919950863376441497, -77.36742616270637996, 8.988568817287896806 ) ) ;
#32496=CARTESIAN_POINT ( 'NONE',  ( -8.382198119002001846, -79.89173351027790204, -7.453647783897999979 ) ) ;
#32497=CARTESIAN_POINT ( 'NONE',  ( 4.889518234483114512, -81.00000000000000000, 9.699724439954369615 ) ) ;
#32518=CARTESIAN_POINT ( 'NONE',  ( 1.533663219811999934, -76.20928543398198940, -11.15151220388999853 ) ) ;
#32519=CARTESIAN_POINT ( 'NONE',  ( 10.28683214875539953, -77.87376456324562923, 3.156758843427483363 ) ) ;
#32520=CARTESIAN_POINT ( 'NONE',  ( -8.557169117579000783, -77.69558072920298741, -8.383968101560000719 ) ) ;
#32526=CARTESIAN_POINT ( 'NONE',  ( 1.672085670906209298, -80.96293633418511604, 10.61893514166530927 ) ) ;
#32527=DIRECTION ( 'NONE',  ( 0.9999813732757145690, 0.000000000000000000, -0.006103531896856088240 ) ) ;
#32529=CARTESIAN_POINT ( 'NONE',  ( 9.087383623426001478, -77.59198448012199378, -6.455544860934000262 ) ) ;
#32530=CARTESIAN_POINT ( 'NONE',  ( 11.61133755414000035, -76.92639651314304672, 3.999933378912999604 ) ) ;
#32531=CARTESIAN_POINT ( 'NONE',  ( 10.99151865632000025, -80.62809514466069061, -1.817614465157000092 ) ) ;
#32535=CARTESIAN_POINT ( 'NONE',  ( 8.196653188619999142, -77.50811055442200370, 7.657217973713000170 ) ) ;
#32538=CARTESIAN_POINT ( 'NONE',  ( -10.31401527466070256, -76.78841872786956912, 3.823154250450220282 ) ) ;
#32558=CARTESIAN_POINT ( 'NONE',  ( -11.02198032011999906, -79.96223007984259823, -0.4665663988222000236 ) ) ;
#32564=EDGE_CURVE ( 'NONE', #53569, #51194, #8638, .T. ) ;
#32578=CARTESIAN_POINT ( 'NONE',  ( 3.370554742410903248, -77.04759005475500544, -11.56126178251549241 ) ) ;
#32591=CARTESIAN_POINT ( 'NONE',  ( -10.58783149161999937, -80.79384588825814717, -3.847989116766000084 ) ) ;
#32592=CARTESIAN_POINT ( 'NONE',  ( -11.68767212001979594, -76.77916666666666856, 3.140974612311315806 ) ) ;
#32593=CARTESIAN_POINT ( 'NONE',  ( 10.75000000000000000, -76.85000000000000853, 0.000000000000000000 ) ) ;
#32609=CARTESIAN_POINT ( 'NONE',  ( 7.575877328000173883, -79.41276128209595697, 7.626825700000964048 ) ) ;
#32621=CARTESIAN_POINT ( 'NONE',  ( -7.589549450764452310, -77.16263193562646450, -7.613205801859955990 ) ) ;
#32625=CARTESIAN_POINT ( 'NONE',  ( 11.77452260639999970, -79.82453443975478535, 1.259536412044000020 ) ) ;
#32629=CARTESIAN_POINT ( 'NONE',  ( 6.013200962235000446, -77.95638901018298839, 10.30906962990999887 ) ) ;
#32634=CARTESIAN_POINT ( 'NONE',  ( -10.47020627418440242, -78.97916666666667140, 2.813789756862221214 ) ) ;
#32643=CARTESIAN_POINT ( 'NONE',  ( -2.813789756862251856, -80.60416666666665719, -10.47020627418439709 ) ) ;
#32648=CARTESIAN_POINT ( 'NONE',  ( 11.01994305158000031, -76.43468485262199863, -1.906499110313000234 ) ) ;
#32659=DIRECTION ( 'NONE',  ( 0.000000000000000000, -1.000000000000000000, 0.000000000000000000 ) ) ;
#32661=CYLINDRICAL_SURFACE ( 'NONE', #42701, 12.00000000000000000 ) ;
#32680=AXIS2_PLACEMENT_3D ( 'NONE', #41651, #14770, #54933 ) ;
#32684=CARTESIAN_POINT ( 'NONE',  ( -2.563933300740000032, -80.81563101109908587, -10.99401458260000020 ) ) ;
#32688=CARTESIAN_POINT ( 'NONE',  ( -9.302864017704999711, -76.94885861019999140, -6.266965030821000759 ) ) ;
#32694=CARTESIAN_POINT ( 'NONE',  ( -2.292169028871041903, -76.10729166666139633, 10.76107357871677550 ) ) ;
#32695=ORIENTED_EDGE ( 'NONE', *, *, #31687, .F. ) ;
#32698=CARTESIAN_POINT ( 'NONE',  ( -0.3187246912203000049, -80.57556890496380220, 11.26088853021000169 ) ) ;
#32704=CARTESIAN_POINT ( 'NONE',  ( -8.689305806348999184, -77.82054998477100582, -8.513430283325000403 ) ) ;
#32712=CARTESIAN_POINT ( 'NONE',  ( 0.000000000000000000, -87.20000000000000284, 0.000000000000000000 ) ) ;
#32732=CARTESIAN_POINT ( 'NONE',  ( -10.85634995915000012, -76.10481652993199475, -5.741293403527000017 ) ) ;
#32737=CARTESIAN_POINT ( 'NONE',  ( 9.453938376997999882, -79.04522201375752388, 6.036651369377000087 ) ) ;
#32745=CARTESIAN_POINT ( 'NONE',  ( 11.76923221829999910, -77.33985457952199738, 1.980068107414000300 ) ) ;
#32749=CARTESIAN_POINT ( 'NONE',  ( -0.2648292726109000017, -79.40352125521398818, 10.91353432424999959 ) ) ;
#32757=CARTESIAN_POINT ( 'NONE',  ( -10.75000000000000000, -77.00000000000000000, 0.000000000000000000 ) ) ;
#32763=CARTESIAN_POINT ( 'NONE',  ( -0.4163023988263999664, -79.39864834222998979, -11.25436168207999899 ) ) ;
#32765=CARTESIAN_POINT ( 'NONE',  ( -8.787981800519466091, -79.60831884209565601, -7.924599827265385699 ) ) ;
#32770=VECTOR ( 'NONE', #37588, 1000.000000000000000 ) ;
#32781=CARTESIAN_POINT ( 'NONE',  ( 5.986666392495521904, -78.77217535623724132, -8.928609192334358013 ) ) ;
#32783=CARTESIAN_POINT ( 'NONE',  ( -7.860507001410999450, -76.68702291099154422, 7.955276143908999842 ) ) ;
#32787=CARTESIAN_POINT ( 'NONE',  ( -11.18443158117183778, -76.51668518724613932, 4.872433950202917252 ) ) ;
#32788=CARTESIAN_POINT ( 'NONE',  ( -4.743944233800447385, -78.64250398762337113, -11.00068109039020747 ) ) ;
#32789=CARTESIAN_POINT ( 'NONE',  ( -10.75729140709000120, -78.78896392293299300, -3.177859684493999914 ) ) ;
#32795=CARTESIAN_POINT ( 'NONE',  ( 0.000000000000000000, -75.15999999999999659, 0.000000000000000000 ) ) ;
#32812=CARTESIAN_POINT ( 'NONE',  ( 9.133850598315257585, -77.89447637907150579, 5.680044527171443036 ) ) ;
#32813=CARTESIAN_POINT ( 'NONE',  ( -10.26943924278000075, -78.52305958491099602, 6.168847710360999770 ) ) ;
#32814=CARTESIAN_POINT ( 'NONE',  ( 0.000000000000000000, -75.15999999999999659, 0.000000000000000000 ) ) ;
#32815=CARTESIAN_POINT ( 'NONE',  ( -6.606735055424326930, -79.02724754890354575, 8.596828543386198618 ) ) ;
#32818=CARTESIAN_POINT ( 'NONE',  ( 8.156436652089588790, -80.90677963425484620, 7.002206209730132080 ) ) ;
#32822=CARTESIAN_POINT ( 'NONE',  ( -10.75275020201999965, -78.47680183458999181, -2.465785609032999925 ) ) ;
#32823=CARTESIAN_POINT ( 'NONE',  ( -8.598496321198998871, -77.21327568127719587, -8.768570137950998600 ) ) ;
#32824=CARTESIAN_POINT ( 'NONE',  ( -9.154119576699001115, -80.84287663268978008, 6.349747989568999884 ) ) ;
#32829=CARTESIAN_POINT ( 'NONE',  ( -11.16975252231999960, -76.75880881764298636, 1.027088271520000040 ) ) ;
#32831=CARTESIAN_POINT ( 'NONE',  ( 6.586108526242999694, -80.17391735373439587, 8.810401493720998900 ) ) ;
#32840=DIRECTION ( 'NONE',  ( 0.8090169943749182524, 0.000000000000000000, 0.5877852522925132162 ) ) ;
#32841=CARTESIAN_POINT ( 'NONE',  ( 3.140974612311377090, -79.44583333333332575, -11.68767212001978528 ) ) ;
#32850=CARTESIAN_POINT ( 'NONE',  ( -9.010285311145000975, -78.94123101036599621, -6.562724981485000164 ) ) ;
#32853=ORIENTED_EDGE ( 'NONE', *, *, #58029, .F. ) ;
#32856=ORIENTED_EDGE ( 'NONE', *, *, #50298, .F. ) ;
#32866=ORIENTED_EDGE ( 'NONE', *, *, #15687, .F. ) ;
#32877=CARTESIAN_POINT ( 'NONE',  ( 3.140974612311326908, -76.75416666666663446, 11.68767212001979772 ) ) ;
#32881=EDGE_CURVE ( 'NONE', #36154, #42760, #5938, .T. ) ;
#32886=CARTESIAN_POINT ( 'NONE',  ( -9.329288041359642847, -76.64178376729412889, -5.387529410381943329 ) ) ;
#32890=CARTESIAN_POINT ( 'NONE',  ( -7.374560639699019760, -78.32708333333330586, 9.596002108778129980 ) ) ;
#32902=CARTESIAN_POINT ( 'NONE',  ( 10.70966587101897183, -79.35754135609677462, 1.004977551424543369 ) ) ;
#32903=CIRCLE ( 'NONE', #11238, 12.50000000000000000 ) ;
#32915=LINE ( 'NONE', #55965, #8693 ) ;
#32919=CARTESIAN_POINT ( 'NONE',  ( 11.77452260639999970, -79.89232299303098728, 1.259536412044000020 ) ) ;
#32924=CARTESIAN_POINT ( 'NONE',  ( 11.32533557775999888, -77.84787174848798941, -3.764608412264000226 ) ) ;
#32928=CARTESIAN_POINT ( 'NONE',  ( -6.606377239730371720, -78.92708333333332860, 8.596418555780411808 ) ) ;
#32936=CARTESIAN_POINT ( 'NONE',  ( -10.75000000000000000, -77.00000000000000000, 0.000000000000000000 ) ) ;
#32942=CARTESIAN_POINT ( 'NONE',  ( -7.434989412783546747, -79.79999999999998295, -9.267694697335807419 ) ) ;
#32944=AXIS2_PLACEMENT_3D ( 'NONE', #24331, #2199, #47368 ) ;
#32946=CARTESIAN_POINT ( 'NONE',  ( 10.12567350656000009, -75.98320989681799631, 4.748118780173999909 ) ) ;
#32952=EDGE_CURVE ( 'NONE', #7885, #14050, #33325, .T. ) ;
#32958=CARTESIAN_POINT ( 'NONE',  ( -10.65912025651878281, -78.08960475230161080, 1.406514330260667078 ) ) ;
#32977=CARTESIAN_POINT ( 'NONE',  ( 6.405550539766999840, -80.53584952307009814, 9.295753483539000328 ) ) ;
#32980=CARTESIAN_POINT ( 'NONE',  ( 7.199825537761999961, -77.22122204021799519, 8.601198917431998936 ) ) ;
#32985=CARTESIAN_POINT ( 'NONE',  ( 10.74305781343810295, -81.00000000000002842, -2.396161594354234481 ) ) ;
#32989=CARTESIAN_POINT ( 'NONE',  ( 8.828526701892000617, -80.39498278894200212, -6.997593314318000246 ) ) ;
#32997=CARTESIAN_POINT ( 'NONE',  ( 5.622631719431000263, -79.09562780968799700, 10.78740717875000144 ) ) ;
#33000=EDGE_LOOP ( 'NONE', ( #58127, #45380, #34165 ) ) ;
#33003=CARTESIAN_POINT ( 'NONE',  ( -10.48543666025111420, -79.75833333333331154, 6.043427764450754580 ) ) ;
#33006=CARTESIAN_POINT ( 'NONE',  ( -0.6644248411249000785, -76.24408568656099305, -12.21661133770999896 ) ) ;
#33015=CARTESIAN_POINT ( 'NONE',  ( -10.64922275351036340, -76.72873637915004963, 2.917915514433102597 ) ) ;
#33028=CARTESIAN_POINT ( 'NONE',  ( 11.61133755414000035, -76.84250581942099245, 3.999933378912999604 ) ) ;
#33032=CARTESIAN_POINT ( 'NONE',  ( 8.645668071321999548, -78.55496783972452590, 7.146365085715999044 ) ) ;
#33036=LINE ( 'NONE', #14458, #37035 ) ;
#33039=CARTESIAN_POINT ( 'NONE',  ( -12.03258451680999919, -78.00461903155100174, 0.6424029262030001020 ) ) ;
#33043=CARTESIAN_POINT ( 'NONE',  ( -10.06651861793999991, -78.99497611018699672, 4.223809761943999597 ) ) ;
#33047=CARTESIAN_POINT ( 'NONE',  ( -11.11223348184000059, -79.79208530464400440, -4.928830210637000775 ) ) ;
#33058=CARTESIAN_POINT ( 'NONE',  ( -11.55240038170842709, -79.56519809028500845, -2.255166230233432323 ) ) ;
#33064=CARTESIAN_POINT ( 'NONE',  ( -4.152657972338684722, -79.44472964675378535, -10.42003074508492233 ) ) ;
#33070=CARTESIAN_POINT ( 'NONE',  ( 10.06780253793347413, -76.09155368262285890, -4.475612946776665879 ) ) ;
#33074=ORIENTED_EDGE ( 'NONE', *, *, #14932, .F. ) ;
#33076=FACE_OUTER_BOUND ( 'NONE', #32068, .T. ) ;
#33077=CARTESIAN_POINT ( 'NONE',  ( 7.286211459007912339, -78.78428004322132949, -7.904517777456380401 ) ) ;
#33085=CARTESIAN_POINT ( 'NONE',  ( 11.36836877616901731, -77.77436589406271139, -3.778912901489055898 ) ) ;
#33086=CARTESIAN_POINT ( 'NONE',  ( 4.653115705712000505, -78.99293419121799786, -10.20620521156999949 ) ) ;
#33104=EDGE_LOOP ( 'NONE', ( #19631, #4491, #12031, #22792 ) ) ;
#33108=CARTESIAN_POINT ( 'NONE',  ( 4.744749809752532244, -77.93878674868346934, 9.646253385772624256 ) ) ;
#33109=CARTESIAN_POINT ( 'NONE',  ( 10.18066396183999878, -78.36028369236800017, 6.314281093748000728 ) ) ;
#33113=CARTESIAN_POINT ( 'NONE',  ( 1.407073214895890878, -78.96473917796927822, 10.74996459197358689 ) ) ;
#33115=CARTESIAN_POINT ( 'NONE',  ( 10.10817968731031513, -80.87791439531011406, 3.669898630734008904 ) ) ;
#33118=CARTESIAN_POINT ( 'NONE',  ( 11.01479880718999915, -78.20443840457200224, -0.6131407820818999266 ) ) ;
#33119=CARTESIAN_POINT ( 'NONE',  ( -3.164411967817999827, -77.25425841958221440, -11.86639179494000018 ) ) ;
#33120=CARTESIAN_POINT ( 'NONE',  ( -10.48974755655999935, -80.54876778545759919, -3.001463441570999979 ) ) ;
#33126=CARTESIAN_POINT ( 'NONE',  ( 7.155101792066000499, -78.51525063703199692, -8.354909834651998324 ) ) ;
#33130=CARTESIAN_POINT ( 'NONE',  ( 6.632299823822999763, -77.18051343188000146, -9.958931470938999553 ) ) ;
#33135=CARTESIAN_POINT ( 'NONE',  ( -11.00476719864000152, -77.25954786493399240, 2.393546210564999832 ) ) ;
#33138=CARTESIAN_POINT ( 'NONE',  ( -1.570796326794938524, -77.68541666666666856, 11.99999999999999645 ) ) ;
#33140=LINE ( 'NONE', #41142, #48769 ) ;
#33147=CARTESIAN_POINT ( 'NONE',  ( -1.463640999337999959, -78.50544952233700258, -10.83301059047000159 ) ) ;
#33152=VERTEX_POINT ( 'NONE', #38107 ) ;
#33194=CARTESIAN_POINT ( 'NONE',  ( 0.6195125560301592005, -79.47047398390786555, 10.74289813788460002 ) ) ;
#33211=EDGE_LOOP ( 'NONE', ( #23264, #45905, #1553, #23801 ) ) ;
#33214=CARTESIAN_POINT ( 'NONE',  ( -10.65106809510000119, -79.16321472370599110, 5.591232889670999739 ) ) ;
#33216=CARTESIAN_POINT ( 'NONE',  ( 0.000000000000000000, -76.00000000000000000, 0.000000000000000000 ) ) ;
#33220=CARTESIAN_POINT ( 'NONE',  ( 2.220279159302000149, -77.98351832560599917, 11.72628939184999908 ) ) ;
#33229=EDGE_CURVE ( 'NONE', #32066, #3688, #7109, .T. ) ;
#33236=CARTESIAN_POINT ( 'NONE',  ( -4.331976239377192783, -79.80000000000002558, -11.03186125555349228 ) ) ;
#33240=CARTESIAN_POINT ( 'NONE',  ( 1.849737152796000039, -76.62788311584399992, 11.02961253862999946 ) ) ;
#33243=CARTESIAN_POINT ( 'NONE',  ( 9.925898951148999672, -76.53469514392799056, -5.249786549701999760 ) ) ;
#33254=CARTESIAN_POINT ( 'NONE',  ( -9.936194076909385942, -78.06890473706415889, 4.102870334978085509 ) ) ;
#33259=CIRCLE ( 'NONE', #43687, 11.70000000000000107 ) ;
#33272=CARTESIAN_POINT ( 'NONE',  ( 11.24487063635999995, -80.46590415106278726, 0.9974943187964001590 ) ) ;
#33276=CARTESIAN_POINT ( 'NONE',  ( 8.282307197233999219, -78.09278501627599667, -7.564489280985000619 ) ) ;
#33277=DIRECTION ( 'NONE',  ( 1.000000000000000000, 0.000000000000000000, 0.000000000000000000 ) ) ;
#33285=CARTESIAN_POINT ( 'NONE',  ( -10.58783149161999937, -80.72605733498191682, -3.847989116766000084 ) ) ;
#33295=CARTESIAN_POINT ( 'NONE',  ( -5.775534476593000122, -78.17323108527999409, 10.70634074252000012 ) ) ;
#33297=CARTESIAN_POINT ( 'NONE',  ( 7.921549804313935184, -78.69040357935692498, -7.357602076918057676 ) ) ;
#33302=CARTESIAN_POINT ( 'NONE',  ( -10.75000000000000000, -77.60000000000000853, 2.252154972635999871E-14 ) ) ;
#33307=CARTESIAN_POINT ( 'NONE',  ( -10.06651861793999991, -78.54179491694800674, 4.223809761943999597 ) ) ;
#33312=LINE ( 'NONE', #10608, #22556 ) ;
#33324=CARTESIAN_POINT ( 'NONE',  ( 8.135116633385999663, -76.95127711100199974, 9.200136113044999675 ) ) ;
#33325=B_SPLINE_CURVE_WITH_KNOTS ( 'NONE', 3,
 ( #6231, #45532, #45827, #5647, #19825, #14210, #36940, #46123, #679, #51128, #27782, #14503, #15088, #28364, #18662, #28662, #41961, #37520, #37229, #41669, #32787, #50540, #9504, #54951, #5940, #10094, #14792, #23073, #50834, #37816, #50248, #55538, #28073, #27491, #10380 ),
 .UNSPECIFIED., .F., .F.,
 ( 4, 1, 1, 1, 1, 1, 1, 1, 1, 1, 1, 1, 1, 1, 1, 1, 1, 1, 1, 1, 1, 1, 1, 1, 1, 1, 1, 1, 1, 1, 1, 1, 4 ),
 ( 0.000000000000000000, 0.01250201779797715899, 0.04500188491171358551, 0.07750175202545862840, 0.1100016191391893078, 0.1425014862529343229, 0.1750013533666937848, 0.2075012204804100591, 0.2400010875941263333, 0.2725009547078425798, 0.3050008218215588540, 0.3375006889354190132, 0.3700005560491352874, 0.4025004231628515616, 0.4350002902765678359, 0.4675001573902841101, 0.5000000245040003843, 0.5324998916178604880, 0.5649997587315768177, 0.5974996258452930364, 0.6299994929590093662, 0.6624993600727255849, 0.6949992271864419147, 0.7274990943001582444, 0.7599989614140183480, 0.7924988285277345668, 0.8249986956414508965, 0.8574985627551672263, 0.8899984298688834450, 0.9224982969825997747, 0.9549981640964599894, 0.9874980312101760971, 1.000000000000000000 ),
 .UNSPECIFIED. ) ;
#33340=CARTESIAN_POINT ( 'NONE',  ( 11.95316821454999889, -78.24878287036499103, -1.522347302216999987 ) ) ;
#33344=CARTESIAN_POINT ( 'NONE',  ( -9.475123589965999571, -79.48523028421899994, 5.421936826000999687 ) ) ;
#33345=CARTESIAN_POINT ( 'NONE',  ( -10.54404894584495800, -79.58452146335964983, 2.093743504281901480 ) ) ;
#33358=CARTESIAN_POINT ( 'NONE',  ( 11.26184072110999779, -78.52708536617198831, 0.07002095171033999310 ) ) ;
#33360=CARTESIAN_POINT ( 'NONE',  ( 5.802455652062412206, -79.21544088115599891, -10.31381048005165013 ) ) ;
#33371=VECTOR ( 'NONE', #2880, 1000.000000000000000 ) ;
#33372=CARTESIAN_POINT ( 'NONE',  ( -12.00000000000000000, -77.29999999999999716, 0.000000000000000000 ) ) ;
#33374=EDGE_LOOP ( 'NONE', ( #520, #16987, #11478, #49557 ) ) ;
#33376=CARTESIAN_POINT ( 'NONE',  ( 9.472593219588741675, -78.81085708764649667, -5.088232997904594157 ) ) ;
#33377=EDGE_CURVE ( 'NONE', #36154, #33872, #26768, .T. ) ;
#33385=CARTESIAN_POINT ( 'NONE',  ( 9.376438147752001129, -79.53766105125399122, -6.156339679782000474 ) ) ;
#33391=CARTESIAN_POINT ( 'NONE',  ( 9.070820421759657748, -78.14995580251232354, 6.598623026053274110 ) ) ;
#33393=CARTESIAN_POINT ( 'NONE',  ( 9.596002108778174389, -77.59791666666664867, -7.374560639698961140 ) ) ;
#33399=CARTESIAN_POINT ( 'NONE',  ( -5.246265831776000255, -79.73908801482100728, -10.82514862071000117 ) ) ;
#33400=AXIS2_PLACEMENT_3D ( 'NONE', #4120, #23519, #22121 ) ;
#33404=CARTESIAN_POINT ( 'NONE',  ( -7.374560639698973574, -79.47291666666666288, -9.596002108778167283 ) ) ;
#33406=CARTESIAN_POINT ( 'NONE',  ( 4.675525028857307142, -77.93936046386056660, 9.679868625465889664 ) ) ;
#33407=CARTESIAN_POINT ( 'NONE',  ( 1.634596122093999959, -78.92999931626700061, 11.63574645295999943 ) ) ;
#33411=CARTESIAN_POINT ( 'NONE',  ( 9.576401669510142156, -80.88767897940253704, 4.883949131846009095 ) ) ;
#33414=CARTESIAN_POINT ( 'NONE',  ( 9.706674989537999565, -77.16945737050299670, -5.242346328414999590 ) ) ;
#33415=CARTESIAN_POINT ( 'NONE',  ( -6.620362748380999918, -76.22968996195905333, -10.34376132320999986 ) ) ;
#33416=CARTESIAN_POINT ( 'NONE',  ( -3.140974612311351777, -78.40416666666665435, -11.68767212001978884 ) ) ;
#33417=VERTEX_POINT ( 'NONE', #11130 ) ;
#33423=CARTESIAN_POINT ( 'NONE',  ( 8.196653188619999142, -77.57589910769799246, 7.657217973713000170 ) ) ;
#33445=CARTESIAN_POINT ( 'NONE',  ( -0.2277317800897999955, -78.51452830333799682, -10.99999347944999961 ) ) ;
#33448=ORIENTED_EDGE ( 'NONE', *, *, #50667, .F. ) ;
#33450=AXIS2_PLACEMENT_3D ( 'NONE', #49324, #26866, #40461 ) ;
#33460=FACE_OUTER_BOUND ( 'NONE', #48418, .T. ) ;
#33466=CARTESIAN_POINT ( 'NONE',  ( 9.576266942516207692, -76.04999999999998295, -5.533717098459915995 ) ) ;
#33470=CARTESIAN_POINT ( 'NONE',  ( -4.582365512893317394, -77.39392094393495825, -11.13666644834475861 ) ) ;
#33482=DIRECTION ( 'NONE',  ( 0.000000000000000000, -1.000000000000000000, 0.000000000000000000 ) ) ;
#33484=EDGE_LOOP ( 'NONE', ( #46335, #10174, #49459, #31764, #38178 ) ) ;
#33496=CARTESIAN_POINT ( 'NONE',  ( -1.485504995112404858, -79.48613549087271224, 10.64710564121015679 ) ) ;
#33499=CARTESIAN_POINT ( 'NONE',  ( 0.000000000000000000, -75.15999999999999659, 0.000000000000000000 ) ) ;
#33509=CARTESIAN_POINT ( 'NONE',  ( 4.415872262643816271, -80.25885311859400417, -9.801209063010123401 ) ) ;
#33515=CARTESIAN_POINT ( 'NONE',  ( 11.90415444617999974, -79.80461201918980407, -1.731350929957999885 ) ) ;
#33519=CARTESIAN_POINT ( 'NONE',  ( 11.75393452337000078, -77.35954407085999662, -2.068948229565000130 ) ) ;
#33531=CARTESIAN_POINT ( 'NONE',  ( 5.413904038987179312, -80.66666666666664298, -9.393203674808262349 ) ) ;
#33533=CARTESIAN_POINT ( 'NONE',  ( -10.78228907302829320, -79.80000000000002558, -5.154748993316502492 ) ) ;
#33534=VECTOR ( 'NONE', #4521, 1000.000000000000000 ) ;
#33538=CARTESIAN_POINT ( 'NONE',  ( -8.075725583014000009, -76.46247691852698836, -7.736700848913999451 ) ) ;
#33541=CARTESIAN_POINT ( 'NONE',  ( 10.99909880189000155, -76.65258609231899811, 1.593564419259000164 ) ) ;
#33548=CARTESIAN_POINT ( 'NONE',  ( 4.687352340516000027, -79.23329064464900284, -11.13768991102999983 ) ) ;
#33549=CARTESIAN_POINT ( 'NONE',  ( -9.933930371580135699, -78.06886005323073618, 4.108349863449450190 ) ) ;
#33566=B_SPLINE_SURFACE_WITH_KNOTS ( 'NONE', 3, 3, ( 
 ( #37726, #42167, #46321, #1735, #28270, #19728, #37429, #55746, #15291, #33285, #37141, #55150, #14696, #55449, #32698, #50746, #14992, #10288, #5846, #23852, #32989, #51035, #10583, #27299, #40892, #36454, #23751, #9894, #772, #14016, #32014, #18463, #50056, #18749, #19333 ),
 ( #49768, #1056, #37034, #483, #13725, #41764, #9602, #55049, #5171, #32591, #50641, #19044, #14597, #27876, #9309, #41471, #46216, #31430, #45334, #27587, #55343, #32297, #14304, #23459, #50344, #41182, #5457, #9019, #23174, #45630, #10188, #28166, #45924, #5743, #1342 ),
 ( #36168, #37327, #49470, #27006, #4884, #45040, #4594, #18175, #22590, #40603, #200, #54481, #54187, #31722, #22881, #36743, #54761, #35273, #35572, #22888, #18181, #36460, #17285, #17585, #35874, #32021, #44445, #8724, #17885, #30849, #40900, #58024, #44745, #45340, #207 ),
 ( #49475, #3997, #48886, #53903, #26717, #49171, #22296, #39720, #4296, #36176, #40313, #45047, #53306, #22599, #50063, #22001, #9316, #58322, #57728, #40610, #54193, #54487, #27309, #18469, #13731, #31728, #14023, #49773, #53599, #4891, #8428, #13434, #9609, #489, #27595 ) ),
 .UNSPECIFIED., .F., .F., .F.,
 ( 4, 4 ),
 ( 4, 1, 1, 1, 1, 1, 1, 1, 1, 1, 1, 1, 1, 1, 1, 1, 1, 1, 1, 1, 1, 1, 1, 1, 1, 1, 1, 1, 1, 1, 1, 1, 4 ),
 ( -0.5168282991433000850, 1.516828299142999992 ),
 ( 0.4364214072047999937, 0.4543785682496999656, 0.4723357292945999930, 0.4902928903395999960, 0.5082500513844999679, 0.5262072124294999709, 0.5441643734743999428, 0.5621215345193999458, 0.5800786955643000287, 0.5980358566093000316, 0.6159930176542000035, 0.6339501786992000065, 0.6519073397440999784, 0.6698645007890999814, 0.6878216618339999533, 0.7057788228789999563, 0.7237359839238999282, 0.7416931449688000111, 0.7596503060138000141, 0.7776074670587000970, 0.7955646281037001000, 0.8135217891486000719, 0.8314789501936000748, 0.8494361112385000467, 0.8673932722835000497, 0.8853504333284000216, 0.9033075943734000246, 0.9212647554182999965, 0.9392219164632999995, 0.9571790775082000824, 0.9751362385532000854, 0.9930933995981000573, 1.011050560643000029 ),
 .UNSPECIFIED. ) ;
#33568=CARTESIAN_POINT ( 'NONE',  ( 9.751903312417001146, -80.50087683706640007, 5.687046010848999522 ) ) ;
#33572=CARTESIAN_POINT ( 'NONE',  ( 0.1392748842281999744, -77.27569472622099056, 11.21600254538999941 ) ) ;
#33578=ORIENTED_EDGE ( 'NONE', *, *, #38191, .T. ) ;
#33583=AXIS2_PLACEMENT_3D ( 'NONE', #22136, #44581, #30694 ) ;
#33589=CARTESIAN_POINT ( 'NONE',  ( 4.484119338316999936, -77.48133731782699840, -11.43188768503999952 ) ) ;
#33591=CARTESIAN_POINT ( 'NONE',  ( -10.74992925859148230, -77.58958685757916385, 1.407065223439301072 ) ) ;
#33592=ORIENTED_EDGE ( 'NONE', *, *, #17943, .T. ) ;
#33599=CARTESIAN_POINT ( 'NONE',  ( -8.157922760392999351, -79.63124863701999345, -7.254216858269000312 ) ) ;
#33614=CARTESIAN_POINT ( 'NONE',  ( 0.000000000000000000, -82.00000000000000000, 0.000000000000000000 ) ) ;
#33616=CARTESIAN_POINT ( 'NONE',  ( 0.03250568004163000707, -76.00867412998898942, 11.74995503739000036 ) ) ;
#33619=CARTESIAN_POINT ( 'NONE',  ( 6.879576957522999692, -79.07245835675909973, 8.859431780707000215 ) ) ;
#33620=CIRCLE ( 'NONE', #35506, 14.00000000000000000 ) ;
#33621=ORIENTED_EDGE ( 'NONE', *, *, #57139, .F. ) ;
#33629=CARTESIAN_POINT ( 'NONE',  ( -11.66523904145000046, -77.96402128256200115, -3.450322983582000180 ) ) ;
#33633=CARTESIAN_POINT ( 'NONE',  ( 5.592013246121999792, -78.85879439517700007, 9.375753510130000024 ) ) ;
#33634=CARTESIAN_POINT ( 'NONE',  ( -10.65756401913684215, -79.58963493226011110, 1.416508826642955521 ) ) ;
#33635=ORIENTED_EDGE ( 'NONE', *, *, #756, .T. ) ;
#33638=ADVANCED_FACE ( 'NONE', ( #35260, #30552 ), #34973, .F. ) ;
#33639=CARTESIAN_POINT ( 'NONE',  ( 6.606377239730313988, -77.32291666666665719, 8.596418555780454440 ) ) ;
#33647=CARTESIAN_POINT ( 'NONE',  ( -8.320158381697998706, -78.71773976718499455, 7.590054615178000397 ) ) ;
#33663=CARTESIAN_POINT ( 'NONE',  ( 8.338887569536000299, -77.14397343098400484, 9.430583988958000319 ) ) ;
#33664=CARTESIAN_POINT ( 'NONE',  ( 2.285767309104500988, -78.74219246598565292, -10.50419463615617488 ) ) ;
#33675=CARTESIAN_POINT ( 'NONE',  ( -11.19989528650999944, -78.82951613320700801, 0.6168112860373000661 ) ) ;
#33681=CARTESIAN_POINT ( 'NONE',  ( 3.895551333537116800, -77.19668379744932452, 10.51885396664144423 ) ) ;
#33684=CARTESIAN_POINT ( 'NONE',  ( 0.000000000000000000, -75.15999999999999659, 0.000000000000000000 ) ) ;
#33685=CARTESIAN_POINT ( 'NONE',  ( 8.596418555780418913, -80.80208333333334281, 6.606377239730356621 ) ) ;
#33692=ORIENTED_EDGE ( 'NONE', *, *, #26215, .F. ) ;
#33693=CARTESIAN_POINT ( 'NONE',  ( 8.871207433088001082, -78.68252314293499694, 8.146610743062000282 ) ) ;
#33695=CARTESIAN_POINT ( 'NONE',  ( 1.407066150998827370, -79.23556352264608904, -10.74982909488969973 ) ) ;
#33696=CARTESIAN_POINT ( 'NONE',  ( 8.770451247185000909, -78.87574068541999850, 8.160602927202999624 ) ) ;
#33701=CARTESIAN_POINT ( 'NONE',  ( 8.164054339978811470, -80.90669609449903987, 6.993313037839142154 ) ) ;
#33704=CARTESIAN_POINT ( 'NONE',  ( -10.94146508061000134, -77.46905714352298844, -1.409282183016999923 ) ) ;
#33705=CARTESIAN_POINT ( 'NONE',  ( -10.06605292056000067, -80.49507241345030195, 4.209295221118999564 ) ) ;
#33713=CARTESIAN_POINT ( 'NONE',  ( -11.21668965365999959, -77.76655350871099870, -0.06311738993059998193 ) ) ;
#33722=ORIENTED_EDGE ( 'NONE', *, *, #53604, .T. ) ;
#33724=CIRCLE ( 'NONE', #14840, 11.05000000000000071 ) ;
#33727=CARTESIAN_POINT ( 'NONE',  ( -3.140974612311351777, -76.90416666666665435, -11.68767212001978884 ) ) ;
#33743=ORIENTED_EDGE ( 'NONE', *, *, #29620, .F. ) ;
#33745=CARTESIAN_POINT ( 'NONE',  ( -6.700596268546000545, -78.14582039176799810, -8.618433365121999756 ) ) ;
#33749=CARTESIAN_POINT ( 'NONE',  ( -1.780884232981000181, -79.81062908972909042, -11.07459082487999957 ) ) ;
#33759=CARTESIAN_POINT ( 'NONE',  ( 1.387435826181647514, -77.43417277704999435, -11.96237581351085844 ) ) ;
#33765=CARTESIAN_POINT ( 'NONE',  ( 2.813981643250826004, -76.74597719254359163, -10.47041296866918891 ) ) ;
#33782=CARTESIAN_POINT ( 'NONE',  ( 1.571200994964738085, -79.46334789937733944, 10.64531129885916094 ) ) ;
#33783=AXIS2_PLACEMENT_3D ( 'NONE', #57718, #48876, #13424 ) ;
#33788=CARTESIAN_POINT ( 'NONE',  ( 10.69210609810000001, -77.98167474757299544, 3.151740433137000252 ) ) ;
#33795=CARTESIAN_POINT ( 'NONE',  ( -10.35486996921426517, -76.19583333330172081, 5.986144667812050457 ) ) ;
#33796=CARTESIAN_POINT ( 'NONE',  ( -3.708203932498999933, -79.79999999999999716, 11.41267819554000162 ) ) ;
#33797=AXIS2_PLACEMENT_3D ( 'NONE', #846, #5247, #37110 ) ;
#33799=CARTESIAN_POINT ( 'NONE',  ( 9.785129497364000173, -79.40228377048700281, -6.997026981537000090 ) ) ;
#33803=CARTESIAN_POINT ( 'NONE',  ( -11.57073820100000106, -77.60370790967400012, 2.924640136927000089 ) ) ;
#33806=CARTESIAN_POINT ( 'NONE',  ( 10.75000000000000000, -78.75000000000000000, 0.000000000000000000 ) ) ;
#33818=CARTESIAN_POINT ( 'NONE',  ( -9.151116546556963272, -79.79999999999999716, -7.636046516761507696 ) ) ;
#33819=CARTESIAN_POINT ( 'NONE',  ( -6.095795872867655341, -80.02337930389114717, 8.857137469015752274 ) ) ;
#33822=CARTESIAN_POINT ( 'NONE',  ( 7.486068761172999686, -76.01845923541398520, -8.059700645992000645 ) ) ;
#33827=CARTESIAN_POINT ( 'NONE',  ( 9.715343368859999273, -76.10078336855899295, -5.397362455191000663 ) ) ;
#33834=CARTESIAN_POINT ( 'NONE',  ( -5.069472984156999651, -79.91866724859939097, 10.81386965974999903 ) ) ;
#33835=CARTESIAN_POINT ( 'NONE',  ( -10.54437012725677647, -78.08449553974310220, 2.092245762801656639 ) ) ;
#33867=CARTESIAN_POINT ( 'NONE',  ( 6.277107794117254613, -78.83005409785420170, 10.03091776325296891 ) ) ;
#33869=CARTESIAN_POINT ( 'NONE',  ( 4.570427068259999892, -77.67124252579399979, 11.39767413300000065 ) ) ;
#33872=VERTEX_POINT ( 'NONE', #13788 ) ;
#33876=ADVANCED_FACE ( 'NONE', ( #32086 ), #45995, .F. ) ;
#33877=CARTESIAN_POINT ( 'NONE',  ( 10.75040930116792204, -77.83963288239696965, -1.407121311787697948 ) ) ;
#33881=CARTESIAN_POINT ( 'NONE',  ( -0.2230286467304000153, -78.19680123892500490, -10.77282081049999896 ) ) ;
#33896=DIRECTION ( 'NONE',  ( 0.000000000000000000, -1.000000000000000000, 0.000000000000000000 ) ) ;
#33898=CARTESIAN_POINT ( 'NONE',  ( 0.03250568004163000707, -75.94088557671300066, 11.74995503739000036 ) ) ;
#33900=FACE_OUTER_BOUND ( 'NONE', #28432, .T. ) ;
#33902=CARTESIAN_POINT ( 'NONE',  ( 10.48543666025110710, -78.00833333333332575, -6.043427764450776785 ) ) ;
#33909=ADVANCED_FACE ( 'NONE', ( #53226 ), #57903, .F. ) ;
#33912=CARTESIAN_POINT ( 'NONE',  ( -11.68231536908000123, -77.48916203849999818, 2.952842578158000109 ) ) ;
#33913=DIRECTION ( 'NONE',  ( 0.000000000000000000, 1.000000000000000000, 0.000000000000000000 ) ) ;
#33916=CARTESIAN_POINT ( 'NONE',  ( -8.824204240651999598, -79.07668513919199427, -6.427191105727000142 ) ) ;
#33917=CARTESIAN_POINT ( 'NONE',  ( -10.03645592992567792, -79.57090332437941527, 3.852638260147155602 ) ) ;
#33929=EDGE_CURVE ( 'NONE', #21876, #41938, #15034, .T. ) ;
#33930=CARTESIAN_POINT ( 'NONE',  ( 10.97564558566000059, -79.04457588320700268, 2.523721168482999655 ) ) ;
#33931=CARTESIAN_POINT ( 'NONE',  ( -4.800269761346773301, -76.26018993196245788, 10.10126516968071719 ) ) ;
#33941=CARTESIAN_POINT ( 'NONE',  ( 10.73640186359711102, -76.13322000874006790, -2.284131902630157196 ) ) ;
#33942=DIRECTION ( 'NONE',  ( 1.000000000000000000, 0.000000000000000000, 0.000000000000000000 ) ) ;
#33947=CARTESIAN_POINT ( 'NONE',  ( 6.829512357978999582, -77.43143009854699699, -9.995615053322000065 ) ) ;
#33948=CARTESIAN_POINT ( 'NONE',  ( -4.666033688610307983, -78.68943876540365068, -9.684451540703740591 ) ) ;
#33952=AXIS2_PLACEMENT_3D ( 'NONE', #49766, #36165, #54185 ) ;
#33957=CARTESIAN_POINT ( 'NONE',  ( -9.393200444579274944, -79.64169496360098321, -5.413760864891401070 ) ) ;
#33959=CARTESIAN_POINT ( 'NONE',  ( 5.137083998358000336, -77.21100733245999947, -10.56753840748999984 ) ) ;
#33960=CARTESIAN_POINT ( 'NONE',  ( 4.782478426736999744, -79.67384276626299311, 10.14623135401999932 ) ) ;
#33968=DIRECTION ( 'NONE',  ( 0.7071067811865474617, -0.7071067811865474617, 4.376097137204291133E-09 ) ) ;
#33982=CARTESIAN_POINT ( 'NONE',  ( -8.596154512980129780, -79.15224688203926462, -6.606175269931966909 ) ) ;
#33983=CARTESIAN_POINT ( 'NONE',  ( -1.360213228908000005, -77.68205080677400076, -11.90234785270000017 ) ) ;
#33985=CARTESIAN_POINT ( 'NONE',  ( 5.413694191244308840, -78.93348499250215866, 9.392869764965404045 ) ) ;
#33987=CARTESIAN_POINT ( 'NONE',  ( 10.74987353692243452, -80.85518448745408193, 0.6718904260645724991 ) ) ;
#33990=CARTESIAN_POINT ( 'NONE',  ( -10.37098203719999923, -77.98654766055700804, -3.760912916518000415 ) ) ;
#33997=B_SPLINE_CURVE_WITH_KNOTS ( 'NONE', 3,
 ( #46996, #51418, #20968, #47287, #52561, #7680, #30098, #43134, #42841, #24824, #43411, #38684, #6815, #56704, #2399, #56416, #15965, #38973, #33957, #10975, #16261, #11549 ),
 .UNSPECIFIED., .F., .F.,
 ( 4, 2, 2, 2, 2, 2, 2, 2, 2, 2, 4 ),
 ( 0.000000000000000000, 0.1250000000000000000, 0.2500000000000000000, 0.3750000000000000000, 0.4375000000000000000, 0.5000000000000000000, 0.5625000000000000000, 0.6250000000000000000, 0.7500000000000000000, 0.8750000000000000000, 1.000000000000000000 ),
 .UNSPECIFIED. ) ;
#34000=CARTESIAN_POINT ( 'NONE',  ( 9.070694317316998934, -78.06615328173100465, 6.598531290616000078 ) ) ;
#34004=CARTESIAN_POINT ( 'NONE',  ( 11.80177567542000006, -76.84575795437399393, 2.898902813627999731 ) ) ;
#34013=CARTESIAN_POINT ( 'NONE',  ( 6.043427764450807871, -76.96666666666666856, -10.48543666025108934 ) ) ;
#34017=DIRECTION ( 'NONE',  ( 1.000000000000000000, 0.000000000000000000, 0.000000000000000000 ) ) ;
#34024=ADVANCED_FACE ( 'NONE', ( #28312 ), #41929, .T. ) ;
#34027=CARTESIAN_POINT ( 'NONE',  ( -1.323062013136505399, -80.99999999999998579, -10.86425420506007633 ) ) ;
#34028=CARTESIAN_POINT ( 'NONE',  ( -10.91657421154000041, -77.57385718872899361, -0.06142861151470999787 ) ) ;
#34049=FACE_OUTER_BOUND ( 'NONE', #33211, .T. ) ;
#34053=ADVANCED_FACE ( 'NONE', ( #54903 ), #34363, .F. ) ;
#34076=CARTESIAN_POINT ( 'NONE',  ( 9.014158510551999015, -78.00891109057499762, 6.557403976990999972 ) ) ;
#34082=CARTESIAN_POINT ( 'NONE',  ( 7.653722864265482428, -80.28804818156974932, -7.548741967642948580 ) ) ;
#34084=CARTESIAN_POINT ( 'NONE',  ( 7.359053403517531677, -80.16684166704409620, 8.232126067569696559 ) ) ;
#34086=CARTESIAN_POINT ( 'NONE',  ( -5.092641036025000290, -79.40810352659100602, 10.89826376711000044 ) ) ;
#34088=CARTESIAN_POINT ( 'NONE',  ( -8.415968974905998934, -79.88124863702039136, -7.483677623529000122 ) ) ;
#34103=CARTESIAN_POINT ( 'NONE',  ( -10.21591591617042205, -80.07484147801372387, 3.346207656172486722 ) ) ;
#34106=CARTESIAN_POINT ( 'NONE',  ( 1.849737152796000039, -76.69567166912000289, 11.02961253862999946 ) ) ;
#34107=CARTESIAN_POINT ( 'NONE',  ( 8.079871975571242260, -76.40862220706031849, 7.134473887754699817 ) ) ;
#34109=CARTESIAN_POINT ( 'NONE',  ( 10.90992603612999901, -76.12586531054799366, -2.119726332427000148 ) ) ;
#34112=CARTESIAN_POINT ( 'NONE',  ( 10.25000000000000000, -87.20000000000000284, 0.000000000000000000 ) ) ;
#34116=CARTESIAN_POINT ( 'NONE',  ( -9.563733257752160100, -78.06231107666935998, 4.912333404894130950 ) ) ;
#34117=EDGE_CURVE ( 'NONE', #29449, #185, #37196, .T. ) ;
#34125=CARTESIAN_POINT ( 'NONE',  ( -7.608356748847191042, -79.22937652759581795, 9.340614718761999669 ) ) ;
#34136=CARTESIAN_POINT ( 'NONE',  ( 11.22355342542000045, -80.50686022575678180, 0.9700744431168999427 ) ) ;
#34144=CARTESIAN_POINT ( 'NONE',  ( 1.455635362263224986, -79.96447437086105481, 10.65250472726658693 ) ) ;
#34152=ADVANCED_FACE ( 'NONE', ( #47958 ), #50969, .F. ) ;
#34155=ORIENTED_EDGE ( 'NONE', *, *, #42080, .F. ) ;
#34156=CARTESIAN_POINT ( 'NONE',  ( 12.02223179210000126, -78.94651279900399743, 0.8134715296432000198 ) ) ;
#34165=ORIENTED_EDGE ( 'NONE', *, *, #44536, .F. ) ;
#34176=CARTESIAN_POINT ( 'NONE',  ( -6.489766492868402459, -80.42572473943350531, -9.141528674627377171 ) ) ;
#34177=CARTESIAN_POINT ( 'NONE',  ( 11.53501176087999980, -78.87824739248154060, -3.234124663588000548 ) ) ;
#34184=CARTESIAN_POINT ( 'NONE',  ( -11.80208112487999905, -77.02061369597500118, -3.396125071686999952 ) ) ;
#34187=CARTESIAN_POINT ( 'NONE',  ( 12.00000000000000000, -78.04999999999999716, 0.000000000000000000 ) ) ;
#34194=CARTESIAN_POINT ( 'NONE',  ( 12.06733228363000165, -78.18105580595199910, -1.536887159723000051 ) ) ;
#34200=ORIENTED_EDGE ( 'NONE', *, *, #11708, .T. ) ;
#34204=CARTESIAN_POINT ( 'NONE',  ( 7.234766560894000165, -79.01412808429699908, 9.437955368358000641 ) ) ;
#34208=DIRECTION ( 'NONE',  ( -3.552713678800000476E-14, -1.000000000000000000, 1.184237892933000067E-14 ) ) ;
#34210=CARTESIAN_POINT ( 'NONE',  ( 9.596002108778174389, -78.09791666666666288, -7.374560639698961140 ) ) ;
#34215=CARTESIAN_POINT ( 'NONE',  ( -10.68477278295909372, -79.01421070604040153, 5.086768384352462036 ) ) ;
#34226=LINE ( 'NONE', #19512, #30199 ) ;
#34230=ORIENTED_EDGE ( 'NONE', *, *, #38692, .T. ) ;
#34231=CARTESIAN_POINT ( 'NONE',  ( -10.67341028599000019, -76.21560886216698805, 6.449573273694999997 ) ) ;
#34232=CARTESIAN_POINT ( 'NONE',  ( -6.557449765169716116, -78.67302949370692033, -8.547667297717341128 ) ) ;
#34243=CARTESIAN_POINT ( 'NONE',  ( 10.12058791103999944, -79.61937008025999774, 4.836508133599999759 ) ) ;
#34252=CARTESIAN_POINT ( 'NONE',  ( -3.633154385059917058, -77.25115648345233410, 10.61234178577903009 ) ) ;
#34257=CARTESIAN_POINT ( 'NONE',  ( 5.413904038987143785, -80.83333333333331439, 9.393203674808290771 ) ) ;
#34264=CARTESIAN_POINT ( 'NONE',  ( 3.630949683904999947, -79.79999999999999716, -11.17491406647000041 ) ) ;
#34271=CARTESIAN_POINT ( 'NONE',  ( 2.228685126279000173, -77.92621464558799005, 11.77068507108999995 ) ) ;
#34277=CARTESIAN_POINT ( 'NONE',  ( -10.59418153559903963, -76.58652079386806122, 1.823743049675861316 ) ) ;
#34278=CARTESIAN_POINT ( 'NONE',  ( -4.522750724863999316, -78.43558352699498926, 9.935798501838000618 ) ) ;
#34279=CARTESIAN_POINT ( 'NONE',  ( 10.76452101003999928, -80.76354927348663182, -1.780076958437000201 ) ) ;
#34288=CARTESIAN_POINT ( 'NONE',  ( -0.9512330062464999791, -78.21565086401200517, 11.17646036812999988 ) ) ;
#34292=CARTESIAN_POINT ( 'NONE',  ( 10.10886165594999930, -76.27976687979999326, -6.745106749100000521 ) ) ;
#34296=CARTESIAN_POINT ( 'NONE',  ( -1.612912635236000147, -78.52781295235500636, 10.91330597072999886 ) ) ;
#34314=ORIENTED_EDGE ( 'NONE', *, *, #48434, .F. ) ;
#34316=CARTESIAN_POINT ( 'NONE',  ( -10.43309661003928035, -81.00000000000001421, -2.732452926732640730 ) ) ;
#34317=CARTESIAN_POINT ( 'NONE',  ( 6.963658808075999573, -78.25476576377499782, -8.131364605499999954 ) ) ;
#34332=CARTESIAN_POINT ( 'NONE',  ( -10.75000000000000000, -76.50000000000000000, 0.000000000000000000 ) ) ;
#34339=CARTESIAN_POINT ( 'NONE',  ( -6.777984382448000389, -78.27882627552999395, -9.878005474088999094 ) ) ;
#34345=CARTESIAN_POINT ( 'NONE',  ( -8.684735281668000795, -77.87832987473298374, -7.170030519161000093 ) ) ;
#34356=CARTESIAN_POINT ( 'NONE',  ( -8.547463563348092208, -77.04807323675491659, 6.557389287125792166 ) ) ;
#34363=CONICAL_SURFACE ( 'NONE', #41002, 10.90000000000000036, 0.7853981633972997312 ) ;
#34366=CARTESIAN_POINT ( 'NONE',  ( 1.499018853861999956, -77.57312960254600398, 11.04570246958999924 ) ) ;
#34372=CARTESIAN_POINT ( 'NONE',  ( 10.75000000000000000, -77.85000000000000853, 0.000000000000000000 ) ) ;
#34373=CARTESIAN_POINT ( 'NONE',  ( 5.978428684135045579, -80.27239524385058189, -8.933915976532038172 ) ) ;
#34374=CARTESIAN_POINT ( 'NONE',  ( -8.859283645363305482, -76.15416666664359013, 7.973755076573407763 ) ) ;
#34375=CARTESIAN_POINT ( 'NONE',  ( 6.586108526242999694, -80.17391735373439587, 8.810401493720998900 ) ) ;
#34377=CARTESIAN_POINT ( 'NONE',  ( 2.377756013412999803, -79.20693940223900142, -11.79209151100000064 ) ) ;
#34380=FACE_OUTER_BOUND ( 'NONE', #56049, .T. ) ;
#34394=EDGE_LOOP ( 'NONE', ( #48643, #10923, #48849, #41735, #39346, #40477, #29437, #32695, #15529, #29170, #39182 ) ) ;
#34401=CARTESIAN_POINT ( 'NONE',  ( -7.860507001410999450, -76.77091749508699081, 7.955276143908999842 ) ) ;
#34406=CARTESIAN_POINT ( 'NONE',  ( -7.730852068515999598, -76.89588675065598977, 7.824058043802000206 ) ) ;
#34412=CARTESIAN_POINT ( 'NONE',  ( -4.175974021636958078, -78.00676210295078761, 9.905762318292611113 ) ) ;
#34417=CARTESIAN_POINT ( 'NONE',  ( 10.48543666025108045, -79.19166666666664867, 6.043427764450817641 ) ) ;
#34428=CARTESIAN_POINT ( 'NONE',  ( 3.862060628231000159, -80.59715328376763921, 10.58270681924999934 ) ) ;
#34429=CARTESIAN_POINT ( 'NONE',  ( -11.27112434177000111, -80.28882241345029058, -1.746253588004999857 ) ) ;
#34436=CARTESIAN_POINT ( 'NONE',  ( 4.234904783647084336, -79.94291063207141690, 9.880592056022285519 ) ) ;
#34446=CARTESIAN_POINT ( 'NONE',  ( 11.05834404496999923, -78.97364211442699400, 4.786306364259000468 ) ) ;
#34449=ORIENTED_EDGE ( 'NONE', *, *, #17014, .T. ) ;
#34457=ORIENTED_EDGE ( 'NONE', *, *, #2994, .T. ) ;
#34473=CARTESIAN_POINT ( 'NONE',  ( -1.925872869407999843, -76.61078631292498642, -12.12904120624999926 ) ) ;
#34485=CARTESIAN_POINT ( 'NONE',  ( 9.289757862025998847, -77.74698675917198898, 7.853848066408001038 ) ) ;
#34490=CARTESIAN_POINT ( 'NONE',  ( -10.63482758102835746, -79.58845129605020929, 1.575059985258391526 ) ) ;
#34494=CARTESIAN_POINT ( 'NONE',  ( 5.873650711053000073, -79.85752639446890555, -10.25566215449000040 ) ) ;
#34502=EDGE_LOOP ( 'NONE', ( #52270, #47916, #19311, #40510 ) ) ;
#34504=CARTESIAN_POINT ( 'NONE',  ( -11.32256795663581883, -79.07170504178779424, -3.221356905262933168 ) ) ;
#34514=CARTESIAN_POINT ( 'NONE',  ( -5.414043966650280204, -78.51670080977129373, 9.393383066539517046 ) ) ;
#34518=CARTESIAN_POINT ( 'NONE',  ( -1.974112733099000039, -76.93905973945899746, -12.43285320951000017 ) ) ;
#34519=CARTESIAN_POINT ( 'NONE',  ( 2.133450394463557664, -78.74103176239034951, -10.53608711097416162 ) ) ;
#34531=CARTESIAN_POINT ( 'NONE',  ( 0.9578316561262000262, -79.03348640149199866, -11.17589679220000143 ) ) ;
#34554=DIRECTION ( 'NONE',  ( 0.000000000000000000, 0.000000000000000000, -1.000000000000000000 ) ) ;
#34559=CARTESIAN_POINT ( 'NONE',  ( 9.450487096927000508, -77.76343875304499420, -7.362360902974999455 ) ) ;
#34560=CARTESIAN_POINT ( 'NONE',  ( 0.000000000000000000, -81.00000000000000000, 0.000000000000000000 ) ) ;
#34572=CARTESIAN_POINT ( 'NONE',  ( 7.372964296364999726, -79.14958221312299713, 9.618238180306001084 ) ) ;
#34573=CARTESIAN_POINT ( 'NONE',  ( 0.000000000000000000, -87.70000000000000284, 0.000000000000000000 ) ) ;
#34579=CARTESIAN_POINT ( 'NONE',  ( -5.227273583242999067, -76.09884160047198520, -11.10057349953000028 ) ) ;
#34584=CARTESIAN_POINT ( 'NONE',  ( -5.182070223403000497, -78.55504929535699432, 9.738987759633999985 ) ) ;
#34591=CARTESIAN_POINT ( 'NONE',  ( 11.68767212001979594, -79.52916666666665435, -3.140974612311341563 ) ) ;
#34603=ORIENTED_EDGE ( 'NONE', *, *, #10602, .F. ) ;
#34606=CARTESIAN_POINT ( 'NONE',  ( -8.496131438301000927, -77.51938450272599823, 6.855006679309999740 ) ) ;
#34610=CARTESIAN_POINT ( 'NONE',  ( -10.71602610194999805, -79.67444737472000327, 3.314346869870000489 ) ) ;
#34629=CARTESIAN_POINT ( 'NONE',  ( 3.925078296951999501, -78.55011942976800299, 11.31856107452000160 ) ) ;
#34636=CARTESIAN_POINT ( 'NONE',  ( -7.743768518152000624, -77.38807570069999997, -8.177286450628999503 ) ) ;
#34654=CARTESIAN_POINT ( 'NONE',  ( -10.52129323452999898, -77.68207497455300370, 3.681981700656000278 ) ) ;
#34660=CARTESIAN_POINT ( 'NONE',  ( -2.486379155175535871, -80.20678445994957428, -10.46580476966082962 ) ) ;
#34666=CARTESIAN_POINT ( 'NONE',  ( -6.349996674360999904, -78.90074028895499225, -9.301156207373001195 ) ) ;
#34668=CARTESIAN_POINT ( 'NONE',  ( 10.75041758345825649, -77.36048236442238135, 1.407139100108084406 ) ) ;
#34687=CARTESIAN_POINT ( 'NONE',  ( -8.506113518985836564, -80.04778286667620080, 6.573857701660976716 ) ) ;
#34690=CARTESIAN_POINT ( 'NONE',  ( 9.776276929627000456, -76.04354117740300012, -5.431214116490000521 ) ) ;
#34693=CARTESIAN_POINT ( 'NONE',  ( 9.723003665007999174, -76.67014927275398861, -5.142475670412999911 ) ) ;
#34701=CARTESIAN_POINT ( 'NONE',  ( 0.9986783041480190581, -80.96805384704971686, 10.70471205834406625 ) ) ;
#34706=CARTESIAN_POINT ( 'NONE',  ( -10.87922314793346423, -79.26468826379790755, 5.174618772388034138 ) ) ;
#34711=CIRCLE ( 'NONE', #33797, 12.09999999999999964 ) ;
#34715=CARTESIAN_POINT ( 'NONE',  ( 6.985849709488999970, -80.92822782980758234, -8.837815942395002011 ) ) ;
#34719=CARTESIAN_POINT ( 'NONE',  ( -12.00000000000000000, -78.89999999999999147, -1.868256502752000067E-14 ) ) ;
#34722=CARTESIAN_POINT ( 'NONE',  ( 4.235425280252315794, -79.94290626548179546, 9.880369340961230762 ) ) ;
#34726=CARTESIAN_POINT ( 'NONE',  ( 9.898965768568219303, -77.31804819846105659, -4.223239295616174616 ) ) ;
#34735=CARTESIAN_POINT ( 'NONE',  ( -10.67791114319000023, -78.72947827561399947, -5.583725037239000599 ) ) ;
#34740=B_SPLINE_CURVE_WITH_KNOTS ( 'NONE', 3,
 ( #16231, #11232, #57243, #43105, #34210, #56388, #34792, #52247, #38366, #24797, #20939, #11804, #25365, #42811, #56102, #2663, #47554, #15938 ),
 .UNSPECIFIED., .F., .F.,
 ( 4, 2, 2, 2, 2, 2, 2, 2, 4 ),
 ( 0.000000000000000000, 0.1250000000000000000, 0.2500000000000000000, 0.3750000000000000000, 0.5000000000000000000, 0.6250000000000000000, 0.7500000000000000000, 0.8750000000000000000, 1.000000000000000000 ),
 .UNSPECIFIED. ) ;
#34745=VERTEX_POINT ( 'NONE', #28403 ) ;
#34747=CARTESIAN_POINT ( 'NONE',  ( -3.463460669170729478, -80.69899254569148184, -10.20046286209545983 ) ) ;
#34755=CARTESIAN_POINT ( 'NONE',  ( -10.26943924278000075, -78.60695423824412842, 6.168847710361000658 ) ) ;
#34757=CARTESIAN_POINT ( 'NONE',  ( 5.246383657897999875, -77.46100733245999947, -10.79237965019999912 ) ) ;
#34759=ADVANCED_FACE ( 'NONE', ( #8586 ), #37275, .F. ) ;
#34764=CARTESIAN_POINT ( 'NONE',  ( -10.85634995915000012, -76.03702797665600599, -5.741293403527000017 ) ) ;
#34775=CARTESIAN_POINT ( 'NONE',  ( 10.96171043400000045, -78.08619942611500164, -5.535041421897999747 ) ) ;
#34780=CARTESIAN_POINT ( 'NONE',  ( 9.599999999999999645, -87.59999999999999432, 0.000000000000000000 ) ) ;
#34782=CARTESIAN_POINT ( 'NONE',  ( -4.927957436858316775, -79.51302443800736341, 9.553899519113622674 ) ) ;
#34785=CARTESIAN_POINT ( 'NONE',  ( 8.459138740827000902, -79.37812103921298501, -8.569435492024000567 ) ) ;
#34792=CARTESIAN_POINT ( 'NONE',  ( 6.043427764450807871, -78.06666666666666288, -10.48543666025108756 ) ) ;
#34795=CARTESIAN_POINT ( 'NONE',  ( 3.042547531669000271, -78.64783470746900207, -10.31045122763999977 ) ) ;
#34811=CARTESIAN_POINT ( 'NONE',  ( -9.952602430950999945, -76.70740172182600247, 7.514132727938000578 ) ) ;
#34812=CARTESIAN_POINT ( 'NONE',  ( 2.106029303673160324, -78.74082198396830279, -10.54159598279656329 ) ) ;
#34819=CARTESIAN_POINT ( 'NONE',  ( 6.433795189870999742, -77.42361205349585873, -9.188274595716000803 ) ) ;
#34822=CARTESIAN_POINT ( 'NONE',  ( -9.735611069857000643, -79.36032251751400679, 5.570995215215999607 ) ) ;
#34831=CIRCLE ( 'NONE', #48103, 9.599999999999999645 ) ;
#34840=CARTESIAN_POINT ( 'NONE',  ( 9.393203674808260573, -77.79166666666665719, 5.413904038987188194 ) ) ;
#34845=CARTESIAN_POINT ( 'NONE',  ( -10.61596739836999959, -78.53665897790600070, -5.551333230057999835 ) ) ;
#34858=CARTESIAN_POINT ( 'NONE',  ( -6.516581675540000340, -79.40704064464900114, -10.39800818482999922 ) ) ;
#34862=CARTESIAN_POINT ( 'NONE',  ( 1.508420534579999917, -77.69816034697798557, 11.11497989572000122 ) ) ;
#34865=CARTESIAN_POINT ( 'NONE',  ( 0.4178879169752000022, -76.13657433877699532, -12.26266848588000080 ) ) ;
#34869=CARTESIAN_POINT ( 'NONE',  ( -10.64923527428000050, -79.68499373684099396, 3.293689214829000012 ) ) ;
#34872=ADVANCED_FACE ( 'NONE', ( #47757 ), #38216, .F. ) ;
#34885=VERTEX_POINT ( 'NONE', #52458 ) ;
#34891=CARTESIAN_POINT ( 'NONE',  ( -0.2440801457610911052, -81.00000000000000000, -10.96803368417560876 ) ) ;
#34892=CARTESIAN_POINT ( 'NONE',  ( -10.30400671801000101, -77.54662084572800040, 3.605941145585999763 ) ) ;
#34894=CARTESIAN_POINT ( 'NONE',  ( -9.805641529082999241, -79.23866588669099542, -5.446788484474000214 ) ) ;
#34910=CARTESIAN_POINT ( 'NONE',  ( -5.582142573279000430, -79.09604631854099921, -10.84844757254999870 ) ) ;
#34912=CARTESIAN_POINT ( 'NONE',  ( -10.61596739836999959, -78.74002463773399541, -5.551333230057999835 ) ) ;
#34918=SURFACE_STYLE_USAGE ( .BOTH. , #57377 ) ;
#34920=CARTESIAN_POINT ( 'NONE',  ( -11.07095105964000048, -78.38183842717499772, 1.299477954992000139 ) ) ;
#34922=CARTESIAN_POINT ( 'NONE',  ( 11.08684999561000062, -80.58721576625140415, 1.943057827011999805 ) ) ;
#34924=CARTESIAN_POINT ( 'NONE',  ( 9.984017254981603529, -80.28079889738930319, 4.071156503779067570 ) ) ;
#34939=CARTESIAN_POINT ( 'NONE',  ( -3.573177736666999671, -77.04238470710198783, 10.43715168250999881 ) ) ;
#34945=CARTESIAN_POINT ( 'NONE',  ( -5.781545516559535081, -80.17986992905298393, -9.063146604324529676 ) ) ;
#34949=CARTESIAN_POINT ( 'NONE',  ( 7.652056849482000267, -79.38624118732400348, 9.281873293285000770 ) ) ;
#34951=EDGE_CURVE ( 'NONE', #35616, #9151, #29047, .T. ) ;
#34952=CARTESIAN_POINT ( 'NONE',  ( -0.4163023988263999664, -79.44546714899098561, -11.25436168207999899 ) ) ;
#34961=CYLINDRICAL_SURFACE ( 'NONE', #52730, 11.05000000000000071 ) ;
#34963=CARTESIAN_POINT ( 'NONE',  ( 5.472379214682000281, -79.74019400902800214, -9.446080217779000421 ) ) ;
#34966=CARTESIAN_POINT ( 'NONE',  ( 3.042547531669000271, -78.24783470746899638, -10.31045122763999977 ) ) ;
#34970=CARTESIAN_POINT ( 'NONE',  ( -2.807719666672398695, -79.80000000000001137, 11.69429938913882694 ) ) ;
#34972=CARTESIAN_POINT ( 'NONE',  ( -10.59627636761023339, -80.08682005774406321, 1.811415407155257729 ) ) ;
#34973=PLANE ( 'NONE',  #37155 ) ;
#34978=CARTESIAN_POINT ( 'NONE',  ( 10.91568895729999866, -76.21867431695000050, 1.352609846672000016 ) ) ;
#34990=ORIENTED_EDGE ( 'NONE', *, *, #35614, .F. ) ;
#34991=CARTESIAN_POINT ( 'NONE',  ( 8.596418555780417137, -80.19791666666667140, -6.606377239730353956 ) ) ;
#34992=CARTESIAN_POINT ( 'NONE',  ( -11.85739648576925909, -79.28587530551916984, 2.129864859879342820 ) ) ;
#35002=CARTESIAN_POINT ( 'NONE',  ( 10.99960575394902129, -80.99614106727162266, -0.5334183479100040870 ) ) ;
#35009=CARTESIAN_POINT ( 'NONE',  ( 4.239312547723716129, -79.94287370176201080, 9.878703068895035244 ) ) ;
#35018=CARTESIAN_POINT ( 'NONE',  ( -10.75000000000000000, -80.50000000000000000, -1.711887504597999906E-14 ) ) ;
#35026=ORIENTED_EDGE ( 'NONE', *, *, #27080, .T. ) ;
#35035=CARTESIAN_POINT ( 'NONE',  ( -8.255731568163469092, -80.90898308749885359, -7.584690471252304889 ) ) ;
#35054=CARTESIAN_POINT ( 'NONE',  ( -11.77559907170000031, -77.89629421814900923, -3.482965070681999897 ) ) ;
#35059=CARTESIAN_POINT ( 'NONE',  ( -5.099192467852374122, -79.51443440021429865, 9.463776008281715946 ) ) ;
#35061=CARTESIAN_POINT ( 'NONE',  ( -12.00000000000000355, -78.89293765275958492, 1.064976873965742366 ) ) ;
#35062=CARTESIAN_POINT ( 'NONE',  ( 8.263989999164000011, -79.07297727176099045, 8.606143803265000614 ) ) ;
#35068=CARTESIAN_POINT ( 'NONE',  ( -10.75000000000000000, -77.00000000000000000, 0.000000000000000000 ) ) ;
#35080=VERTEX_POINT ( 'NONE', #28777 ) ;
#35081=DIRECTION ( 'NONE',  ( -0.7071067811864976127, 0.7071067811865975328, 1.603636560452993712E-09 ) ) ;
#35093=CARTESIAN_POINT ( 'NONE',  ( 4.323029931973999318, -76.84458834893798951, -11.57148487019000171 ) ) ;
#35094=DIRECTION ( 'NONE',  ( -1.000000000000000000, 0.000000000000000000, 0.000000000000000000 ) ) ;
#35102=CARTESIAN_POINT ( 'NONE',  ( 2.976864594307000011, -77.39637571049389919, -10.81463766284999828 ) ) ;
#35104=CARTESIAN_POINT ( 'NONE',  ( 6.766402264611000028, -79.57821326152900099, -8.946167390840999545 ) ) ;
#35112=CARTESIAN_POINT ( 'NONE',  ( -10.31421052434999908, -76.82175206120300004, 3.823226550887000030 ) ) ;
#35122=CARTESIAN_POINT ( 'NONE',  ( -8.596418555780431348, -79.55208333333332860, -6.606377239730338857 ) ) ;
#35125=B_SPLINE_SURFACE_WITH_KNOTS ( 'NONE', 3, 3, ( 
 ( #51172, #20448, #15721, #20735, #11881, #29573, #47630, #7445, #7153, #55883, #28704, #39023, #34004, #3020, #25154, #21017, #43180, #24583, #47042, #6274, #2735, #19868, #51464, #38732, #56751, #16311, #11019, #34292, #29285, #52326, #15133, #42307, #2162, #37863, #29003 ),
 ( #20162, #33130, #6572, #10726, #42599, #38151, #56173, #35437, #7730, #58187, #49046, #44614, #44318, #48756, #39881, #53179, #53466, #12728, #3308, #44037, #4169, #8888, #26883, #53769, #30148, #39597, #21302, #22462, #39310, #34865, #34579, #31299, #13008, #35738, #44907 ),
 ( #4463, #30721, #8593, #26011, #40175, #57600, #52611, #57320, #16884, #12162, #57035, #17451, #8303, #31008, #48198, #26303, #17161, #22167, #13305, #26580, #17750, #49342, #16594, #52895, #25730, #43756, #3873, #12445, #57894, #30441, #21873, #8014, #48471, #3587, #21591 ),
 ( #35147, #1219, #9183, #49637, #54643, #40766, #41639, #36910, #55213, #36038, #31595, #32178, #40474, #5333, #27463, #36624, #27169, #19209, #18339, #5048, #5616, #18916, #45206, #37201, #32465, #28044, #27754, #50218, #23340, #14182, #54921, #9766, #4754, #45501, #46090 ) ),
 .UNSPECIFIED., .F., .F., .F.,
 ( 4, 4 ),
 ( 4, 1, 1, 1, 1, 1, 1, 1, 1, 1, 1, 1, 1, 1, 1, 1, 1, 1, 1, 1, 1, 1, 1, 1, 1, 1, 1, 1, 1, 1, 1, 1, 4 ),
 ( -0.1772706441294000235, 1.177270644128999955 ),
 ( -0.01390847417841000085, 0.008692796361505999644, 0.03129406690142000347, 0.05389533744134000076, 0.07649660798125000605, 0.09909787852116999640, 0.1216991490611000065, 0.1443004196010000129, 0.1669016901409000053, 0.1895029606807999978, 0.2121042312206999902, 0.2347055017607000138, 0.2573067723006000063, 0.2799080428405000265, 0.3025093133803999912, 0.3251105839203000114, 0.3477118544601999761, 0.3703131250002000274, 0.3929143955401000476, 0.4155156660800000124, 0.4381169366199000326, 0.4607182071597999973, 0.4833194776997000175, 0.5059207482395999822, 0.5285220187796000335, 0.5511232893194999427, 0.5737245598593999629, 0.5963258303992999831, 0.6189271009392000034, 0.6415283714791000236, 0.6641296420191000749, 0.6867309125589999841, 0.7093321830989000043 ),
 .UNSPECIFIED. ) ;
#35130=CARTESIAN_POINT ( 'NONE',  ( -8.885616033064000163, -78.00760259185899770, 8.035041515002001589 ) ) ;
#35134=CARTESIAN_POINT ( 'NONE',  ( -12.00019890019965096, -76.39977373798492977, -1.177339121803222359E-06 ) ) ;
#35137=CARTESIAN_POINT ( 'NONE',  ( 12.00000000000000888, -78.53958333333332575, -1.570796326794872577 ) ) ;
#35147=CARTESIAN_POINT ( 'NONE',  ( 8.159281975656000441, -77.05763688248899257, -8.859554478729998905 ) ) ;
#35151=CARTESIAN_POINT ( 'NONE',  ( -7.286644543156999276, -79.20872152740099637, -8.282906837769999697 ) ) ;
#35155=CARTESIAN_POINT ( 'NONE',  ( -10.57172952794455156, -76.48333333333334849, 2.251292830498277109 ) ) ;
#35159=CARTESIAN_POINT ( 'NONE',  ( 5.022587898441999599, -78.48512198850698951, -11.20577484976000093 ) ) ;
#35160=CARTESIAN_POINT ( 'NONE',  ( -1.407171709420465211, -79.38541666666665719, 10.74999999999999467 ) ) ;
#35162=AXIS2_PLACEMENT_3D ( 'NONE', #28452, #19609, #45911 ) ;
#35166=CARTESIAN_POINT ( 'NONE',  ( 10.40070879200345466, -78.82965153313729445, -2.740125206622860965 ) ) ;
#35171=CARTESIAN_POINT ( 'NONE',  ( -10.75986520424384274, -81.00000000000001421, -0.7996052922503522620 ) ) ;
#35178=CARTESIAN_POINT ( 'NONE',  ( -10.71602610194999805, -79.74223592799599203, 3.314346869870000489 ) ) ;
#35194=CARTESIAN_POINT ( 'NONE',  ( 2.784107197330000005, -79.65218441210198819, -11.87846276067000062 ) ) ;
#35196=CARTESIAN_POINT ( 'NONE',  ( 5.537129384246000541, -79.03844710739599577, 10.62336504503000079 ) ) ;
#35203=CARTESIAN_POINT ( 'NONE',  ( -0.9550654082404999023, -78.20516599075500608, 11.22148896650999816 ) ) ;
#35205=CARTESIAN_POINT ( 'NONE',  ( -10.85082013035999893, -80.80199725428047941, 2.992226394595999928 ) ) ;
#35220=CARTESIAN_POINT ( 'NONE',  ( 0.000000000000000000, -82.09999999999999432, 0.000000000000000000 ) ) ;
#35222=CARTESIAN_POINT ( 'NONE',  ( 4.029831046159999985, -78.43071061401199984, -10.51637221458999960 ) ) ;
#35227=LINE ( 'NONE', #53258, #42161 ) ;
#35228=CARTESIAN_POINT ( 'NONE',  ( -3.860146505116679005, -80.19620181100606260, -10.03328294032903578 ) ) ;
#35230=CARTESIAN_POINT ( 'NONE',  ( 6.606377239730347739, -77.17708333333330017, -8.596418555780422466 ) ) ;
#35235=CARTESIAN_POINT ( 'NONE',  ( -6.231249681807000229, -79.74506692201100577, 9.381124237602000093 ) ) ;
#35237=CARTESIAN_POINT ( 'NONE',  ( 2.813637286836895068, -77.45420692980438560, 10.46962234225027366 ) ) ;
#35247=CARTESIAN_POINT ( 'NONE',  ( 9.200987374210999548, -78.86863103297000066, 5.875133813785999415 ) ) ;
#35260=FACE_BOUND ( 'NONE', #49335, .T. ) ;
#35266=CARTESIAN_POINT ( 'NONE',  ( 9.958655842330001562, -76.24375625893898700, 4.669801055666999545 ) ) ;
#35273=CARTESIAN_POINT ( 'NONE',  ( 10.07210119001000059, -80.62085295350529179, 5.045985883512999592 ) ) ;
#35294=CARTESIAN_POINT ( 'NONE',  ( -3.135571036917709886, -79.99881628433968217, 10.28260097463162914 ) ) ;
#35297=ORIENTED_EDGE ( 'NONE', *, *, #42905, .F. ) ;
#35298=CARTESIAN_POINT ( 'NONE',  ( -2.904718832244216564, -77.20339151522927068, -10.35162020224675139 ) ) ;
#35307=CARTESIAN_POINT ( 'NONE',  ( 4.527593368978999777, -77.60351546138099366, 11.29085598690000047 ) ) ;
#35322=FACE_OUTER_BOUND ( 'NONE', #16176, .T. ) ;
#35324=ADVANCED_FACE ( 'NONE', ( #6055 ), #23480, .F. ) ;
#35327=CARTESIAN_POINT ( 'NONE',  ( 6.035966914210000311, -77.98297998349713112, 10.34809972146999968 ) ) ;
#35341=ADVANCED_FACE ( 'NONE', ( #19066 ), #37054, .F. ) ;
#35346=CARTESIAN_POINT ( 'NONE',  ( -9.904830252356999765, -76.99205734789899225, 4.590139709818999769 ) ) ;
#35347=CARTESIAN_POINT ( 'NONE',  ( -7.278283919121999901, -77.36717634323900938, 9.747261860606000639 ) ) ;
#35352=CARTESIAN_POINT ( 'NONE',  ( -9.358528765448124176, -79.55917755226546717, 5.292934104458898226 ) ) ;
#35355=CARTESIAN_POINT ( 'NONE',  ( 2.220113589157999723, -79.83089276362140652, -11.83482178057999867 ) ) ;
#35357=CARTESIAN_POINT ( 'NONE',  ( 1.822780608403999913, -80.50309514466069061, 11.02275947276000068 ) ) ;
#35374=CARTESIAN_POINT ( 'NONE',  ( 0.000000000000000000, -90.35000000009100063, 0.000000000000000000 ) ) ;
#35381=CARTESIAN_POINT ( 'NONE',  ( -6.658992300009000331, -76.27083001266900908, -10.40411675648000056 ) ) ;
#35391=CARTESIAN_POINT ( 'NONE',  ( -7.301194973305000779, -79.33308617451200462, 8.515319286630999684 ) ) ;
#35393=DIRECTION ( 'NONE',  ( 0.000000000000000000, -1.000000000000000000, 0.000000000000000000 ) ) ;
#35395=ORIENTED_EDGE ( 'NONE', *, *, #28233, .F. ) ;
#35410=CARTESIAN_POINT ( 'NONE',  ( 8.596418555780450887, -79.69791666666668561, -6.606377239730321982 ) ) ;
#35411=CARTESIAN_POINT ( 'NONE',  ( -8.982117338527000783, -79.69889424580067327, 6.718606902359000266 ) ) ;
#35412=CARTESIAN_POINT ( 'NONE',  ( -1.407171709420465211, -77.88541666666667140, 10.74999999999999467 ) ) ;
#35417=FACE_OUTER_BOUND ( 'NONE', #49785, .T. ) ;
#35418=CARTESIAN_POINT ( 'NONE',  ( -10.75000000000000000, -79.10000000000000853, 0.000000000000000000 ) ) ;
#35421=CARTESIAN_POINT ( 'NONE',  ( 11.32533557775999888, -77.80105294172599883, -3.764608412264000226 ) ) ;
#35434=CARTESIAN_POINT ( 'NONE',  ( 1.633411169670999863, -77.97052377699598935, -11.09730050697999992 ) ) ;
#35437=CARTESIAN_POINT ( 'NONE',  ( -10.58700924204000060, -76.96669458148599574, 6.201838006055000463 ) ) ;
#35441=CARTESIAN_POINT ( 'NONE',  ( 5.768362037549999322, -78.30992220834100692, -9.403610972502001175 ) ) ;
#35449=CARTESIAN_POINT ( 'NONE',  ( -0.08732773870155000062, -78.70215651189698747, 12.27958277169999945 ) ) ;
#35451=EDGE_CURVE ( 'NONE', #1173, #36999, #534, .T. ) ;
#35456=CARTESIAN_POINT ( 'NONE',  ( 2.813789756862229652, -78.35416666666665719, 10.47020627418440064 ) ) ;
#35461=CARTESIAN_POINT ( 'NONE',  ( -10.75000000000000000, -78.00000000000000000, 2.252154972635999871E-14 ) ) ;
#35469=CARTESIAN_POINT ( 'NONE',  ( 2.179295889402999897, -78.55775731164598596, 11.00312592022000047 ) ) ;
#35486=CARTESIAN_POINT ( 'NONE',  ( 12.19992621721999981, -79.20211240836600552, 1.693460693027999842 ) ) ;
#35488=CARTESIAN_POINT ( 'NONE',  ( -5.786162884931686179, -78.02038376788627261, 9.061535599160601251 ) ) ;
#35490=CARTESIAN_POINT ( 'NONE',  ( 9.789819849890999848, -78.83501197700098828, -6.904744247936999813 ) ) ;
#35492=CONICAL_SURFACE ( 'NONE', #10078, 13.94999999993999928, 0.7853981633972997312 ) ;
#35494=CARTESIAN_POINT ( 'NONE',  ( 0.000000000000000000, -90.29999999999999716, 0.000000000000000000 ) ) ;
#35498=CARTESIAN_POINT ( 'NONE',  ( -4.550163292746999488, -77.41531204370200214, -10.30194052436999996 ) ) ;
#35500=CARTESIAN_POINT ( 'NONE',  ( -1.822066877594999967, -80.21134816220060770, 11.10737283064000103 ) ) ;
#35506=AXIS2_PLACEMENT_3D ( 'NONE', #5107, #18104, #49101 ) ;
#35520=CARTESIAN_POINT ( 'NONE',  ( -8.684735281668000795, -77.83151106797200214, -7.170030519161000093 ) ) ;
#35526=CARTESIAN_POINT ( 'NONE',  ( 3.969016993814154848, -80.25512807981924368, -9.991659506732283091 ) ) ;
#35533=CARTESIAN_POINT ( 'NONE',  ( 10.58513040395000004, -78.60114051593500051, 3.845644306921999878 ) ) ;
#35545=CARTESIAN_POINT ( 'NONE',  ( -11.02198032011999906, -79.64450301542999000, -0.4665663988222000236 ) ) ;
#35564=CARTESIAN_POINT ( 'NONE',  ( -10.81829297021999992, -76.44441179485198745, 1.986553170785000155 ) ) ;
#35571=CARTESIAN_POINT ( 'NONE',  ( -0.8455117474470024153, -80.98139262285351947, 10.71661036402546330 ) ) ;
#35572=CARTESIAN_POINT ( 'NONE',  ( 11.22355342542000045, -80.59075526750170582, 0.9700744431168999427 ) ) ;
#35593=CARTESIAN_POINT ( 'NONE',  ( -5.052420809101000088E-14, -80.79999999999999716, -13.89999999999999858 ) ) ;
#35596=CARTESIAN_POINT ( 'NONE',  ( -4.008563851605106976, -77.19461823621462315, -9.976209684486235574 ) ) ;
#35604=CARTESIAN_POINT ( 'NONE',  ( -11.75651041636212746, -76.05651041660414080, -1.538071389465395677 ) ) ;
#35607=CARTESIAN_POINT ( 'NONE',  ( -8.937463246932001226, -78.13263333629100771, 8.081925660605000061 ) ) ;
#35614=EDGE_CURVE ( 'NONE', #20674, #26795, #19502, .T. ) ;
#35616=VERTEX_POINT ( 'NONE', #57247 ) ;
#35620=DIRECTION ( 'NONE',  ( -1.000000000000000000, 0.000000000000000000, 0.000000000000000000 ) ) ;
#35638=CARTESIAN_POINT ( 'NONE',  ( 2.244378098519284936, -78.24176656480896952, -10.54564492727542024 ) ) ;
#35643=CARTESIAN_POINT ( 'NONE',  ( -0.8033103333046999195, -77.64572957994299429, -10.88715107357000100 ) ) ;
#35645=CARTESIAN_POINT ( 'NONE',  ( -10.52667135666000142, -78.33036326492899093, 6.323366929881999887 ) ) ;
#35647=CARTESIAN_POINT ( 'NONE',  ( -10.75000000000000000, -79.01041666666667140, -1.407171709420429018 ) ) ;
#35651=ORIENTED_EDGE ( 'NONE', *, *, #56411, .T. ) ;
#35653=CARTESIAN_POINT ( 'NONE',  ( -9.403529956545000346, -79.07069129717299916, 7.335493971768999977 ) ) ;
#35654=CARTESIAN_POINT ( 'NONE',  ( 6.339406590914999917, -80.46812245865710622, 9.199765193516999062 ) ) ;
#35657=CARTESIAN_POINT ( 'NONE',  ( -11.16975252231999960, -76.82659737091999830, 1.027088271520000040 ) ) ;
#35672=CARTESIAN_POINT ( 'NONE',  ( 3.140974612311377090, -76.94583333333332575, -11.68767212001978528 ) ) ;
#35688=CARTESIAN_POINT ( 'NONE',  ( -1.918609024215000014, -76.73587854621999327, -12.08329390949000093 ) ) ;
#35689=CARTESIAN_POINT ( 'NONE',  ( -9.768056576080892839, -78.63443854277882394, -4.490846406839354543 ) ) ;
#35696=CARTESIAN_POINT ( 'NONE',  ( 10.79417609527999922, -77.47808473949946517, -3.050225076229999832 ) ) ;
#35698=CARTESIAN_POINT ( 'NONE',  ( -11.19989528650999944, -78.89730468648299677, 0.6168112860373000661 ) ) ;
#35710=CARTESIAN_POINT ( 'NONE',  ( 7.144724566336000393, -76.52727280461898829, 9.988770583665001368 ) ) ;
#35715=CARTESIAN_POINT ( 'NONE',  ( -10.75000000000000000, -79.50000000000000000, 0.000000000000000000 ) ) ;
#35716=CARTESIAN_POINT ( 'NONE',  ( 8.554126827399000987, -79.94402133281720069, -7.255689219360999864 ) ) ;
#35726=CARTESIAN_POINT ( 'NONE',  ( -11.69669687464000063, -78.56067377359198645, 2.371241166392999755 ) ) ;
#35730=CARTESIAN_POINT ( 'NONE',  ( -5.250095168255000111, -80.11166617326099981, -9.571408815458999797 ) ) ;
#35738=CARTESIAN_POINT ( 'NONE',  ( -11.85634656288999977, -75.99822096499200086, 1.610826861118999975 ) ) ;
#35740=CARTESIAN_POINT ( 'NONE',  ( -10.75000000000000000, -77.60000000000000853, 2.252154972635999871E-14 ) ) ;
#35742=CARTESIAN_POINT ( 'NONE',  ( 11.26004178396000199, -80.02508423127190440, -0.2131731071575000136 ) ) ;
#35751=CARTESIAN_POINT ( 'NONE',  ( -12.22643784615999962, -77.83401841833600088, -1.144550905343000080 ) ) ;
#35754=CARTESIAN_POINT ( 'NONE',  ( -8.596418555780466875, -79.44791666666665719, 6.606377239730298001 ) ) ;
#35755=CARTESIAN_POINT ( 'NONE',  ( -10.75000000000000000, -78.50000000000000000, 0.000000000000000000 ) ) ;
#35760=CARTESIAN_POINT ( 'NONE',  ( 10.48060664564022737, -78.83212343620286333, -2.412640484422836185 ) ) ;
#35762=AXIS2_PLACEMENT_3D ( 'NONE', #42960, #56531, #16090 ) ;
#35767=CARTESIAN_POINT ( 'NONE',  ( -9.301504212792000459, -78.18631111317900206, -5.931589059777999218 ) ) ;
#35772=CARTESIAN_POINT ( 'NONE',  ( 9.376438147752001129, -79.40208394470199949, -6.156339679782000474 ) ) ;
#35787=CARTESIAN_POINT ( 'NONE',  ( 11.31276370261999986, -79.72349187107899127, 4.871084483227000383 ) ) ;
#35788=CARTESIAN_POINT ( 'NONE',  ( -11.35374465838000013, -76.14602084646099911, -0.6977592397238999711 ) ) ;
#35789=CARTESIAN_POINT ( 'NONE',  ( -5.897312117113708396, -78.02137868188400205, 8.988332804861963510 ) ) ;
#35790=CARTESIAN_POINT ( 'NONE',  ( -11.92766985523999956, -77.70911065163099352, -1.116582401450000095 ) ) ;
#35798=CARTESIAN_POINT ( 'NONE',  ( 2.837175473061999575, -78.24565671216601004, 10.77984396480000129 ) ) ;
#35814=B_SPLINE_SURFACE_WITH_KNOTS ( 'NONE', 3, 3, ( 
 ( #7240, #16969, #48563, #26103, #11968, #56547, #57692, #47710, #17248, #8390, #44127, #57118, #34088, #7532, #11683, #26386, #20534, #35235, #43848, #3676, #57412, #53268, #16108, #29944, #16684, #38532, #25245, #52125, #34952, #48282, #25820, #21390, #52983, #30239, #7821, #29660, #21678, #12533, #39683, #20814, #43264, #2819, #38821, #47998, #25531, #43549, #3114, #21105, #34666, #52695, #12249, #23141, #27266, #9571, #35832, #26676, #22257, #21962, #18721, #35533, #40571, #5142, #8987, #41148, #44707, #740, #4261 ),
 ( #58283, #49734, #39972, #26970, #36715, #54728, #44407, #22850, #40272, #53561, #53862, #32270, #45002, #17846, #4559, #14273, #50315, #27555, #9862, #36423, #3959, #49436, #13395, #13986, #50025, #31396, #22560, #57986, #164, #45599, #18139, #17543, #13100, #31983, #31096, #36135, #18433, #49133, #8685, #9277, #54151, #13693, #31688, #45303, #4854, #40862, #452, #54450, #24312, #32850, #41444, #19304, #1028, #11041, #45890, #55902, #19587, #42326, #15152, #15456, #5422, #46187, #10443, #51483, #14565, #33445, #33147 ),
 ( #51192, #24011, #42028, #19010, #1894, #10747, #6299, #50608, #46775, #37003, #1596, #1311, #28723, #55020, #32558, #19886, #29023, #47062, #37880, #27845, #23432, #10157, #37587, #50897, #28430, #5712, #28134, #55309, #23720, #41732, #37294, #14855, #46478, #6004, #55605, #31881, #31288, #17742, #10055, #18034, #18907, #36614, #40757, #9758, #50208, #23333, #36027, #31583, #27160, #14465, #640, #9469, #40163, #41343, #27743, #351, #27454, #28037, #45790, #26872, #5326, #927, #5035, #50501, #18330, #36900, #44899 ),
 ( #54913, #32456, #46082, #13588, #54636, #4452, #22453, #45492, #22156, #40467, #58177, #35730, #45199, #23037, #53758, #49924, #9176, #13295, #41053, #49333, #8878, #59, #18623, #14172, #54053, #32169, #49628, #4746, #22747, #36323, #54347, #13886, #1497, #38071, #33344, #51377, #28321, #32749, #56091, #15051, #46373, #15637, #10342, #56378, #55503, #11511, #28915, #37192, #6486, #33916, #24497, #51955, #33043, #50797, #42511, #2081, #38356, #33633, #19487, #5897, #20361, #15929, #23907, #42802, #5607, #2364, #51675 ) ),
 .UNSPECIFIED., .F., .F., .F.,
 ( 4, 4 ),
 ( 4, 1, 1, 1, 1, 1, 1, 1, 1, 1, 1, 1, 1, 1, 1, 1, 1, 1, 1, 1, 1, 1, 1, 1, 1, 1, 1, 1, 1, 1, 1, 1, 1, 1, 1, 1, 1, 1, 1, 1, 1, 1, 1, 1, 1, 1, 1, 1, 1, 1, 1, 1, 1, 1, 1, 1, 1, 1, 1, 1, 1, 1, 1, 1, 4 ),
 ( -0.1772706441294000235, 1.177270644128999955 ),
 ( -0.02000000000000000042, -0.003749999999999999861, 0.01250000000000000069, 0.02875000000000000125, 0.04499999999999999833, 0.06124999999999999889, 0.07749999999999999944, 0.09375000000000000000, 0.1100000000000000006, 0.1262500000000000011, 0.1424999999999999878, 0.1587500000000000022, 0.1749999999999999889, 0.1912500000000000033, 0.2074999999999999900, 0.2237500000000000044, 0.2399999999999999911, 0.2562499999999999778, 0.2725000000000000200, 0.2887500000000000067, 0.3049999999999999933, 0.3212499999999999800, 0.3375000000000000222, 0.3537500000000000089, 0.3699999999999999956, 0.3862499999999999822, 0.4025000000000000244, 0.4187500000000000111, 0.4349999999999999978, 0.4512499999999999845, 0.4675000000000000266, 0.4837500000000000133, 0.5000000000000000000, 0.5162499999999999867, 0.5324999999999999734, 0.5487499999999999600, 0.5649999999999999467, 0.5812500000000000444, 0.5975000000000000311, 0.6137500000000000178, 0.6300000000000000044, 0.6462499999999999911, 0.6624999999999999778, 0.6787499999999999645, 0.6949999999999999512, 0.7112500000000000488, 0.7275000000000000355, 0.7437500000000000222, 0.7600000000000000089, 0.7762499999999999956, 0.7924999999999999822, 0.8087499999999999689, 0.8249999999999999556, 0.8412500000000000533, 0.8575000000000000400, 0.8737500000000000266, 0.8900000000000000133, 0.9062500000000000000, 0.9224999999999999867, 0.9387499999999999734, 0.9549999999999999600, 0.9712499999999999467, 0.9875000000000000444, 1.003749999999999920, 1.020000000000000018 ),
 .UNSPECIFIED. ) ;
#35820=CARTESIAN_POINT ( 'NONE',  ( -7.664623337597000763, -77.27352982952599803, -8.093710500358000104 ) ) ;
#35821=EDGE_CURVE ( 'NONE', #51047, #5424, #22693, .T. ) ;
#35827=CARTESIAN_POINT ( 'NONE',  ( 2.113904672446926813, -80.24111766284364933, -10.53987543967868312 ) ) ;
#35828=CARTESIAN_POINT ( 'NONE',  ( 10.75000000000000355, -77.23958333333331439, -1.407171709420407035 ) ) ;
#35829=CARTESIAN_POINT ( 'NONE',  ( 10.54280189716214267, -78.62763935669978821, 3.830266094756761941 ) ) ;
#35832=CARTESIAN_POINT ( 'NONE',  ( -5.290207344092000774, -78.73732223094400240, 9.942216594703999988 ) ) ;
#35839=ADVANCED_FACE ( 'NONE', ( #24149 ), #33566, .F. ) ;
#35846=CARTESIAN_POINT ( 'NONE',  ( 7.779872909029999839, -79.45384861441699798, 7.821464818102998429 ) ) ;
#35854=VERTEX_POINT ( 'NONE', #9026 ) ;
#35865=CARTESIAN_POINT ( 'NONE',  ( 9.621556021936999770, -76.73787633716699474, -5.088820230768000386 ) ) ;
#35874=CARTESIAN_POINT ( 'NONE',  ( -6.474781754604000739, -80.41016915147990574, -9.218806710208998112 ) ) ;
#35898=CARTESIAN_POINT ( 'NONE',  ( -5.075520895105466224, -77.18593687418551497, -9.477339433974600880 ) ) ;
#35905=CARTESIAN_POINT ( 'NONE',  ( 11.70000000000000107, -80.79999999999999716, 0.000000000000000000 ) ) ;
#35907=CARTESIAN_POINT ( 'NONE',  ( 10.95272639356999989, -78.90591505001499684, 4.740592608656999829 ) ) ;
#35926=CARTESIAN_POINT ( 'NONE',  ( -11.96278216175999987, -78.14575587604012696, 0.6386762756999999624 ) ) ;
#35937=FACE_OUTER_BOUND ( 'NONE', #33104, .T. ) ;
#35946=CARTESIAN_POINT ( 'NONE',  ( 7.007185918478000097, -77.34612980692300255, 8.371063940391000102 ) ) ;
#35947=CARTESIAN_POINT ( 'NONE',  ( 11.82394432951000063, -78.60165641916699997, -3.315134025842000121 ) ) ;
#35957=CARTESIAN_POINT ( 'NONE',  ( -9.263776019951999174, -80.18834097062810429, -6.245495121194999832 ) ) ;
#35961=CARTESIAN_POINT ( 'NONE',  ( -6.984027423104000043, -77.26237885894900614, 8.777327129872999123 ) ) ;
#35977=CARTESIAN_POINT ( 'NONE',  ( 10.75000000000000000, -78.85000000000000853, 0.000000000000000000 ) ) ;
#35986=CARTESIAN_POINT ( 'NONE',  ( 12.19542156202999905, -76.36703390147599180, -0.9791554825414000574 ) ) ;
#35993=CARTESIAN_POINT ( 'NONE',  ( -8.649885944100999424, -77.80492085552104697, -7.141259254888000285 ) ) ;
#36007=CARTESIAN_POINT ( 'NONE',  ( -10.51110168222999874, -76.15842815987500103, 6.351495789100000344 ) ) ;
#36013=CARTESIAN_POINT ( 'NONE',  ( 10.12058791103999944, -79.53547618779010975, 4.836508133599999759 ) ) ;
#36014=CARTESIAN_POINT ( 'NONE',  ( 6.606377239730313988, -77.82291666666665719, 8.596418555780454440 ) ) ;
#36018=CARTESIAN_POINT ( 'NONE',  ( 0.000000000000000000, -90.39999999999999147, -9.599999999999999645 ) ) ;
#36019=CARTESIAN_POINT ( 'NONE',  ( 9.450487096927000508, -77.69565019976899123, -7.362360902974999455 ) ) ;
#36022=CARTESIAN_POINT ( 'NONE',  ( 9.414842545117998895, -77.77392362630298805, -7.334592169791999794 ) ) ;
#36027=CARTESIAN_POINT ( 'NONE',  ( 0.9420327262254000189, -79.09066710378499465, -10.99155624668999920 ) ) ;
#36038=CARTESIAN_POINT ( 'NONE',  ( -1.155714523305999997, -76.75577497604999166, 12.45063448816000040 ) ) ;
#36042=CARTESIAN_POINT ( 'NONE',  ( 8.679422240859999249, -78.40488561575499205, -6.994438423095999724 ) ) ;
#36050=CARTESIAN_POINT ( 'NONE',  ( -10.75000000000000000, -76.50000000000000000, 0.000000000000000000 ) ) ;
#36056=( NAMED_UNIT ( * ) SI_UNIT ( $, .STERADIAN. ) SOLID_ANGLE_UNIT ( ) );
#36057=CARTESIAN_POINT ( 'NONE',  ( 10.48543666025108401, -77.09166666666666856, 6.043427764450814976 ) ) ;
#36067=CARTESIAN_POINT ( 'NONE',  ( -5.656567264032000608, -77.72329328214799204, -9.471271359694998893 ) ) ;
#36072=CARTESIAN_POINT ( 'NONE',  ( 10.49311453041000064, -79.98736301501259049, -3.963918880051000126 ) ) ;
#36075=ORIENTED_EDGE ( 'NONE', *, *, #25630, .T. ) ;
#36093=CARTESIAN_POINT ( 'NONE',  ( -6.568157394400000015, -79.86252639446888679, 9.960850882888999891 ) ) ;
#36094=CARTESIAN_POINT ( 'NONE',  ( 0.1565658240112999811, -75.94730213011300179, 11.25550456148000045 ) ) ;
#36095=CARTESIAN_POINT ( 'NONE',  ( -5.081867896333786661, -78.01424454617936988, 9.472916454327915403 ) ) ;
#36096=CARTESIAN_POINT ( 'NONE',  ( 11.88382656225999945, -78.37381361479698683, -1.513515996960000054 ) ) ;
#36098=CARTESIAN_POINT ( 'NONE',  ( -10.68107435978283526, -79.08975591983691800, 1.407249667601314203 ) ) ;
#36100=CARTESIAN_POINT ( 'NONE',  ( 1.676866965995471581, -80.96289916692815325, 10.61818188551169762 ) ) ;
#36103=CARTESIAN_POINT ( 'NONE',  ( 10.27624888046999985, -78.10947499715699394, -4.318947732659999872 ) ) ;
#36105=CARTESIAN_POINT ( 'NONE',  ( -11.11481121949999995, -80.89657200469704890, -0.7603797884353999947 ) ) ;
#36111=CARTESIAN_POINT ( 'NONE',  ( -11.16975252231999960, -76.69102026436699759, 1.027088271520000040 ) ) ;
#36114=CARTESIAN_POINT ( 'NONE',  ( 10.40641373605281572, -76.87100247242075568, 2.787300749583467852 ) ) ;
#36122=CARTESIAN_POINT ( 'NONE',  ( -0.9550654082404999023, -78.15834718399401027, 11.22148896650999816 ) ) ;
#36135=CARTESIAN_POINT ( 'NONE',  ( -7.255688098778000139, -79.32253981239199447, 8.462245020330000145 ) ) ;
#36141=MANIFOLD_SOLID_BREP ( 'Stock-MAS-694-1', #27688 ) ;
#36154=VERTEX_POINT ( 'NONE', #44093 ) ;
#36156=CARTESIAN_POINT ( 'NONE',  ( -5.508096857961803927, -76.98721230508247970, -10.70907476296403971 ) ) ;
#36163=CIRCLE ( 'NONE', #35162, 13.89999999999999858 ) ;
#36164=CARTESIAN_POINT ( 'NONE',  ( -7.568094764011999764, -76.39424791087300548, 7.981591190547998593 ) ) ;
#36165=DIRECTION ( 'NONE',  ( 0.000000000000000000, 1.000000000000000000, 0.000000000000000000 ) ) ;
#36168=CARTESIAN_POINT ( 'NONE',  ( 10.70339364929999881, -81.10241592956339218, 2.537196166659999808 ) ) ;
#36173=CARTESIAN_POINT ( 'NONE',  ( 5.136988255280226845, -77.24434066579330249, -10.56734161811198369 ) ) ;
#36176=CARTESIAN_POINT ( 'NONE',  ( -10.58783149161999937, -80.92942299481059365, -3.847989116766000084 ) ) ;
#36185=ADVANCED_FACE ( 'NONE', ( #41411 ), #20348, .T. ) ;
#36199=ORIENTED_EDGE ( 'NONE', *, *, #25141, .F. ) ;
#36200=CARTESIAN_POINT ( 'NONE',  ( 0.6835541566232417043, -77.23019398958709303, -10.73029167179032228 ) ) ;
#36206=DIRECTION ( 'NONE',  ( -0.9999896828222031298, 0.000000000000000000, -0.004542493714850020202 ) ) ;
#36207=CARTESIAN_POINT ( 'NONE',  ( 0.000000000000000000, -75.15999999999999659, 0.000000000000000000 ) ) ;
#36208=ORIENTED_EDGE ( 'NONE', *, *, #4331, .T. ) ;
#36209=CARTESIAN_POINT ( 'NONE',  ( -4.725986768004000638, -78.71600984204799545, -10.95903971673999955 ) ) ;
#36214=EDGE_CURVE ( 'NONE', #31986, #20195, #9015, .T. ) ;
#36215=CARTESIAN_POINT ( 'NONE',  ( 9.596002108778145967, -78.60208333333332575, 7.374560639699001996 ) ) ;
#36223=DIRECTION ( 'NONE',  ( 0.000000000000000000, -1.000000000000000000, 0.000000000000000000 ) ) ;
#36226=CARTESIAN_POINT ( 'NONE',  ( 11.97742283006000363, -77.90159203722610926, 0.2395971301470839476 ) ) ;
#36231=B_SPLINE_CURVE_WITH_KNOTS ( 'NONE', 3,
 ( #13632, #54672, #14213, #13335, #27202, #40798, #26912, #9802, #18369, #27785, #49671, #40508, #967, #32497, #9216, #45830, #49966, #27494, #36943, #8922, #23373, #5081, #31629, #23076, #41091, #682, #5366, #103, #18665, #18078 ),
 .UNSPECIFIED., .F., .F.,
 ( 4, 2, 1, 2, 2, 2, 2, 2, 2, 1, 2, 2, 2, 2, 2, 4 ),
 ( 0.000000000000000000, 0.1250000000000001665, 0.1875000000000002498, 0.2187500000000002776, 0.2500000000000003331, 0.3125000000000004996, 0.3750000000000006106, 0.4375000000000007772, 0.5000000000000008882, 0.5625000000000009992, 0.5937500000000008882, 0.6250000000000008882, 0.6875000000000006661, 0.7500000000000005551, 0.8750000000000002220, 1.000000000000000000 ),
 .UNSPECIFIED. ) ;
#36234=CARTESIAN_POINT ( 'NONE',  ( 0.9451020025315389761, -76.28046875000043769, 11.98011734817885987 ) ) ;
#36246=LINE ( 'NONE', #275, #3335 ) ;
#36249=CARTESIAN_POINT ( 'NONE',  ( -10.82730428396000022, -77.53678420793599457, -1.394578048285000094 ) ) ;
#36251=LINE ( 'NONE', #54271, #31661 ) ;
#36257=CARTESIAN_POINT ( 'NONE',  ( -10.90197693778999977, -79.65663117581799213, -4.835570938503999550 ) ) ;
#36258=CARTESIAN_POINT ( 'NONE',  ( -1.599027143172000009, -80.95995837030230291, 10.93957212085000030 ) ) ;
#36259=DIRECTION ( 'NONE',  ( 0.000000000000000000, -1.000000000000000000, 0.000000000000000000 ) ) ;
#36263=DIRECTION ( 'NONE',  ( 3.552713678800000476E-14, -1.000000000000000000, 2.634929311776999987E-13 ) ) ;
#36275=EDGE_LOOP ( 'NONE', ( #2038, #29881, #28336, #45734 ) ) ;
#36286=CARTESIAN_POINT ( 'NONE',  ( -2.015231956295000071, -76.14730429832600578, 11.93705991877000017 ) ) ;
#36293=CARTESIAN_POINT ( 'NONE',  ( 6.043427764450807871, -78.96666666666664014, -10.48543666025108934 ) ) ;
#36305=CARTESIAN_POINT ( 'NONE',  ( 6.725657209017000149, -77.37424939625499576, -9.843613558058999402 ) ) ;
#36319=CARTESIAN_POINT ( 'NONE',  ( -4.070249838183999991, -78.47928582732099301, 11.21911621747999810 ) ) ;
#36323=CARTESIAN_POINT ( 'NONE',  ( -4.041492642110999789, -79.62141199922800183, -10.14108984350000142 ) ) ;
#36330=CARTESIAN_POINT ( 'NONE',  ( -1.570796326794937636, -77.78541666666664867, 11.99999999999999467 ) ) ;
#36334=CARTESIAN_POINT ( 'NONE',  ( -0.2277317800897999955, -78.33225536775100295, -10.99999347944999961 ) ) ;
#36336=CARTESIAN_POINT ( 'NONE',  ( -9.393203674808288994, -79.95833333333331439, 5.413904038987134015 ) ) ;
#36352=CARTESIAN_POINT ( 'NONE',  ( -1.407199056997702646, -77.71460739497811687, -10.68073707906693848 ) ) ;
#36356=CARTESIAN_POINT ( 'NONE',  ( 0.5327216036087999429, -76.70229421267099212, -10.90374125898999935 ) ) ;
#36361=CARTESIAN_POINT ( 'NONE',  ( 10.54265532893000135, -78.54383683591599663, 3.830212845596999927 ) ) ;
#36372=CARTESIAN_POINT ( 'NONE',  ( -11.68767212001978706, -78.42083333333333428, -3.140974612311364655 ) ) ;
#36380=CARTESIAN_POINT ( 'NONE',  ( 7.541040361361999622, -78.82956348204299957, 9.261319756036000328 ) ) ;
#36381=CARTESIAN_POINT ( 'NONE',  ( 1.566004458289000034, -76.34473956280800166, -11.38667055607000123 ) ) ;
#36382=CARTESIAN_POINT ( 'NONE',  ( -5.117374279120588731, -78.01454871243346645, 9.453798672375675949 ) ) ;
#36383=CARTESIAN_POINT ( 'NONE',  ( -8.148905501844000199, -78.69936539988199797, -8.781309899900000104 ) ) ;
#36388=CARTESIAN_POINT ( 'NONE',  ( 6.897442179429761566, -80.91971616786906907, 8.256491842899244205 ) ) ;
#36392=CARTESIAN_POINT ( 'NONE',  ( 8.230685248253001518, -78.08223865415499176, -7.517341346183999740 ) ) ;
#36399=CARTESIAN_POINT ( 'NONE',  ( 10.29113596735999892, -77.48087421142000153, 4.462133020506000136 ) ) ;
#36403=CARTESIAN_POINT ( 'NONE',  ( -7.102903299382814062, -78.56775757425661766, -8.111946779019795883 ) ) ;
#36407=CARTESIAN_POINT ( 'NONE',  ( -11.75000000038751580, -76.05000000000001137, 1.230457119308518754 ) ) ;
#36410=CARTESIAN_POINT ( 'NONE',  ( -8.764875654205999567, -77.72256569596500242, 7.071839882566000490 ) ) ;
#36422=FACE_OUTER_BOUND ( 'NONE', #25402, .T. ) ;
#36423=CARTESIAN_POINT ( 'NONE',  ( 1.092964466808999946, -79.75832130042100232, 11.09324250366999998 ) ) ;
#36429=VERTEX_POINT ( 'NONE', #58394 ) ;
#36454=CARTESIAN_POINT ( 'NONE',  ( -9.421357847594000745, -80.24449435892378801, -6.176342950743000770 ) ) ;
#36460=CARTESIAN_POINT ( 'NONE',  ( 5.620590082324000036, -80.50046220949079157, -9.763102121971000358 ) ) ;
#36470=CARTESIAN_POINT ( 'NONE',  ( -4.687291826975000575, -79.51105952742696559, 9.674546195918276581 ) ) ;
#36471=EDGE_CURVE ( 'NONE', #24242, #21820, #26898, .T. ) ;
#36485=CARTESIAN_POINT ( 'NONE',  ( -4.332804415639630591, -77.19199523647633043, -9.839746177953021089 ) ) ;
#36497=CARTESIAN_POINT ( 'NONE',  ( 11.88272347344000046, -77.45440045069699408, 1.999161996513999950 ) ) ;
#36503=CARTESIAN_POINT ( 'NONE',  ( 6.043427764450761686, -78.63333333333329733, 10.48543666025110888 ) ) ;
#36504=CARTESIAN_POINT ( 'NONE',  ( -10.75000000000000000, -80.09999999999999432, -1.711887504597999906E-14 ) ) ;
#36512=CARTESIAN_POINT ( 'NONE',  ( 11.09875712452000052, -75.95812795482899560, 1.375294608629999971 ) ) ;
#36515=CARTESIAN_POINT ( 'NONE',  ( 0.4844284812283000119, -77.52178162129314387, 11.97002061315000176 ) ) ;
#36517=CARTESIAN_POINT ( 'NONE',  ( 7.508184180775703709, -77.03326573943833466, -8.333593418791714669 ) ) ;
#36531=CARTESIAN_POINT ( 'NONE',  ( -10.65320897811829859, -78.11245643503170299, -1.664319544042534904 ) ) ;
#36537=VECTOR ( 'NONE', #44586, 1000.000000000000114 ) ;
#36541=CARTESIAN_POINT ( 'NONE',  ( 12.10970598371999962, -77.13667338628398795, 2.037349774713999917 ) ) ;
#36548=EDGE_CURVE ( 'NONE', #12329, #52300, #36251, .T. ) ;
#36550=CARTESIAN_POINT ( 'NONE',  ( -9.893264523052000214, -80.61023151026600431, -4.935169213743999528 ) ) ;
#36553=CARTESIAN_POINT ( 'NONE',  ( 3.895497176768000003, -77.18066982994299963, 10.51870773133999926 ) ) ;
#36558=CARTESIAN_POINT ( 'NONE',  ( 10.29636973964252356, -81.00000000000000000, -3.915276559953854818 ) ) ;
#36573=ORIENTED_EDGE ( 'NONE', *, *, #37483, .T. ) ;
#36574=CARTESIAN_POINT ( 'NONE',  ( 0.03238307785349000406, -75.99818925673099557, 11.70563754594999750 ) ) ;
#36596=DIRECTION ( 'NONE',  ( 0.000000000000000000, 1.000000000000000000, 0.000000000000000000 ) ) ;
#36605=CARTESIAN_POINT ( 'NONE',  ( 0.000000000000000000, -75.15999999999999659, 0.000000000000000000 ) ) ;
#36606=CARTESIAN_POINT ( 'NONE',  ( -11.92766985523999956, -77.50574499180299881, -1.116582401450000095 ) ) ;
#36610=CARTESIAN_POINT ( 'NONE',  ( -11.88268207399999987, -77.58401841833600088, -1.112370969927999997 ) ) ;
#36614=CARTESIAN_POINT ( 'NONE',  ( 10.75129243007999946, -79.22684881879399654, 2.472133787718999720 ) ) ;
#36620=CARTESIAN_POINT ( 'NONE',  ( 2.813789756862229652, -77.35416666666665719, 10.47020627418440064 ) ) ;
#36624=CARTESIAN_POINT ( 'NONE',  ( 4.744332214898999034, -76.52937854621998781, -11.56915240781999898 ) ) ;
#36629=CARTESIAN_POINT ( 'NONE',  ( 10.47694508628999976, -78.48659464476099856, 3.806339902057000124 ) ) ;
#36631=CARTESIAN_POINT ( 'NONE',  ( -10.47020627418440242, -79.97916666666665719, 2.813789756862221214 ) ) ;
#36643=CARTESIAN_POINT ( 'NONE',  ( 10.10224734436263638, -78.82234514084187538, -3.676033498293930002 ) ) ;
#36644=CARTESIAN_POINT ( 'NONE',  ( 9.596002108778145967, -79.60208333333332575, 7.374560639699001996 ) ) ;
#36651=CARTESIAN_POINT ( 'NONE',  ( 9.148615368834404293, -77.85575384033435853, 7.734521845670259133 ) ) ;
#36652=CARTESIAN_POINT ( 'NONE',  ( 8.554126827399000987, -80.02791522528700341, -7.255689219360999864 ) ) ;
#36674=CARTESIAN_POINT ( 'NONE',  ( 10.33813847379999906, -79.23687103921299979, 6.695438874393000006 ) ) ;
#36675=CARTESIAN_POINT ( 'NONE',  ( -8.527808771699001866, -76.65038675065599705, 7.705797137820999509 ) ) ;
#36676=CARTESIAN_POINT ( 'NONE',  ( -2.100575672690006446, -77.99078096341597188, 10.54268409913574445 ) ) ;
#36680=CARTESIAN_POINT ( 'NONE',  ( 8.103107792609110405, -80.90736235359815964, 7.063989823860713280 ) ) ;
#36683=CARTESIAN_POINT ( 'NONE',  ( -9.465408641230000697, -77.34685739310599217, 5.887328751257999926 ) ) ;
#36685=CARTESIAN_POINT ( 'NONE',  ( -11.00003927284999961, -80.96429906910999819, -0.7525280789652001312 ) ) ;
#36690=CARTESIAN_POINT ( 'NONE',  ( -6.659967121051000305, -76.77272929337298990, -9.025682433062998555 ) ) ;
#36702=CARTESIAN_POINT ( 'NONE',  ( -3.647741209468000179, -77.17783883592798588, 10.65494948965999988 ) ) ;
#36709=CARTESIAN_POINT ( 'NONE',  ( -7.532536244959458394, -80.16368247948770431, -7.669252981571465178 ) ) ;
#36714=CARTESIAN_POINT ( 'NONE',  ( 6.321411194148057078, -79.08065831076486063, 10.10170745394536596 ) ) ;
#36715=CARTESIAN_POINT ( 'NONE',  ( 10.56933735542999919, -80.16686644544779483, 3.541701167072000445 ) ) ;
#36743=CARTESIAN_POINT ( 'NONE',  ( 3.862060628231000159, -80.68104832551259165, 10.58270681924999934 ) ) ;
#36749=CARTESIAN_POINT ( 'NONE',  ( 8.852642474645787019, -77.49067155497328940, -8.178101815369194227 ) ) ;
#36759=CARTESIAN_POINT ( 'NONE',  ( -7.614443659027361200, -79.53779634012535382, 7.588181420400903932 ) ) ;
#36762=EDGE_LOOP ( 'NONE', ( #3185, #46561, #21175, #38932, #33635 ) ) ;
#36779=ORIENTED_EDGE ( 'NONE', *, *, #24433, .F. ) ;
#36781=FACE_OUTER_BOUND ( 'NONE', #25314, .T. ) ;
#36783=CARTESIAN_POINT ( 'NONE',  ( 10.75624577990000041, -78.40392649052799356, -5.431293436759999871 ) ) ;
#36792=CARTESIAN_POINT ( 'NONE',  ( 7.374560639698954034, -78.62291666666662593, 9.596002108778181494 ) ) ;
#36801=CARTESIAN_POINT ( 'NONE',  ( -5.279550234765999939, -76.28419320068699960, -9.859017853534000508 ) ) ;
#36804=CARTESIAN_POINT ( 'NONE',  ( -1.667212297213999994, -76.71026873785200451, 11.10423992239999968 ) ) ;
#36816=CARTESIAN_POINT ( 'NONE',  ( 5.413904038987179312, -79.66666666666662877, -9.393203674808262349 ) ) ;
#36817=DIRECTION ( 'NONE',  ( 0.000000000000000000, 0.7071067811866525998, -0.7071067811864425456 ) ) ;
#36819=CARTESIAN_POINT ( 'NONE',  ( -10.48543666025111776, -79.35833333333330586, 6.043427764450754580 ) ) ;
#36829=CARTESIAN_POINT ( 'NONE',  ( -7.347140770713999736, -77.29944927882600325, 9.839476697348001011 ) ) ;
#36836=CARTESIAN_POINT ( 'NONE',  ( -2.662490087786000270, -79.23049308225799336, -11.62527415693000066 ) ) ;
#36837=CARTESIAN_POINT ( 'NONE',  ( -1.649606550861999921, -81.16313956354109393, 11.28560569546000103 ) ) ;
#36845=CARTESIAN_POINT ( 'NONE',  ( 3.399186938124000079, -81.00000000000000000, -10.46162167925000119 ) ) ;
#36846=ORIENTED_EDGE ( 'NONE', *, *, #23496, .F. ) ;
#36855=CARTESIAN_POINT ( 'NONE',  ( -0.8126767071385999630, -78.94632035071100518, -12.25297252704000073 ) ) ;
#36865=AXIS2_PLACEMENT_3D ( 'NONE', #11701, #56855, #23949 ) ;
#36877=ORIENTED_EDGE ( 'NONE', *, *, #43832, .F. ) ;
#36897=CARTESIAN_POINT ( 'NONE',  ( -7.140570215937000143, -77.50263047206500744, 9.562832187120999805 ) ) ;
#36900=CARTESIAN_POINT ( 'NONE',  ( -0.2253802134100999777, -78.58225536775100295, -10.88640714497000062 ) ) ;
#36908=EDGE_CURVE ( 'NONE', #47018, #35080, #33259, .T. ) ;
#36910=CARTESIAN_POINT ( 'NONE',  ( -10.78924115793999938, -76.83124045265999769, 6.320304850973999855 ) ) ;
#36916=CARTESIAN_POINT ( 'NONE',  ( 0.9518616847512999524, -78.84066710378499465, -11.10623968335000100 ) ) ;
#36918=CARTESIAN_POINT ( 'NONE',  ( 6.606377239730313988, -79.82291666666665719, 8.596418555780454440 ) ) ;
#36925=CARTESIAN_POINT ( 'NONE',  ( -9.760776772971999193, -92.33215535459000023, -3.252729338753999803E-10 ) ) ;
#36930=B_SPLINE_CURVE_WITH_KNOTS ( 'NONE', 3,
 ( #1334, #2487, #50921, #20491, #16059, #29329, #51217, #38487, #41759, #24914, #32877, #14881, #19913, #6028, #42933, #20204, #56504, #19329 ),
 .UNSPECIFIED., .F., .F.,
 ( 4, 2, 2, 2, 2, 2, 2, 2, 4 ),
 ( 0.000000000000000000, 0.1250000000000000278, 0.2500000000000000555, 0.3750000000000000000, 0.5000000000000000000, 0.6250000000000000000, 0.7500000000000000000, 0.8750000000000001110, 1.000000000000000000 ),
 .UNSPECIFIED. ) ;
#36932=( GEOMETRIC_REPRESENTATION_CONTEXT ( 3 ) GLOBAL_UNCERTAINTY_ASSIGNED_CONTEXT ( ( #51429 ) ) GLOBAL_UNIT_ASSIGNED_CONTEXT ( ( #40420, #31241, #45158 ) ) REPRESENTATION_CONTEXT ( 'NONE', 'WORKASPACE' ) );
#36933=CARTESIAN_POINT ( 'NONE',  ( 9.567317839327603934, -78.81236982575325101, -4.905351266707688396 ) ) ;
#36934=ORIENTED_EDGE ( 'NONE', *, *, #55333, .T. ) ;
#36935=CARTESIAN_POINT ( 'NONE',  ( 1.849737152796000039, -76.61177708502411576, 11.02961253863000124 ) ) ;
#36938=EDGE_CURVE ( 'NONE', #34885, #37074, #49332, .T. ) ;
#36940=CARTESIAN_POINT ( 'NONE',  ( -12.18072440915408450, -77.04494352351606778, 0.6797451543154154896 ) ) ;
#36941=CARTESIAN_POINT ( 'NONE',  ( 2.228715616918034215, -77.91001247118138906, 11.77084610582519453 ) ) ;
#36942=CARTESIAN_POINT ( 'NONE',  ( -5.394429334091999984, -79.91896985327970526, -9.834543342166998769 ) ) ;
#36943=CARTESIAN_POINT ( 'NONE',  ( 7.685486533051383518, -81.00000000000001421, 7.726202419513529485 ) ) ;
#36949=AXIS2_PLACEMENT_3D ( 'NONE', #41100, #23955, #14805 ) ;
#36953=CARTESIAN_POINT ( 'NONE',  ( -12.00000000000000000, -77.39999999999999147, 0.000000000000000000 ) ) ;
#36963=CARTESIAN_POINT ( 'NONE',  ( 9.696452258889999953, -75.92770142656900134, 4.797923606538000207 ) ) ;
#36964=CARTESIAN_POINT ( 'NONE',  ( 10.45679952538025503, -77.86866984986814089, 2.493435623531266021 ) ) ;
#36965=CARTESIAN_POINT ( 'NONE',  ( -3.085175050843000477, -78.17037848440200776, -11.57574012064000080 ) ) ;
#36967=AXIS2_PLACEMENT_3D ( 'NONE', #4979, #32405, #54582 ) ;
#36969=DIRECTION ( 'NONE',  ( 0.000000000000000000, 0.000000000000000000, -1.000000000000000000 ) ) ;
#36971=CARTESIAN_POINT ( 'NONE',  ( 3.981698583510459244, -80.94499118605105537, 9.985454001900388121 ) ) ;
#36974=CARTESIAN_POINT ( 'NONE',  ( -9.936460025306999455, -77.42856642211100393, -5.051867252445999767 ) ) ;
#36976=CARTESIAN_POINT ( 'NONE',  ( 9.669337410324999382, -80.66897452307009075, -5.298214362520000442 ) ) ;
#36980=CARTESIAN_POINT ( 'NONE',  ( -10.54491486739000017, -77.72600129843600314, -3.823987582478999947 ) ) ;
#36993=CARTESIAN_POINT ( 'NONE',  ( -6.043427764450832740, -77.71666666666666856, 10.48543666025107512 ) ) ;
#36996=CARTESIAN_POINT ( 'NONE',  ( -6.805157294386518174, -80.17080800408460561, -8.328756680024682169 ) ) ;
#36999=VERTEX_POINT ( 'NONE', #24794 ) ;
#37003=CARTESIAN_POINT ( 'NONE',  ( 2.005614507304999794, -80.09841179485169960, -10.84800649278999884 ) ) ;
#37021=ORIENTED_EDGE ( 'NONE', *, *, #21413, .T. ) ;
#37022=DIRECTION ( 'NONE',  ( 0.000000000000000000, -1.000000000000000000, 0.000000000000000000 ) ) ;
#37034=CARTESIAN_POINT ( 'NONE',  ( 11.14639666075000157, -81.00452969028360428, -1.632917082138999776 ) ) ;
#37035=VECTOR ( 'NONE', #918, 1000.000000000000000 ) ;
#37036=CARTESIAN_POINT ( 'NONE',  ( -3.140974612311405512, -76.69583333333332575, 11.68767212001977640 ) ) ;
#37039=CARTESIAN_POINT ( 'NONE',  ( 9.596002108778145967, -78.20208333333333428, 7.374560639699002884 ) ) ;
#37042=DIRECTION ( 'NONE',  ( -1.000000000000000000, 0.000000000000000000, 0.000000000000000000 ) ) ;
#37046=PLANE ( 'NONE',  #21147 ) ;
#37049=CARTESIAN_POINT ( 'NONE',  ( -1.743222555440693489, -79.48802005694665240, 10.60902930704550506 ) ) ;
#37054=CYLINDRICAL_SURFACE ( 'NONE', #18417, 10.75000000000000000 ) ;
#37058=LINE ( 'NONE', #13746, #3152 ) ;
#37064=CARTESIAN_POINT ( 'NONE',  ( -5.721970631177883071, -77.18051251777001198, -9.113473785769789615 ) ) ;
#37065=CARTESIAN_POINT ( 'NONE',  ( 6.365665562422999635, -79.13050366622999832, 10.17242851768000023 ) ) ;
#37068=CARTESIAN_POINT ( 'NONE',  ( -9.625846388754000671, -79.18507706297299364, -7.214584339064000318 ) ) ;
#37072=CARTESIAN_POINT ( 'NONE',  ( 9.113984702984998520, -77.92925969475899706, 7.705244011730999709 ) ) ;
#37074=VERTEX_POINT ( 'NONE', #3794 ) ;
#37076=CARTESIAN_POINT ( 'NONE',  ( -9.393203674808288994, -78.95833333333332860, 5.413904038987134015 ) ) ;
#37081=B_SPLINE_SURFACE_WITH_KNOTS ( 'NONE', 3, 3, ( 
 ( #46702, #1819, #19816, #20389, #38387, #11251, #56120, #16538, #7383, #30086, #33663, #47854, #56695, #3256, #52836, #34518, #52550, #12391, #12105, #56407, #29231, #21536, #25384, #43981, #56976, #7959, #2961, #7100, #29518, #47280, #48139, #42832, #15956, #43399, #29798 ),
 ( #11822, #33947, #57263, #7671, #30381, #51703, #6809, #20959, #15666, #38964, #43123, #52267, #24817, #16829, #51987, #20676, #21245, #25673, #2393, #34811, #43700, #39247, #48420, #25959, #3534, #11541, #47574, #25099, #2682, #38675, #16253, #34231, #9430, #36286, #12676 ),
 ( #4109, #17106, #16, #40424, #13844, #9136, #54308, #3820, #22111, #53127, #21822, #4997, #39825, #17396, #35093, #31843, #17994, #18292, #49885, #49287, #27419, #45455, #13552, #39541, #27121, #30952, #26827, #57547, #35381, #30667, #54011, #58133, #26250, #4409, #53406 ),
 ( #48991, #48705, #40120, #12956, #8248, #45161, #17698, #8536, #44265, #31544, #57839, #44557, #26530, #4710, #22709, #35688, #53715, #13252, #31245, #40722, #8838, #314, #44857, #22412, #35986, #49589, #886, #33006, #37743, #23002, #18870, #19163, #45753, #5286, #36574 ) ),
 .UNSPECIFIED., .F., .F., .F.,
 ( 4, 4 ),
 ( 4, 1, 1, 1, 1, 1, 1, 1, 1, 1, 1, 1, 1, 1, 1, 1, 1, 1, 1, 1, 1, 1, 1, 1, 1, 1, 1, 1, 1, 1, 1, 1, 4 ),
 ( -0.1772706441294000235, 1.177270644128999955 ),
 ( -0.01510644027126000107, 0.009441525169539000117, 0.03398949061033999797, 0.05853745605114000355, 0.08308542149195000115, 0.1076333869326999981, 0.1321813523735999862, 0.1567293178143999988, 0.1812772832552000113, 0.2058252486960000238, 0.2303732141367999808, 0.2549211795776000211, 0.2794691450183999781, 0.3040171104591999907, 0.3285650759000000032, 0.3531130413408000157, 0.3776610067816000282, 0.4022089722223999853, 0.4267569376631999978, 0.4513049031039999548, 0.4758528685447999673, 0.5004008339856000909, 0.5249487994264000479, 0.5494967648672000049, 0.5740447303079999619, 0.5985926957488000300, 0.6231406611895999870, 0.6476886266303999440, 0.6722365920712000120, 0.6967845575119999690, 0.7213325229527999261, 0.7458804883935999941, 0.7704284538343999511 ),
 .UNSPECIFIED. ) ;
#37090=CARTESIAN_POINT ( 'NONE',  ( 10.02574878253000001, -76.48484873660000005, 4.955627619753999902 ) ) ;
#37091=EDGE_CURVE ( 'NONE', #31953, #23662, #40697, .T. ) ;
#37108=CARTESIAN_POINT ( 'NONE',  ( 12.00000000000000000, -78.64999999999999147, 0.000000000000000000 ) ) ;
#37110=DIRECTION ( 'NONE',  ( -1.000000000000000000, 0.000000000000000000, 0.000000000000000000 ) ) ;
#37127=CARTESIAN_POINT ( 'NONE',  ( -11.40251694347999845, -80.77844001750112568, -0.2650480098012999997 ) ) ;
#37130=CARTESIAN_POINT ( 'NONE',  ( 8.196653188619999142, -77.71147621424999841, 7.657217973713000170 ) ) ;
#37136=CARTESIAN_POINT ( 'NONE',  ( -5.497476511162663115, -76.12291666666041579, 9.512467313639556110 ) ) ;
#37141=CARTESIAN_POINT ( 'NONE',  ( -11.26045488449999965, -80.69595964897830243, 0.3336940576009999604 ) ) ;
#37147=CARTESIAN_POINT ( 'NONE',  ( 2.739292792226000195, -77.90193793104199926, -11.85237552491999935 ) ) ;
#37155=AXIS2_PLACEMENT_3D ( 'NONE', #39706, #7553, #20834 ) ;
#37178=CARTESIAN_POINT ( 'NONE',  ( -6.620362748380999918, -76.14579926823699907, -10.34376132320999986 ) ) ;
#37179=DIRECTION ( 'NONE',  ( 0.7071067811865975328, -0.7071067811864976127, -4.006680953078982088E-09 ) ) ;
#37182=CARTESIAN_POINT ( 'NONE',  ( -9.735611069857000643, -79.20864007176808741, 5.570995215215999607 ) ) ;
#37183=EDGE_LOOP ( 'NONE', ( #1612, #56712, #56272, #52914 ) ) ;
#37189=CARTESIAN_POINT ( 'NONE',  ( -5.241653689492999924, -77.66540636460800329, -10.72196665943000049 ) ) ;
#37192=CARTESIAN_POINT ( 'NONE',  ( -2.772348231745000113, -79.13115782519599861, -10.55885653242000011 ) ) ;
#37193=CARTESIAN_POINT ( 'NONE',  ( 12.00000000000000000, -76.54999999999999716, 0.000000000000000000 ) ) ;
#37194=ORIENTED_EDGE ( 'NONE', *, *, #17429, .T. ) ;
#37196=CIRCLE ( 'NONE', #30605, 10.25000000000000000 ) ;
#37201=CARTESIAN_POINT ( 'NONE',  ( 3.245333607557999933, -76.22751663978100112, 12.07566914630000099 ) ) ;
#37204=CYLINDRICAL_SURFACE ( 'NONE', #8902, 11.70000000000000107 ) ;
#37207=CARTESIAN_POINT ( 'NONE',  ( 8.769046271958000460, -78.47261268016799818, -7.066663249742999753 ) ) ;
#37209=CARTESIAN_POINT ( 'NONE',  ( -1.407171709420465211, -79.88541666666665719, 10.74999999999999467 ) ) ;
#37216=CARTESIAN_POINT ( 'NONE',  ( 10.47020627418438643, -79.27083333333335702, 2.813789756862283387 ) ) ;
#37222=CARTESIAN_POINT ( 'NONE',  ( 10.19409538785635405, -78.82440253168712729, -3.416663174436564088 ) ) ;
#37225=CARTESIAN_POINT ( 'NONE',  ( 11.06808393496999976, -76.51144931706768659, 1.603559079323000347 ) ) ;
#37229=CARTESIAN_POINT ( 'NONE',  ( -10.47957108958864758, -76.59215066385610271, -6.245855599599564378 ) ) ;
#37230=CARTESIAN_POINT ( 'NONE',  ( -11.61470386271144584, -77.53020205524934738, 2.935752974902272161 ) ) ;
#37231=CARTESIAN_POINT ( 'NONE',  ( 9.376438147752001129, -79.46987249797800246, -6.156339679782000474 ) ) ;
#37233=ADVANCED_FACE ( 'NONE', ( #5544 ), #581, .T. ) ;
#37244=CARTESIAN_POINT ( 'NONE',  ( 12.00000000000000000, -78.64999999999999147, 0.000000000000000000 ) ) ;
#37255=CARTESIAN_POINT ( 'NONE',  ( -1.665424875009057004, -77.98744771326413172, 10.62927728148073214 ) ) ;
#37256=CARTESIAN_POINT ( 'NONE',  ( 1.720939166139000109, -77.27055478756399509, -11.69973432676000158 ) ) ;
#37260=CARTESIAN_POINT ( 'NONE',  ( 9.280195964196915170, -80.89241446635494981, 5.426651790427706068 ) ) ;
#37263=CARTESIAN_POINT ( 'NONE',  ( 7.081068198472000752, -77.27840274250999641, 8.459326660559002065 ) ) ;
#37264=CARTESIAN_POINT ( 'NONE',  ( -11.80208112488000083, -77.17229294297220576, -3.396125071686999952 ) ) ;
#37265=CARTESIAN_POINT ( 'NONE',  ( 10.97353685322999972, -80.65494283066439607, 1.923198805891999985 ) ) ;
#37269=CARTESIAN_POINT ( 'NONE',  ( -10.86658628928999981, -76.71825660736899977, -2.781249891074999869 ) ) ;
#37275=B_SPLINE_SURFACE_WITH_KNOTS ( 'NONE', 3, 3, ( 
 ( #21297, #43454, #17444, #29852, #16878, #26574, #22162, #52319, #12723, #43751, #3015, #3303, #57596, #39303, #57314, #25438, #53172, #39016, #52604, #44031, #26006, #11874, #48466, #34858, #3582, #21586, #8296, #57028, #48752, #40168, #47906, #16586, #7438, #34572, #31292 ),
 ( #27458, #14470, #50506, #22458, #28326, #14754, #33047, #10646, #28625, #46670, #42228, #39223, #39515, #57237, #47828, #30062, #48677, #53381, #12928, #39797, #16224, #25644, #7359, #8506, #25358, #20933, #20650, #17369, #43373, #17081, #43670, #57520, #21792, #30925, #35062 ),
 ( #34494, #30351, #35355, #38935, #57810, #53099, #3228, #30642, #12649, #44238, #56952, #52523, #48112, #48963, #21508, #12362, #21216, #16801, #7644, #34785, #48394, #43099, #8221, #2932, #26222, #3791, #25931, #2656, #52810, #38650, #16511, #52240, #56668, #34204, #12080 ),
 ( #11796, #7931, #29772, #43958, #3506, #22382, #36257, #4079, #27391, #40985, #18556, #14110, #54278, #32107, #40087, #13815, #27094, #27680, #23267, #45724, #5259, #18843, #36836, #40393, #14395, #53683, #31815, #17666, #35653, #13221, #31216, #58402, #49856, #49254, #8806 ) ),
 .UNSPECIFIED., .F., .F., .F.,
 ( 4, 4 ),
 ( 4, 1, 1, 1, 1, 1, 1, 1, 1, 1, 1, 1, 1, 1, 1, 1, 1, 1, 1, 1, 1, 1, 1, 1, 1, 1, 1, 1, 1, 1, 1, 1, 4 ),
 ( -0.1772706441294000235, 1.177270644128999955 ),
 ( 0.4993183012519999964, 0.5152713945944999985, 0.5312244879369000250, 0.5471775812793999716, 0.5631306746219000292, 0.5790837679642999447, 0.5950368613068000023, 0.6109899546492000288, 0.6269430479917000865, 0.6428961413342000331, 0.6588492346765999486, 0.6748023280191000062, 0.6907554213615000327, 0.7067085147039999793, 0.7226616080465000369, 0.7386147013889000634, 0.7545677947314000100, 0.7705208880737999255, 0.7864739814162999831, 0.8024270747588000408, 0.8183801681012000673, 0.8343332614437000139, 0.8502863547860999294, 0.8662394481285999870, 0.8821925414711000446, 0.8981456348135000711, 0.9140987281560000177, 0.9300518214983999332, 0.9460049148408999908, 0.9619580081833999374, 0.9779111015257999640, 0.9938641948683000216, 1.009817288211000141 ),
 .UNSPECIFIED. ) ;
#37288=CARTESIAN_POINT ( 'NONE',  ( -7.599722349268615673, -80.16297892688153581, -7.602663284551876011 ) ) ;
#37294=CARTESIAN_POINT ( 'NONE',  ( -7.286644543156999276, -79.52644859181400250, -8.282906837769999697 ) ) ;
#37312=FACE_OUTER_BOUND ( 'NONE', #18066, .T. ) ;
#37313=CARTESIAN_POINT ( 'NONE',  ( 4.336551063001058637, -77.05429869360747830, -11.23466680206521850 ) ) ;
#37315=ADVANCED_FACE ( 'NONE', ( #47762 ), #39874, .T. ) ;
#37320=CARTESIAN_POINT ( 'NONE',  ( -10.98749645531777830, -77.33354319426250356, -4.929334125398810329 ) ) ;
#37327=CARTESIAN_POINT ( 'NONE',  ( 11.02326530841000007, -81.09238336756219212, 1.187788371667000131 ) ) ;
#37328=DIRECTION ( 'NONE',  ( -0.7071067811864976127, 0.7071067811865975328, 1.669581477361993759E-09 ) ) ;
#37334=CARTESIAN_POINT ( 'NONE',  ( 7.374560639698954922, -78.22291666666667709, 9.596002108778179718 ) ) ;
#37345=CARTESIAN_POINT ( 'NONE',  ( 10.44234272621953608, -79.36931961362199672, 2.576411631240690614 ) ) ;
#37362=CARTESIAN_POINT ( 'NONE',  ( 11.92746894621999942, -79.39426247890499155, 1.562891678063999867 ) ) ;
#37365=ORIENTED_EDGE ( 'NONE', *, *, #57193, .T. ) ;
#37366=CARTESIAN_POINT ( 'NONE',  ( -9.654076420390000024, -78.17342353357300055, -7.016716533807999312 ) ) ;
#37380=CARTESIAN_POINT ( 'NONE',  ( 10.47020627418439531, -80.72916666666667140, -2.813789756862242974 ) ) ;
#37383=CARTESIAN_POINT ( 'NONE',  ( -10.74969614785317340, -80.09697912524651997, 0.4764947645818390920 ) ) ;
#37385=CARTESIAN_POINT ( 'NONE',  ( -5.007180289739999068, -76.67804699982200134, 10.00009952528999868 ) ) ;
#37390=DIRECTION ( 'NONE',  ( -1.000000000000000000, 0.000000000000000000, 0.000000000000000000 ) ) ;
#37394=DIRECTION ( 'NONE',  ( 0.000000000000000000, -1.000000000000000000, 0.000000000000000000 ) ) ;
#37402=CARTESIAN_POINT ( 'NONE',  ( -12.00000000000000000, -77.29999999999999716, 0.000000000000000000 ) ) ;
#37409=CARTESIAN_POINT ( 'NONE',  ( 11.65296779515999859, -77.59787174848798941, -3.873515295708999773 ) ) ;
#37415=EDGE_CURVE ( 'NONE', #35080, #51790, #14421, .T. ) ;
#37417=CARTESIAN_POINT ( 'NONE',  ( 9.852601822233998163, -80.56860390147939199, 5.745770655690999540 ) ) ;
#37421=CARTESIAN_POINT ( 'NONE',  ( -9.998780405325002008, -77.43911278423200883, -5.083552005986999411 ) ) ;
#37429=CARTESIAN_POINT ( 'NONE',  ( -0.9849936891751999157, -80.81635039299281686, -11.22225356808999841 ) ) ;
#37439=CARTESIAN_POINT ( 'NONE',  ( -12.14750708673999924, -78.25461903155100174, 0.6485384821269000177 ) ) ;
#37464=CARTESIAN_POINT ( 'NONE',  ( 3.090997446795999970, -77.27913901744200587, -11.88544462247999967 ) ) ;
#37469=CARTESIAN_POINT ( 'NONE',  ( 4.038993597075479336, -78.40481902541532122, -10.27651239117697557 ) ) ;
#37476=CARTESIAN_POINT ( 'NONE',  ( 0.3849455888886000321, -77.20420800240398762, -11.69935108946000035 ) ) ;
#37482=ORIENTED_EDGE ( 'NONE', *, *, #25391, .T. ) ;
#37483=EDGE_CURVE ( 'NONE', #14498, #27418, #50701, .T. ) ;
#37494=CARTESIAN_POINT ( 'NONE',  ( -10.38493632045999959, -78.74497611018699672, 4.357414620914999759 ) ) ;
#37495=CARTESIAN_POINT ( 'NONE',  ( 4.904027517709028672, -76.51100935185411345, -10.05130150382343679 ) ) ;
#37496=CARTESIAN_POINT ( 'NONE',  ( 8.348814612957056625, -79.73768109752721500, -8.297071948231263150 ) ) ;
#37502=CARTESIAN_POINT ( 'NONE',  ( -7.408952625746029419, -79.41749330375276372, -8.421937422778746907 ) ) ;
#37510=CARTESIAN_POINT ( 'NONE',  ( -12.00000000000000355, -77.28958333333331154, 1.570796326794848596 ) ) ;
#37513=DIRECTION ( 'NONE',  ( 0.000000000000000000, 0.000000000000000000, -1.000000000000000000 ) ) ;
#37514=CARTESIAN_POINT ( 'NONE',  ( 6.653919560569870661, -78.77822032348952064, -8.445832356448455869 ) ) ;
#37517=CARTESIAN_POINT ( 'NONE',  ( 1.546553306619000256, -76.38603960712254093, -11.07619323538000344 ) ) ;
#37520=CARTESIAN_POINT ( 'NONE',  ( -6.471588721810545231, -76.62988340216107019, -10.34169530630836320 ) ) ;
#37521=CARTESIAN_POINT ( 'NONE',  ( 10.18080324349809729, -78.34408151796235131, 6.314367479422754670 ) ) ;
#37522=CARTESIAN_POINT ( 'NONE',  ( 7.910349975595998728, -79.57881786998500218, 7.952639426948999279 ) ) ;
#37531=CARTESIAN_POINT ( 'NONE',  ( 11.68767212001979239, -77.62916666666667709, -3.140974612311342451 ) ) ;
#37545=CARTESIAN_POINT ( 'NONE',  ( 10.45259816626330007, -77.86880115736309449, 2.510970294598007690 ) ) ;
#37546=CARTESIAN_POINT ( 'NONE',  ( -6.777984382448000389, -78.14324916897800222, -9.878005474088999094 ) ) ;
#37548=CARTESIAN_POINT ( 'NONE',  ( 10.75000000000000000, -78.85000000000000853, 0.000000000000000000 ) ) ;
#37551=CARTESIAN_POINT ( 'NONE',  ( 10.75000000000000000, -80.84999999999999432, -1.053639850055999980E-14 ) ) ;
#37554=CARTESIAN_POINT ( 'NONE',  ( -8.507210620304000770, -78.01378400355899601, -7.023467935662000450 ) ) ;
#37555=CARTESIAN_POINT ( 'NONE',  ( 1.808018834342399295, -77.28683563664310441, -11.88153690539541074 ) ) ;
#37556=CARTESIAN_POINT ( 'NONE',  ( -6.315983860361000346, -80.60246315746479695, -8.896737291152998495 ) ) ;
#37565=CARTESIAN_POINT ( 'NONE',  ( -9.302864017704999711, -76.81328150364699070, -6.266965030821000759 ) ) ;
#37574=CARTESIAN_POINT ( 'NONE',  ( 1.514497777301999859, -77.64085666695899590, 11.15976079676000055 ) ) ;
#37587=CARTESIAN_POINT ( 'NONE',  ( 9.953654131039998632, -79.74433933582800194, 4.756732473150000473 ) ) ;
#37588=DIRECTION ( 'NONE',  ( 0.000000000000000000, -1.000000000000000000, 1.958765290093000082E-13 ) ) ;
#37593=B_SPLINE_CURVE_WITH_KNOTS ( 'NONE', 3,
 ( #53145, #52858, #13783, #30403, #18525, #21556, #9373, #7980, #25977, #4656 ),
 .UNSPECIFIED., .F., .F.,
 ( 4, 2, 2, 2, 4 ),
 ( 0.000000000000000000, 0.2500000000000000555, 0.5000000000000001110, 0.7500000000000002220, 1.000000000000000000 ),
 .UNSPECIFIED. ) ;
#37613=CARTESIAN_POINT ( 'NONE',  ( 5.246383657897999875, -77.46100733245999947, -10.79237965019999912 ) ) ;
#37618=CARTESIAN_POINT ( 'NONE',  ( -12.00000000000000000, -76.79999999999999716, 1.164316068523999942E-14 ) ) ;
#37624=CARTESIAN_POINT ( 'NONE',  ( 3.140974612311326908, -78.25416666666664867, 11.68767212001979772 ) ) ;
#37635=CONICAL_SURFACE ( 'NONE', #49916, 10.29999999990999981, 0.7853981633972997312 ) ;
#37638=CARTESIAN_POINT ( 'NONE',  ( -1.268951038218919747, -79.48456372641344103, 10.67475623963393083 ) ) ;
#37643=EDGE_CURVE ( 'NONE', #56437, #28871, #37058, .T. ) ;
#37653=CARTESIAN_POINT ( 'NONE',  ( 6.842135374053461838, -80.28010575421185990, -8.291310720910153975 ) ) ;
#37658=CARTESIAN_POINT ( 'NONE',  ( -0.9103933733443999587, -79.75286604907600463, -11.99492895764000089 ) ) ;
#37662=CARTESIAN_POINT ( 'NONE',  ( 8.241770352740999783, -78.30907011069199086, -8.631843597936001089 ) ) ;
#37671=B_SPLINE_CURVE_WITH_KNOTS ( 'NONE', 3,
 ( #21059, #39060, #57074, #56503, #15762, #29328, #56792, #11639, #2486, #16636, #6615, #16058, #20203, #28746, #6905, #25197, #16352, #34332 ),
 .UNSPECIFIED., .F., .F.,
 ( 4, 2, 2, 2, 2, 2, 2, 2, 4 ),
 ( 0.000000000000000000, 0.1250000000000000000, 0.2499999999999999722, 0.3750000000000000000, 0.5000000000000000000, 0.6250000000000000000, 0.7500000000000000000, 0.8750000000000000000, 1.000000000000000000 ),
 .UNSPECIFIED. ) ;
#37673=ORIENTED_EDGE ( 'NONE', *, *, #13106, .F. ) ;
#37676=VECTOR ( 'NONE', #41793, 1000.000000000000114 ) ;
#37677=CARTESIAN_POINT ( 'NONE',  ( -8.653929927890716911, -79.80000000000001137, -8.194783130391765980 ) ) ;
#37682=CARTESIAN_POINT ( 'NONE',  ( 8.332845033087998843, -75.89124277619099246, -7.273191856730000460 ) ) ;
#37686=FACE_OUTER_BOUND ( 'NONE', #1508, .T. ) ;
#37694=CARTESIAN_POINT ( 'NONE',  ( 3.496086695581000381, -79.86073619718679595, 11.68876967166999847 ) ) ;
#37695=CARTESIAN_POINT ( 'NONE',  ( -9.886815349277940257, -78.06793176728791650, 4.222132225938193706 ) ) ;
#37699=CARTESIAN_POINT ( 'NONE',  ( 9.596002108778145967, -79.20208333333333428, 7.374560639699002884 ) ) ;
#37713=CARTESIAN_POINT ( 'NONE',  ( 11.27907281578000109, -80.95552175511359394, -0.4739325926940000100 ) ) ;
#37716=CARTESIAN_POINT ( 'NONE',  ( -6.984027423104000043, -77.33016741222499491, 8.777327129872999123 ) ) ;
#37721=DIRECTION ( 'NONE',  ( 0.000000000000000000, 1.000000000000000000, 2.010360378377999880E-13 ) ) ;
#37726=CARTESIAN_POINT ( 'NONE',  ( 10.70339364929999881, -80.96683882301098834, 2.537196166659999808 ) ) ;
#37728=ORIENTED_EDGE ( 'NONE', *, *, #36908, .T. ) ;
#37732=CARTESIAN_POINT ( 'NONE',  ( 0.3960817336853000303, -77.45420800240398762, -12.03780325391999995 ) ) ;
#37734=CARTESIAN_POINT ( 'NONE',  ( 9.838187006391597933, -78.71594490248966736, -4.482782177594915041 ) ) ;
#37740=CARTESIAN_POINT ( 'NONE',  ( -8.596574492439220450, -77.65209465126851285, -6.606491961039523630 ) ) ;
#37743=CARTESIAN_POINT ( 'NONE',  ( -6.595392621385999909, -76.20310294825600295, -10.30474759485999847 ) ) ;
#37744=CARTESIAN_POINT ( 'NONE',  ( 1.984688374631000007, -79.71295766602599997, -10.73482082212999877 ) ) ;
#37758=CARTESIAN_POINT ( 'NONE',  ( -10.75000000000000000, -77.50000000000000000, 0.000000000000000000 ) ) ;
#37763=CARTESIAN_POINT ( 'NONE',  ( -8.598496321198998871, -77.19717354083199723, -8.768570137950998600 ) ) ;
#37767=CARTESIAN_POINT ( 'NONE',  ( 2.179295889402999897, -78.60944052572851604, 11.00312592022000047 ) ) ;
#37769=ORIENTED_EDGE ( 'NONE', *, *, #49057, .F. ) ;
#37772=DIRECTION ( 'NONE',  ( -1.000000000000000000, 0.000000000000000000, 0.000000000000000000 ) ) ;
#37775=CARTESIAN_POINT ( 'NONE',  ( 7.822091542723999424, -77.25846663325098973, -9.013910121987001034 ) ) ;
#37792=CARTESIAN_POINT ( 'NONE',  ( 10.63213186872000016, -78.49984902316998614, -3.713725309742000213 ) ) ;
#37810=CARTESIAN_POINT ( 'NONE',  ( 9.076269682406973516, -78.80512772263888621, -5.761168607463022617 ) ) ;
#37816=CARTESIAN_POINT ( 'NONE',  ( 0.4155002556947535730, -76.17709054250207146, -12.19260400794555821 ) ) ;
#37818=CARTESIAN_POINT ( 'NONE',  ( 4.899921843424915657, -78.20843494084340364, -10.93209756983152658 ) ) ;
#37819=CARTESIAN_POINT ( 'NONE',  ( 2.315902194296999728, -78.47544367418299771, -10.97517055051999968 ) ) ;
#37823=ORIENTED_EDGE ( 'NONE', *, *, #26612, .T. ) ;
#37826=CARTESIAN_POINT ( 'NONE',  ( 1.633433878009751483, -77.98653774450133369, -11.09745478611874425 ) ) ;
#37839=CARTESIAN_POINT ( 'NONE',  ( -12.00000000000000178, -79.41041666666664867, -1.570796326794897668 ) ) ;
#37843=CARTESIAN_POINT ( 'NONE',  ( 9.789819849890999848, -78.76722342372499952, -6.904744247936999813 ) ) ;
#37845=CIRCLE ( 'NONE', #24670, 13.89999999999999858 ) ;
#37850=CARTESIAN_POINT ( 'NONE',  ( -10.58794861553789346, -76.58625634654212888, 1.859587138064856315 ) ) ;
#37851=CARTESIAN_POINT ( 'NONE',  ( 10.90309719880000117, -77.19669371350400411, -1.680537371260999890 ) ) ;
#37853=CARTESIAN_POINT ( 'NONE',  ( -7.374560639698971798, -78.37291666666666856, -9.596002108778163731 ) ) ;
#37858=CARTESIAN_POINT ( 'NONE',  ( 11.01642476345000077, -77.03117224766199911, 2.111041454437999842 ) ) ;
#37863=CARTESIAN_POINT ( 'NONE',  ( -11.74310723221000075, -76.06594802940500699, 1.595441940087999999 ) ) ;
#37872=CARTESIAN_POINT ( 'NONE',  ( -3.140974612311405512, -77.69583333333332575, 11.68767212001977640 ) ) ;
#37880=CARTESIAN_POINT ( 'NONE',  ( -2.665716224216999830, -79.85328470783530008, 10.70493771085999946 ) ) ;
#37883=ORIENTED_EDGE ( 'NONE', *, *, #3241, .F. ) ;
#37904=CARTESIAN_POINT ( 'NONE',  ( -11.99999999999999822, -77.30670863885249844, -1.011638905658493126 ) ) ;
#37911=CARTESIAN_POINT ( 'NONE',  ( 12.00000000000000000, -77.14999999999999147, 0.000000000000000000 ) ) ;
#37915=CARTESIAN_POINT ( 'NONE',  ( 10.48543666025108045, -78.19166666666664867, 6.043427764450817641 ) ) ;
#37928=CARTESIAN_POINT ( 'NONE',  ( -1.154578316665619164, -79.48373165137867602, 10.68778363297984058 ) ) ;
#37938=LINE ( 'NONE', #1086, #3877 ) ;
#37940=CARTESIAN_POINT ( 'NONE',  ( 7.705541234979771836, -80.28859837433554958, -7.495979100088282721 ) ) ;
#37942=CARTESIAN_POINT ( 'NONE',  ( -10.46839011967282040, -77.12114419157363443, -2.819731185745065538 ) ) ;
#37947=CARTESIAN_POINT ( 'NONE',  ( 9.785129497364000173, -79.33449521720999087, -6.997026981537000090 ) ) ;
#37951=CARTESIAN_POINT ( 'NONE',  ( 6.420671964385999964, -77.79361311763999254, -10.06034164291999922 ) ) ;
#37954=CARTESIAN_POINT ( 'NONE',  ( -5.413904038987206846, -78.91666666666665719, 9.393203674808249914 ) ) ;
#37966=CARTESIAN_POINT ( 'NONE',  ( 10.72073260548720874, -79.79999999999999716, 4.953289013571211541 ) ) ;
#37968=B_SPLINE_CURVE_WITH_KNOTS ( 'NONE', 3,
 ( #26026, #39038, #8609, #40191, #35754, #44054, #39611, #57615, #35160, #55229, #32482, #13912, #40780, #27183, #1235, #37216, #4771, #23643 ),
 .UNSPECIFIED., .F., .F.,
 ( 4, 2, 2, 2, 2, 2, 2, 2, 4 ),
 ( 0.000000000000000000, 0.1250000000000000000, 0.2500000000000000000, 0.3750000000000000000, 0.5000000000000000000, 0.6250000000000000000, 0.7500000000000000000, 0.8750000000000000000, 1.000000000000000000 ),
 .UNSPECIFIED. ) ;
#37970=CARTESIAN_POINT ( 'NONE',  ( -10.67244467921999984, -76.88050928501199621, 2.904229794498999873 ) ) ;
#37971=CARTESIAN_POINT ( 'NONE',  ( 6.384645922588179090, -76.42558410655975365, 8.681868184700029190 ) ) ;
#37974=CARTESIAN_POINT ( 'NONE',  ( -9.979434319869000092, -76.78551456381899243, 5.147272234993000239 ) ) ;
#37981=CARTESIAN_POINT ( 'NONE',  ( -11.80615446477999875, -79.05949749041099039, 2.575676343767999921 ) ) ;
#37982=CARTESIAN_POINT ( 'NONE',  ( 6.268664514307507929, -76.25703125000501359, 10.22525207047880258 ) ) ;
#37999=CARTESIAN_POINT ( 'NONE',  ( 5.088741150401000723, -79.97850485460629955, 9.946204611282000840 ) ) ;
#38002=CARTESIAN_POINT ( 'NONE',  ( 7.508079800428999917, -77.08504032520899329, -8.333477563431999968 ) ) ;
#38011=CARTESIAN_POINT ( 'NONE',  ( -10.75000000000000000, -80.00000000000000000, 0.000000000000000000 ) ) ;
#38012=DIRECTION ( 'NONE',  ( 0.000000000000000000, 1.000000000000000000, 0.000000000000000000 ) ) ;
#38022=CARTESIAN_POINT ( 'NONE',  ( 10.73158301355000077, -77.61698389494598871, 5.968995448363000556 ) ) ;
#38024=CARTESIAN_POINT ( 'NONE',  ( -2.787250405516429996, -77.49586229219684697, 10.40630179466836225 ) ) ;
#38034=ORIENTED_EDGE ( 'NONE', *, *, #39411, .T. ) ;
#38036=CARTESIAN_POINT ( 'NONE',  ( -7.105843098096999988, -79.00481274797898834, 8.287482117959999783 ) ) ;
#38053=CARTESIAN_POINT ( 'NONE',  ( -11.94395460750000204, -77.11520806422198859, 2.857367593729999822 ) ) ;
#38056=CARTESIAN_POINT ( 'NONE',  ( 11.14115696400000033, -78.99074932775353375, -1.301050381412999890 ) ) ;
#38066=CARTESIAN_POINT ( 'NONE',  ( -4.817132589604000259, -78.53373690646100158, -11.17039677886999982 ) ) ;
#38071=CARTESIAN_POINT ( 'NONE',  ( -10.74525019809999904, -79.51246662722100211, 1.927424232126999870 ) ) ;
#38083=CARTESIAN_POINT ( 'NONE',  ( 5.260169723461094904, -79.38792388839776493, 10.53050267336613999 ) ) ;
#38092=B_SPLINE_CURVE_WITH_KNOTS ( 'NONE', 3,
 ( #10805, #29081, #9924, #5483 ),
 .UNSPECIFIED., .F., .F.,
 ( 4, 4 ),
 ( 0.000000000000000000, 1.000000000000000000 ),
 .UNSPECIFIED. ) ;
#38101=CARTESIAN_POINT ( 'NONE',  ( 2.208636725687457059, -78.74160535473284028, -10.52059596911941952 ) ) ;
#38107=CARTESIAN_POINT ( 'NONE',  ( 6.586108526242999694, -80.17391735373439587, 8.810401493720998900 ) ) ;
#38109=CARTESIAN_POINT ( 'NONE',  ( -9.066796825632000179, -78.88398881921099814, -6.603885667862000375 ) ) ;
#38115=CARTESIAN_POINT ( 'NONE',  ( -8.729826100308692105, -77.79588334348935064, 7.043560550046861657 ) ) ;
#38123=CARTESIAN_POINT ( 'NONE',  ( 3.577370205891725163, -79.79961842550528672, -11.19231790377194713 ) ) ;
#38125=VERTEX_POINT ( 'NONE', #49643 ) ;
#38126=CARTESIAN_POINT ( 'NONE',  ( 12.00000000000000711, -79.63958333333333428, -1.570796326794872355 ) ) ;
#38128=CARTESIAN_POINT ( 'NONE',  ( 9.002946773217001208, -76.07771018338799252, 6.708522467097999709 ) ) ;
#38129=CARTESIAN_POINT ( 'NONE',  ( 8.098714463133978470, -79.29284371306400203, -7.103727516995692604 ) ) ;
#38130=CARTESIAN_POINT ( 'NONE',  ( -1.360213228908000005, -77.74983936004998952, -11.90234785270000017 ) ) ;
#38138=CARTESIAN_POINT ( 'NONE',  ( -9.149418163674001292, -77.00603931249200684, -6.163594735446999984 ) ) ;
#38139=CARTESIAN_POINT ( 'NONE',  ( -8.034660013930000844, -81.08572150553020208, -7.381588020910998971 ) ) ;
#38147=CARTESIAN_POINT ( 'NONE',  ( -6.659967121051000305, -76.84051784664899287, -9.025682433062998555 ) ) ;
#38151=CARTESIAN_POINT ( 'NONE',  ( -11.21131451355000053, -77.04216005809600176, -4.985388207940000704 ) ) ;
#38160=CARTESIAN_POINT ( 'NONE',  ( 7.374560639698993114, -79.47708333333332575, -9.596002108778149520 ) ) ;
#38166=ORIENTED_EDGE ( 'NONE', *, *, #17045, .F. ) ;
#38172=ORIENTED_EDGE ( 'NONE', *, *, #37643, .T. ) ;
#38178=ORIENTED_EDGE ( 'NONE', *, *, #40419, .T. ) ;
#38186=CARTESIAN_POINT ( 'NONE',  ( 7.629353270364749307, -76.29218750007841265, -7.631376092477169415 ) ) ;
#38190=CARTESIAN_POINT ( 'NONE',  ( -9.699999999837999098, -87.69999999983798489, -3.624872775666000097E-09 ) ) ;
#38191=EDGE_CURVE ( 'NONE', #22103, #4693, #11807, .T. ) ;
#38203=CARTESIAN_POINT ( 'NONE',  ( -9.596002108778193929, -77.34791666666663446, 7.374560639698937159 ) ) ;
#38210=CARTESIAN_POINT ( 'NONE',  ( -3.527598694514999966, -78.42305673476900552, -10.69532371905999923 ) ) ;
#38216=CONICAL_SURFACE ( 'NONE', #58014, 9.649999999909001147, 0.7853981633972997312 ) ;
#38223=CARTESIAN_POINT ( 'NONE',  ( 0.2531623955774147117, -79.47320930135717276, 10.74994997524480311 ) ) ;
#38229=CARTESIAN_POINT ( 'NONE',  ( -0.9453041629244000044, -78.09062011958100413, 11.10679974661999836 ) ) ;
#38231=DIRECTION ( 'NONE',  ( 1.000000000000000000, 0.000000000000000000, 0.000000000000000000 ) ) ;
#38237=CARTESIAN_POINT ( 'NONE',  ( 3.552363299575000077, -79.71496112664699751, -11.49294985030999960 ) ) ;
#38242=CARTESIAN_POINT ( 'NONE',  ( -4.070249838183999991, -78.52610463408198882, 11.21911621747999810 ) ) ;
#38243=ORIENTED_EDGE ( 'NONE', *, *, #11767, .F. ) ;
#38257=CARTESIAN_POINT ( 'NONE',  ( 1.941355800891735761, -79.80000000000001137, -11.64207563132269740 ) ) ;
#38259=CARTESIAN_POINT ( 'NONE',  ( -5.514935242309477736, -80.01815905343127611, 9.228334353175002391 ) ) ;
#38262=CARTESIAN_POINT ( 'NONE',  ( -9.831705185582000794, -76.29436059729400199, 5.330239850318999828 ) ) ;
#38267=CARTESIAN_POINT ( 'NONE',  ( 11.02258233089000150, -76.05813824613500174, -2.141614703964000110 ) ) ;
#38272=CARTESIAN_POINT ( 'NONE',  ( 8.958886133240000049, -79.26804927549699187, -8.109116339278001462 ) ) ;
#38273=EDGE_CURVE ( 'NONE', #45906, #31098, #24090, .T. ) ;
#38274=CARTESIAN_POINT ( 'NONE',  ( -8.024340789631628112, -78.04212779903014052, 7.157226290975113869 ) ) ;
#38279=CARTESIAN_POINT ( 'NONE',  ( 11.68767212001978173, -79.17083333333336270, 3.140974612311388192 ) ) ;
#38283=CARTESIAN_POINT ( 'NONE',  ( 0.000000000000000000, -90.39999999999999147, 0.000000000000000000 ) ) ;
#38288=ORIENTED_EDGE ( 'NONE', *, *, #14771, .F. ) ;
#38296=CARTESIAN_POINT ( 'NONE',  ( -8.729704736439998669, -77.84765792925898609, 7.043462628994999974 ) ) ;
#38302=EDGE_LOOP ( 'NONE', ( #44254, #27048, #1602, #38172, #6636 ) ) ;
#38313=CARTESIAN_POINT ( 'NONE',  ( 9.596418076563999477, -77.95619656188999613, -7.476047798475000228 ) ) ;
#38320=EDGE_LOOP ( 'NONE', ( #23225, #39117, #30533 ) ) ;
#38322=CARTESIAN_POINT ( 'NONE',  ( 2.253937565478000060, -78.21495880092599862, -10.68151722998999986 ) ) ;
#38324=CARTESIAN_POINT ( 'NONE',  ( -1.407276357456320737, -80.71461996621154356, -10.68035269161679146 ) ) ;
#38330=CARTESIAN_POINT ( 'NONE',  ( 6.917788961651000434, -78.82398876163412638, -9.780606322222999083 ) ) ;
#38339=CARTESIAN_POINT ( 'NONE',  ( -11.80208112487999905, -77.15619080252700712, -3.396125071686999952 ) ) ;
#38349=CYLINDRICAL_SURFACE ( 'NONE', #32343, 14.00000000000000000 ) ;
#38350=CARTESIAN_POINT ( 'NONE',  ( 9.404538367153101319, -78.70366911081997330, 7.521839627124905725 ) ) ;
#38352=CARTESIAN_POINT ( 'NONE',  ( -10.02269271100999859, -77.46203272307600685, 6.688901441487999477 ) ) ;
#38356=CARTESIAN_POINT ( 'NONE',  ( 2.120986319506000140, -78.88603073817900224, 10.70872462160000005 ) ) ;
#38357=CARTESIAN_POINT ( 'NONE',  ( -10.60025282971301763, -79.58684258122036681, 1.788823804082396940 ) ) ;
#38366=CARTESIAN_POINT ( 'NONE',  ( 1.570796326794910547, -78.03541666666666288, -11.99999999999999822 ) ) ;
#38369=CARTESIAN_POINT ( 'NONE',  ( -4.036005110416000186, -79.18075759821599036, 10.51402051105999824 ) ) ;
#38370=CARTESIAN_POINT ( 'NONE',  ( -10.31421052434999908, -76.82175206120300004, 3.823226550887000030 ) ) ;
#38371=CARTESIAN_POINT ( 'NONE',  ( -3.848761171412311999, -79.14836415611753750, -11.19148989879134248 ) ) ;
#38376=CARTESIAN_POINT ( 'NONE',  ( 11.05000000000000071, -81.00000000000000000, 0.000000000000000000 ) ) ;
#38387=CARTESIAN_POINT ( 'NONE',  ( -8.813874136147999749, -77.38986986081299335, -8.988208014853000805 ) ) ;
#38388=CARTESIAN_POINT ( 'NONE',  ( -4.372067062227771750, -78.69186267950118463, -9.823263076180332121 ) ) ;
#38399=CARTESIAN_POINT ( 'NONE',  ( -10.71602610194999805, -79.81002448127239290, 3.314346869870000489 ) ) ;
#38400=ORIENTED_EDGE ( 'NONE', *, *, #54062, .T. ) ;
#38404=CARTESIAN_POINT ( 'NONE',  ( -10.31421052434999908, -76.82175206120300004, 3.823226550887000030 ) ) ;
#38405=CARTESIAN_POINT ( 'NONE',  ( 8.282422341201556293, -78.04101043050533804, -7.564594445558528335 ) ) ;
#38415=CARTESIAN_POINT ( 'NONE',  ( 11.66950233118999947, -79.38048444465056264, -2.920592611544999606 ) ) ;
#38422=CARTESIAN_POINT ( 'NONE',  ( 4.458743082292000004, -77.41075765253599172, 11.11915799896999957 ) ) ;
#38427=CARTESIAN_POINT ( 'NONE',  ( 10.68871602397163301, -80.85933999195634669, 1.217520377858459346 ) ) ;
#38430=CARTESIAN_POINT ( 'NONE',  ( -0.8117802668354000550, -77.57800251553000237, -11.00194288205000070 ) ) ;
#38431=CARTESIAN_POINT ( 'NONE',  ( 10.47020627418439531, -79.22916666666665719, -2.813789756862242974 ) ) ;
#38432=CARTESIAN_POINT ( 'NONE',  ( -8.904870325259999220, -80.57561547146119096, -6.304511959018999967 ) ) ;
#38434=VERTEX_POINT ( 'NONE', #34795 ) ;
#38440=CARTESIAN_POINT ( 'NONE',  ( -0.9512330062464999791, -78.14786231073598799, 11.17646036812999988 ) ) ;
#38452=CARTESIAN_POINT ( 'NONE',  ( -9.596002108778161954, -76.85208333333332575, -7.374560639698982456 ) ) ;
#38462=B_SPLINE_CURVE_WITH_KNOTS ( 'NONE', 3,
 ( #51690, #46223, #36173, #28170 ),
 .UNSPECIFIED., .F., .F.,
 ( 4, 4 ),
 ( 0.000000000000000000, 1.000000000000000000 ),
 .UNSPECIFIED. ) ;
#38464=VERTEX_POINT ( 'NONE', #30362 ) ;
#38470=CARTESIAN_POINT ( 'NONE',  ( -9.359443164323526076, -81.00000000000002842, -5.435958517830047576 ) ) ;
#38487=CARTESIAN_POINT ( 'NONE',  ( -3.140974612311405512, -76.79583333333332007, 11.68767212001977640 ) ) ;
#38491=B_SPLINE_CURVE_WITH_KNOTS ( 'NONE', 3,
 ( #18005, #55697, #24103, #31553 ),
 .UNSPECIFIED., .F., .F.,
 ( 4, 4 ),
 ( 0.000000000000000000, 1.000000000000000000 ),
 .UNSPECIFIED. ) ;
#38498=CARTESIAN_POINT ( 'NONE',  ( -9.599999999999999645, -87.59999999999999432, 0.000000000000000000 ) ) ;
#38507=EDGE_CURVE ( 'NONE', #13166, #10604, #12089, .T. ) ;
#38511=CARTESIAN_POINT ( 'NONE',  ( -5.413709697356376083, -77.01682545481338593, 9.392928511438244144 ) ) ;
#38520=CARTESIAN_POINT ( 'NONE',  ( 7.110505486850000167, -78.39021989260101009, -8.302835368086999068 ) ) ;
#38526=CARTESIAN_POINT ( 'NONE',  ( 7.163861093844410277, -80.28312376644485937, -8.015740724809139905 ) ) ;
#38530=CARTESIAN_POINT ( 'NONE',  ( 11.90415444617999974, -79.73682346591400005, -1.731350929957999885 ) ) ;
#38532=CARTESIAN_POINT ( 'NONE',  ( 9.414214675708999280, -79.52717617799699212, -6.181142822975999707 ) ) ;
#38549=CARTESIAN_POINT ( 'NONE',  ( -1.293105744743758390, -79.79999999999998295, -11.73994710747565229 ) ) ;
#38550=CARTESIAN_POINT ( 'NONE',  ( -7.786690763151178807, -80.03945749923617825, 7.436444533740759866 ) ) ;
#38554=CARTESIAN_POINT ( 'NONE',  ( 7.995633008690000487, -76.64550778514200147, 7.819446035993999899 ) ) ;
#38558=CARTESIAN_POINT ( 'NONE',  ( -4.975971545690999420, -76.80307774425399714, 9.937770923463000727 ) ) ;
#38564=CARTESIAN_POINT ( 'NONE',  ( -0.4688094130881000354, -79.13080494938900245, -12.19136368054000030 ) ) ;
#38565=CARTESIAN_POINT ( 'NONE',  ( -10.63638328646205977, -78.08841358195864757, 1.565909971404836787 ) ) ;
#38574=CARTESIAN_POINT ( 'NONE',  ( 4.484526869169066288, -79.14462836071079721, 11.18137712903838299 ) ) ;
#38576=DIRECTION ( 'NONE',  ( 0.000000000000000000, 0.000000000000000000, -1.000000000000000000 ) ) ;
#38577=DIRECTION ( 'NONE',  ( -1.000000000000000000, 0.000000000000000000, 0.000000000000000000 ) ) ;
#38583=CARTESIAN_POINT ( 'NONE',  ( -11.03620408507000050, -80.26607873772769608, -2.260839449595000161 ) ) ;
#38591=CARTESIAN_POINT ( 'NONE',  ( 2.042564453799718294, -79.96020142208192283, 10.55469377556154242 ) ) ;
#38593=EDGE_CURVE ( 'NONE', #36429, #26795, #50312, .T. ) ;
#38595=CARTESIAN_POINT ( 'NONE',  ( 10.70940577679425409, -77.34266587486128230, -1.002872783366832499 ) ) ;
#38603=CARTESIAN_POINT ( 'NONE',  ( 2.974124060854000273, -79.04598695555699805, 11.51680281503000103 ) ) ;
#38614=CARTESIAN_POINT ( 'NONE',  ( 9.849799932654001111, -79.35888520700200388, 4.707101791649999534 ) ) ;
#38623=CARTESIAN_POINT ( 'NONE',  ( 7.494231858469171392, -80.53311548344800030, -8.337931667626193644 ) ) ;
#38624=CARTESIAN_POINT ( 'NONE',  ( -7.615853692923001184, -78.57982492282013709, 9.247423260716001181 ) ) ;
#38635=CARTESIAN_POINT ( 'NONE',  ( 3.140974612311377090, -77.94583333333332575, -11.68767212001978528 ) ) ;
#38643=CARTESIAN_POINT ( 'NONE',  ( 3.299676814977999584, -78.58799553730899845, -11.70874303878999889 ) ) ;
#38650=CARTESIAN_POINT ( 'NONE',  ( -6.534644050777999702, -79.11178473073800888, 10.11388646907000144 ) ) ;
#38654=LINE ( 'NONE', #42232, #16646 ) ;
#38660=CARTESIAN_POINT ( 'NONE',  ( 11.42348641225163242, -79.32084716335937458, 3.093858311050987631 ) ) ;
#38670=FACE_OUTER_BOUND ( 'NONE', #20466, .T. ) ;
#38675=CARTESIAN_POINT ( 'NONE',  ( -11.02398976105000017, -76.29757433877699668, -5.829948365135000365 ) ) ;
#38676=CARTESIAN_POINT ( 'NONE',  ( 0.01553455395726060714, -78.72521037431218360, -10.74994277546958266 ) ) ;
#38684=CARTESIAN_POINT ( 'NONE',  ( -0.7036264152036126873, -79.71981223434178787, -10.74968282753707882 ) ) ;
#38687=CARTESIAN_POINT ( 'NONE',  ( 8.733858618705999888, -78.52991636018700206, -7.038306768505999678 ) ) ;
#38692=EDGE_CURVE ( 'NONE', #21820, #10829, #53113, .T. ) ;
#38696=CARTESIAN_POINT ( 'NONE',  ( -5.859527123903457202, -77.76864700048736267, 9.564912485122741614 ) ) ;
#38713=CARTESIAN_POINT ( 'NONE',  ( 11.70594025892000012, -78.26536582366799166, 2.546964289010999583 ) ) ;
#38718=CARTESIAN_POINT ( 'NONE',  ( -10.75000000000000000, -76.59999999999999432, 0.000000000000000000 ) ) ;
#38719=CARTESIAN_POINT ( 'NONE',  ( 4.161322419204999790, -77.18271174891199848, -10.09251018087000062 ) ) ;
#38720=CARTESIAN_POINT ( 'NONE',  ( 6.606377239730347739, -79.17708333333331439, -8.596418555780422466 ) ) ;
#38727=AXIS2_PLACEMENT_3D ( 'NONE', #51897, #19724, #47192 ) ;
#38728=CARTESIAN_POINT ( 'NONE',  ( -2.185791986076000004, -77.94328743399398718, -11.00183730042999919 ) ) ;
#38732=CARTESIAN_POINT ( 'NONE',  ( 3.154088538942999786, -76.43069783301999109, 11.73615235293999959 ) ) ;
#38759=CARTESIAN_POINT ( 'NONE',  ( -9.731251526955000841, -77.11083935769899256, -4.947535720883000643 ) ) ;
#38763=CARTESIAN_POINT ( 'NONE',  ( 3.632329907060999563, -80.04667739574479413, 10.45854222826000068 ) ) ;
#38765=ORIENTED_EDGE ( 'NONE', *, *, #44288, .F. ) ;
#38781=CARTESIAN_POINT ( 'NONE',  ( -0.7928179559538000021, -78.82141258400598360, -11.95355612866999984 ) ) ;
#38788=CARTESIAN_POINT ( 'NONE',  ( 7.183928826236000376, -78.50476576377499782, -8.388570749380001246 ) ) ;
#38809=CARTESIAN_POINT ( 'NONE',  ( -9.398554024959999253, -78.25403817759199399, -5.993477931829000127 ) ) ;
#38815=CARTESIAN_POINT ( 'NONE',  ( 10.12305140789450775, -80.32185189037265616, -3.763052347616244742 ) ) ;
#38816=CARTESIAN_POINT ( 'NONE',  ( 9.238233337088816555, -79.89317385683257555, 5.558906132332217531 ) ) ;
#38819=CARTESIAN_POINT ( 'NONE',  ( -11.60111135005000094, -79.08740487884900006, -3.181408645392000523 ) ) ;
#38821=CARTESIAN_POINT ( 'NONE',  ( 11.18604332926000033, -79.06415834696599632, -1.306292155029999957 ) ) ;
#38822=ORIENTED_EDGE ( 'NONE', *, *, #30439, .T. ) ;
#38840=CARTESIAN_POINT ( 'NONE',  ( -4.848317728770459745, -80.01234159837389370, 9.594520772546756504 ) ) ;
#38842=CARTESIAN_POINT ( 'NONE',  ( 10.02574878253000001, -76.62042584315300076, 4.955627619753999902 ) ) ;
#38845=CARTESIAN_POINT ( 'NONE',  ( 10.95125797090999953, -76.62750415032999740, -1.894616286183999909 ) ) ;
#38852=CARTESIAN_POINT ( 'NONE',  ( -5.072986942693556323, -78.01416854347621666, 9.477675060726154399 ) ) ;
#38865=EDGE_CURVE ( 'NONE', #44663, #21904, #25305, .T. ) ;
#38870=CARTESIAN_POINT ( 'NONE',  ( -10.58783149161999759, -80.77773939978943929, -3.847989116766000084 ) ) ;
#38871=CARTESIAN_POINT ( 'NONE',  ( -5.845697796373999999, -80.35876778545760146, -9.793643869219998521 ) ) ;
#38877=CARTESIAN_POINT ( 'NONE',  ( -1.587769864458760338, -79.98724231797385187, 10.63181754089058373 ) ) ;
#38880=CARTESIAN_POINT ( 'NONE',  ( 9.448596496680870871, -77.31041241042555612, -5.152684619491262552 ) ) ;
#38899=VERTEX_POINT ( 'NONE', #40930 ) ;
#38908=CARTESIAN_POINT ( 'NONE',  ( 10.99419336675999936, -78.93250602332912536, 4.758540471090999979 ) ) ;
#38916=CARTESIAN_POINT ( 'NONE',  ( 9.406806676749999596, -76.69275178953499505, -7.895227358184000899 ) ) ;
#38926=CARTESIAN_POINT ( 'NONE',  ( -11.99726733138999890, -77.51629135392300896, -1.123097615067000010 ) ) ;
#38932=ORIENTED_EDGE ( 'NONE', *, *, #16967, .T. ) ;
#38933=CARTESIAN_POINT ( 'NONE',  ( -11.29698467241381188, -78.87175061103830842, 4.184771565250527736 ) ) ;
#38935=CARTESIAN_POINT ( 'NONE',  ( -1.790564795957000133, -79.80425913277389327, -11.90740541383000028 ) ) ;
#38947=CARTESIAN_POINT ( 'NONE',  ( -8.199429518657952443, -78.98546353816666965, 8.534060759012747965 ) ) ;
#38958=CARTESIAN_POINT ( 'NONE',  ( 9.392816810221818358, -78.39167583925791405, 5.413628547907069155 ) ) ;
#38962=EDGE_CURVE ( 'NONE', #26643, #616, #5790, .T. ) ;
#38964=CARTESIAN_POINT ( 'NONE',  ( 2.587846633264999863, -77.11722910487598881, 12.19916123416999909 ) ) ;
#38965=CARTESIAN_POINT ( 'NONE',  ( 3.614530024087561522, -78.75232390936722027, -10.13845990724425938 ) ) ;
#38973=CARTESIAN_POINT ( 'NONE',  ( -8.596678438649716369, -79.65211059969949758, -6.606629847258154165 ) ) ;
#38976=CARTESIAN_POINT ( 'NONE',  ( -10.34326456654000026, -78.80227979020500584, 4.339929572939999147 ) ) ;
#38979=DIRECTION ( 'NONE',  ( 1.000000000000000000, 0.000000000000000000, 0.000000000000000000 ) ) ;
#38985=CARTESIAN_POINT ( 'NONE',  ( -2.309498544611330750, -77.74141065748534629, 10.97669464986000420 ) ) ;
#38992=CARTESIAN_POINT ( 'NONE',  ( 5.137083998358000336, -77.31100733245999379, -10.56753840748999984 ) ) ;
#38999=EDGE_LOOP ( 'NONE', ( #642, #96 ) ) ;
#39002=CARTESIAN_POINT ( 'NONE',  ( -11.59999999999999964, -90.29999999999999716, 0.000000000000000000 ) ) ;
#39003=CARTESIAN_POINT ( 'NONE',  ( -5.261498566940000288, -77.65492149134999522, -10.76255997729999869 ) ) ;
#39004=CARTESIAN_POINT ( 'NONE',  ( -12.00000000000000000, -77.39999999999999147, 0.000000000000000000 ) ) ;
#39010=CARTESIAN_POINT ( 'NONE',  ( -10.73439844295906731, -76.59513923058339913, 0.6615022803101073823 ) ) ;
#39016=CARTESIAN_POINT ( 'NONE',  ( 12.17932748403999987, -79.56684242973399535, -1.499464232310999900 ) ) ;
#39019=CARTESIAN_POINT ( 'NONE',  ( 11.19952915612999966, -78.07946914900300328, -0.6234238306063999424 ) ) ;
#39022=DIRECTION ( 'NONE',  ( 0.000000000000000000, 1.000000000000000000, 0.000000000000000000 ) ) ;
#39023=CARTESIAN_POINT ( 'NONE',  ( 9.176121104939999995, -76.88349069267898983, 7.967706572806000587 ) ) ;
#39027=CARTESIAN_POINT ( 'NONE',  ( -8.150086036219999386, -78.58228563835899649, 7.434906319739000402 ) ) ;
#39033=CARTESIAN_POINT ( 'NONE',  ( -6.043427764450786555, -76.88333333333332575, -10.48543666025110177 ) ) ;
#39038=CARTESIAN_POINT ( 'NONE',  ( -10.75000000000000355, -79.48958333333334281, 1.407171709420384609 ) ) ;
#39047=CARTESIAN_POINT ( 'NONE',  ( 10.78933672403999999, -76.81123958467900081, -1.663003020634000073 ) ) ;
#39050=CARTESIAN_POINT ( 'NONE',  ( -5.394429334091999984, -79.78339274672698878, -9.834543342166998769 ) ) ;
#39060=CARTESIAN_POINT ( 'NONE',  ( 10.75000000000000355, -76.73958333333331439, -1.407171709420407035 ) ) ;
#39071=CARTESIAN_POINT ( 'NONE',  ( 9.148490208346998998, -78.00753312129299388, 7.734416031130999514 ) ) ;
#39073=EDGE_CURVE ( 'NONE', #47139, #21820, #32915, .T. ) ;
#39079=CARTESIAN_POINT ( 'NONE',  ( 7.538328940029000336, -77.00676689867499647, -8.367052130149000178 ) ) ;
#39081=CARTESIAN_POINT ( 'NONE',  ( 5.516100435859000228, -80.15765279019329625, 9.811525831467001524 ) ) ;
#39098=CARTESIAN_POINT ( 'NONE',  ( 3.831242997621999713, -76.98791202109900667, 10.34520717408000046 ) ) ;
#39105=CARTESIAN_POINT ( 'NONE',  ( 0.4840504722130451465, -80.22894859189042904, -10.73925919085179359 ) ) ;
#39107=CARTESIAN_POINT ( 'NONE',  ( 10.49326040991128828, -80.07116553579604101, -3.963973988046216146 ) ) ;
#39117=ORIENTED_EDGE ( 'NONE', *, *, #57844, .F. ) ;
#39119=FACE_OUTER_BOUND ( 'NONE', #16597, .T. ) ;
#39123=ORIENTED_EDGE ( 'NONE', *, *, #5039, .F. ) ;
#39128=CARTESIAN_POINT ( 'NONE',  ( -8.615032359022308128, -80.04915988844547314, 6.429856405177485357 ) ) ;
#39132=CARTESIAN_POINT ( 'NONE',  ( -1.963210506780999953, -76.44485224922898681, -11.00998129987999974 ) ) ;
#39136=CARTESIAN_POINT ( 'NONE',  ( -8.025391215536000544, -76.45193055640599766, -7.688479554171000707 ) ) ;
#39144=CARTESIAN_POINT ( 'NONE',  ( -0.3097977128257069501, -80.97757901313826778, 10.75868109506080472 ) ) ;
#39147=CARTESIAN_POINT ( 'NONE',  ( 12.00000000000000000, -79.14999999999999147, 0.000000000000000000 ) ) ;
#39151=CARTESIAN_POINT ( 'NONE',  ( -9.134410136912352485, -79.24350122207665947, 7.854726423800818758 ) ) ;
#39160=CARTESIAN_POINT ( 'NONE',  ( -1.123310606857000016, -80.39374047146120006, -11.35014609800000152 ) ) ;
#39177=VERTEX_POINT ( 'NONE', #33796 ) ;
#39180=DIRECTION ( 'NONE',  ( 1.155082973713999823E-13, 0.000000000000000000, 1.000000000000000000 ) ) ;
#39182=ORIENTED_EDGE ( 'NONE', *, *, #7238, .T. ) ;
#39192=CARTESIAN_POINT ( 'NONE',  ( 4.311778524607963625, -80.50626779744442274, -10.34858355512559314 ) ) ;
#39200=CARTESIAN_POINT ( 'NONE',  ( 1.298131932841000147, -76.36488988309598369, 12.21218573294999921 ) ) ;
#39211=CARTESIAN_POINT ( 'NONE',  ( 3.113245456484129203, -78.46450137413576442, -10.55002948983070610 ) ) ;
#39214=CARTESIAN_POINT ( 'NONE',  ( -8.607099856842999941, -77.57054998477100582, -8.432888219828999610 ) ) ;
#39215=DIRECTION ( 'NONE',  ( 0.000000000000000000, 1.000000000000000000, 0.000000000000000000 ) ) ;
#39220=CARTESIAN_POINT ( 'NONE',  ( -6.837720798360027885, -79.52994970263227970, 8.297335093543503959 ) ) ;
#39222=CARTESIAN_POINT ( 'NONE',  ( -9.134410136912348932, -78.84350122207662537, 7.854726423800818758 ) ) ;
#39223=CARTESIAN_POINT ( 'NONE',  ( -3.764285624315000245, -79.65891715040700660, 11.55877412955000061 ) ) ;
#39239=ORIENTED_EDGE ( 'NONE', *, *, #34951, .T. ) ;
#39247=CARTESIAN_POINT ( 'NONE',  ( 1.318177213333999953, -76.62543624521698860, 12.40076185704000089 ) ) ;
#39248=CARTESIAN_POINT ( 'NONE',  ( 4.145023818608256860, -78.75651719028334696, -9.918724640339455334 ) ) ;
#39260=CARTESIAN_POINT ( 'NONE',  ( -11.12496554189999820, -77.26019399548486888, -1.432917402686000097 ) ) ;
#39263=CARTESIAN_POINT ( 'NONE',  ( -7.408849624938999234, -79.46926788952099230, -8.421820339245000397 ) ) ;
#39285=CARTESIAN_POINT ( 'NONE',  ( 8.596418555780418913, -77.80208333333332860, 6.606377239730356621 ) ) ;
#39290=CARTESIAN_POINT ( 'NONE',  ( 11.36821324764999908, -77.79056806846899974, -3.778861202892000115 ) ) ;
#39298=CARTESIAN_POINT ( 'NONE',  ( 12.00000000000000000, -78.54999999999999716, 0.000000000000000000 ) ) ;
#39303=CARTESIAN_POINT ( 'NONE',  ( 4.260122498627000098, -79.67337695312400569, 11.50807400234999989 ) ) ;
#39307=CARTESIAN_POINT ( 'NONE',  ( -7.803863155890000236, -78.27012355001599531, 8.057160196619001624 ) ) ;
#39310=CARTESIAN_POINT ( 'NONE',  ( 5.970850396337000099, -76.17430707708200543, -10.71897758064000072 ) ) ;
#39315=CARTESIAN_POINT ( 'NONE',  ( -10.57985553746999940, -78.66399466736399404, -3.125442558719000008 ) ) ;
#39337=EDGE_CURVE ( 'NONE', #33152, #8440, #1643, .T. ) ;
#39338=CARTESIAN_POINT ( 'NONE',  ( -9.888452460216527129, -81.00000000000000000, -4.376188563388549113 ) ) ;
#39339=CARTESIAN_POINT ( 'NONE',  ( 10.89235442234000040, -77.32873010171299200, 0.7293703643125000191 ) ) ;
#39344=CARTESIAN_POINT ( 'NONE',  ( 8.733858618705999888, -78.39433925363499611, -7.038306768505999678 ) ) ;
#39345=ORIENTED_EDGE ( 'NONE', *, *, #51577, .F. ) ;
#39346=ORIENTED_EDGE ( 'NONE', *, *, #42083, .T. ) ;
#39363=AXIS2_PLACEMENT_3D ( 'NONE', #12002, #11717, #29694 ) ;
#39365=CARTESIAN_POINT ( 'NONE',  ( 11.97742283006000186, -77.95327449044499701, 0.2395971301470999903 ) ) ;
#39371=FILL_AREA_STYLE ('',( #43516 ) ) ;
#39373=CARTESIAN_POINT ( 'NONE',  ( -10.03906427447999938, -77.36083935769899256, -5.104033018226999729 ) ) ;
#39375=CARTESIAN_POINT ( 'NONE',  ( 4.427954972153999691, -80.98098182763799002, -10.19376387942000051 ) ) ;
#39377=CARTESIAN_POINT ( 'NONE',  ( 8.779106447692145210, -80.29927823582293911, 6.259569139016127437 ) ) ;
#39391=B_SPLINE_SURFACE_WITH_KNOTS ( 'NONE', 3, 3, ( 
 ( #8474, #44493, #49525, #18810, #28522, #6095, #9954, #41238, #10838, #37090, #24104, #32648, #1690, #19682, #46571, #42124, #55401, #36801, #10539, #15246, #543, #54819, #55108, #23233, #829, #14078, #18519, #19393, #10243, #32946, #36512, #50700, #1114, #37682, #55698 ),
 ( #54537, #32362, #27935, #32072, #37385, #23520, #33240, #14361, #50113, #51284, #45688, #28814, #46862, #6390, #45984, #24405, #9658, #27647, #5228, #50404, #14653, #5510, #41531, #14948, #19099, #28223, #46277, #5803, #23809, #41825, #1399, #50988, #51575, #43572, #20269 ),
 ( #20836, #11132, #3135, #34401, #29970, #29681, #34106, #25267, #38554, #38842, #56569, #47156, #29396, #48021, #52720, #12272, #39132, #15541, #24976, #6686, #7839, #24694, #38262, #19983, #16708, #56859, #21126, #30261, #52148, #57143, #48301, #16419, #34690, #7555, #33822 ),
 ( #11992, #37970, #42999, #56285, #25553, #51862, #47446, #42420, #52432, #11706, #2556, #20557, #6974, #16129, #47731, #1989, #55995, #42705, #33538, #29110, #43286, #2272, #7266, #15835, #11415, #2840, #43869, #49465, #26133, #4583, #54180, #18167, #13126, #30839, #12838 ) ),
 .UNSPECIFIED., .F., .F., .F.,
 ( 4, 4 ),
 ( 4, 1, 1, 1, 1, 1, 1, 1, 1, 1, 1, 1, 1, 1, 1, 1, 1, 1, 1, 1, 1, 1, 1, 1, 1, 1, 1, 1, 1, 1, 1, 1, 4 ),
 ( -0.5168282991433000850, 1.516828299142999992 ),
 ( -0.009208997693793000497, 0.005755623558620999794, 0.02072024481102999888, 0.03568486606345000478, 0.05064948731585999786, 0.06561410856827000482, 0.08057872982069000378, 0.09554335107309999686, 0.1105079723255000118, 0.1254725935778999990, 0.1404372148303000001, 0.1554018360827999767, 0.1703664573352000056, 0.1853310785876000066, 0.2002956998400000077, 0.2152603210924000088, 0.2302249423447999821, 0.2451895635972000109, 0.2601541848496000120, 0.2751188061020999887, 0.2900834273544999897, 0.3050480486068999908, 0.3200126698593000474, 0.3349772911116999929, 0.3499419123640999940, 0.3649065336164999951, 0.3798711548689999717, 0.3948357761214000283, 0.4098003973737999739, 0.4247650186261999750, 0.4397296398786000315, 0.4546942611309999771, 0.4696588823833999782 ),
 .UNSPECIFIED. ) ;
#39392=CARTESIAN_POINT ( 'NONE',  ( -10.00926467875000014, -76.60660321907299419, 4.638537167971000130 ) ) ;
#39397=CARTESIAN_POINT ( 'NONE',  ( -5.625515643987146319, -80.18124105601512497, -9.161514280032365676 ) ) ;
#39399=CARTESIAN_POINT ( 'NONE',  ( 7.910459948463299362, -79.66262039076877954, 7.952749987741428939 ) ) ;
#39401=CARTESIAN_POINT ( 'NONE',  ( 11.92746894621999942, -79.25868537235298561, 1.562891678063999867 ) ) ;
#39411=EDGE_CURVE ( 'NONE', #23438, #30600, #52540, .T. ) ;
#39420=ORIENTED_EDGE ( 'NONE', *, *, #45014, .T. ) ;
#39424=CARTESIAN_POINT ( 'NONE',  ( -6.937102608493817435, -80.03119389196088207, 8.211835529152839541 ) ) ;
#39430=CARTESIAN_POINT ( 'NONE',  ( 5.402466744453000125, -76.15846601409100458, 9.843631583929999707 ) ) ;
#39442=CARTESIAN_POINT ( 'NONE',  ( 9.393203674808258796, -80.20833333333331439, -5.413904038987190859 ) ) ;
#39460=CARTESIAN_POINT ( 'NONE',  ( -2.184012626508494481, -79.99174196189673580, 10.52796603406774700 ) ) ;
#39497=CARTESIAN_POINT ( 'NONE',  ( -10.51110168222999874, -75.95506250004599735, 6.351495789100000344 ) ) ;
#39506=CARTESIAN_POINT ( 'NONE',  ( -9.933360547807000174, -77.92342353357300055, -7.219704108085999827 ) ) ;
#39512=CARTESIAN_POINT ( 'NONE',  ( -7.601746409728754372, -79.53766441201359783, 7.600897104933312498 ) ) ;
#39515=CARTESIAN_POINT ( 'NONE',  ( 0.2413473483368999972, -79.63228351955899598, 12.15388238791999953 ) ) ;
#39517=DIRECTION ( 'NONE',  ( 0.000000000000000000, 1.000000000000000000, 0.000000000000000000 ) ) ;
#39523=ORIENTED_EDGE ( 'NONE', *, *, #39073, .F. ) ;
#39537=EDGE_CURVE ( 'NONE', #46988, #36429, #40110, .T. ) ;
#39541=CARTESIAN_POINT ( 'NONE',  ( 11.20283039713999962, -76.47574370419398804, 5.204271411707000361 ) ) ;
#39542=CARTESIAN_POINT ( 'NONE',  ( -8.098901191184470605, -78.65749706134158714, -7.103902919008961092 ) ) ;
#39550=CARTESIAN_POINT ( 'NONE',  ( -3.633103876187999681, -77.15124862347786916, 10.61219425078000000 ) ) ;
#39553=CARTESIAN_POINT ( 'NONE',  ( -2.848564863371000122, -79.00625005849099125, -10.84913769893999991 ) ) ;
#39554=ADVANCED_FACE ( 'NONE', ( #53706 ), #7661, .T. ) ;
#39579=CARTESIAN_POINT ( 'NONE',  ( 10.18066396183999878, -78.29249513909199720, 6.314281093748000728 ) ) ;
#39582=CARTESIAN_POINT ( 'NONE',  ( -10.57592698605000159, -78.61493240443898856, -5.530395178621999364 ) ) ;
#39586=CARTESIAN_POINT ( 'NONE',  ( 7.374560639698993114, -78.47708333333332575, -9.596002108778149520 ) ) ;
#39594=CARTESIAN_POINT ( 'NONE',  ( 2.854969924326999919, -78.18841452101000300, 10.84745395576000071 ) ) ;
#39597=CARTESIAN_POINT ( 'NONE',  ( 11.48358316434000059, -76.28750529199700736, 4.321443532648999941 ) ) ;
#39601=CARTESIAN_POINT ( 'NONE',  ( 6.766101950298000212, -78.96359444038398578, 8.713300108436000002 ) ) ;
#39611=CARTESIAN_POINT ( 'NONE',  ( -5.413904038987206846, -79.41666666666665719, 9.393203674808249914 ) ) ;
#39615=ORIENTED_EDGE ( 'NONE', *, *, #5230, .T. ) ;
#39616=ORIENTED_EDGE ( 'NONE', *, *, #9082, .T. ) ;
#39617=CARTESIAN_POINT ( 'NONE',  ( 10.54482503192156173, -78.83451348532614134, -2.089947448372381000 ) ) ;
#39622=CARTESIAN_POINT ( 'NONE',  ( 7.007185918478000097, -76.89294861368399836, 8.371063940391000102 ) ) ;
#39625=CARTESIAN_POINT ( 'NONE',  ( -1.472820794058999905, -78.31263022462898959, -10.90095403661999995 ) ) ;
#39642=CARTESIAN_POINT ( 'NONE',  ( -7.248874762069000610, -79.65039421481900206, -9.668155108506001127 ) ) ;
#39645=CARTESIAN_POINT ( 'NONE',  ( 2.228685126279000173, -78.06179175213999599, 11.77068507108999995 ) ) ;
#39654=CARTESIAN_POINT ( 'NONE',  ( 9.707899084501001141, -77.11571227068199619, 5.708822989341999943 ) ) ;
#39655=CARTESIAN_POINT ( 'NONE',  ( -10.48543666025111420, -78.25833333333331154, 6.043427764450754580 ) ) ;
#39656=FACE_OUTER_BOUND ( 'NONE', #10703, .T. ) ;
#39662=CARTESIAN_POINT ( 'NONE',  ( -0.9512330062464999791, -78.08007375745999923, 11.17646036812999988 ) ) ;
#39663=CARTESIAN_POINT ( 'NONE',  ( 10.20077725957859371, -76.87621043607762772, 3.463738954154604421 ) ) ;
#39671=CARTESIAN_POINT ( 'NONE',  ( -6.618456890295999706, -76.78327565549400902, -8.969427176287000592 ) ) ;
#39677=CARTESIAN_POINT ( 'NONE',  ( -0.7043158906892222904, -80.21985320402481534, -10.73277725065178245 ) ) ;
#39678=CARTESIAN_POINT ( 'NONE',  ( -8.596418555780431348, -77.05208333333332860, -6.606377239730338857 ) ) ;
#39680=CARTESIAN_POINT ( 'NONE',  ( 11.66950233118999947, -79.29659029478199272, -2.920592611544999606 ) ) ;
#39683=CARTESIAN_POINT ( 'NONE',  ( 3.521285801175999985, -79.17310371897299603, 10.69740673549999954 ) ) ;
#39685=ORIENTED_EDGE ( 'NONE', *, *, #51577, .T. ) ;
#39693=CARTESIAN_POINT ( 'NONE',  ( 0.000000000000000000, -75.15999999999999659, 0.000000000000000000 ) ) ;
#39695=CARTESIAN_POINT ( 'NONE',  ( -2.637902738039999750, -79.46783057900900360, 10.59324478783000067 ) ) ;
#39706=CARTESIAN_POINT ( 'NONE',  ( 0.000000000000000000, -90.29999999999999716, 0.000000000000000000 ) ) ;
#39711=CARTESIAN_POINT ( 'NONE',  ( 7.285770374979999353, -76.21115555539499553, -7.844054078469000046 ) ) ;
#39720=CARTESIAN_POINT ( 'NONE',  ( -5.059370734576000395, -80.98961836681789350, -10.06538451635999998 ) ) ;
#39727=AXIS2_PLACEMENT_3D ( 'NONE', #46643, #6171, #24181 ) ;
#39735=CARTESIAN_POINT ( 'NONE',  ( -7.960542989054001595, -80.68744634177852504, 7.971132368775000643 ) ) ;
#39738=CARTESIAN_POINT ( 'NONE',  ( 6.043427764450807871, -79.06666666666666288, -10.48543666025108756 ) ) ;
#39741=CARTESIAN_POINT ( 'NONE',  ( -2.424017749977676051, -79.99353046406088197, 10.47610573998703742 ) ) ;
#39768=CARTESIAN_POINT ( 'NONE',  ( -10.80752097171290416, -80.82844002948797879, 2.980286201706882743 ) ) ;
#39778=CARTESIAN_POINT ( 'NONE',  ( 0.03250568004163000707, -75.87309702343600293, 11.74995503739000036 ) ) ;
#39781=CARTESIAN_POINT ( 'NONE',  ( 1.418826352046264949, -78.23560893958142515, -10.68831118249899426 ) ) ;
#39786=CARTESIAN_POINT ( 'NONE',  ( 3.791268666074999683, -77.37336614992500472, 10.23726759892000082 ) ) ;
#39788=CARTESIAN_POINT ( 'NONE',  ( 7.972949129781999211, -77.12301250442499168, -9.187753233325999247 ) ) ;
#39793=CARTESIAN_POINT ( 'NONE',  ( -9.134412046857288914, -79.55589225187523539, 5.669345810953543285 ) ) ;
#39796=CARTESIAN_POINT ( 'NONE',  ( 6.365665562422999635, -78.73050366622999263, 10.17242851768000023 ) ) ;
#39797=CARTESIAN_POINT ( 'NONE',  ( 8.539931521643000067, -79.44584810362599114, -8.651281711199999336 ) ) ;
#39798=CARTESIAN_POINT ( 'NONE',  ( -5.666459946039999807, -80.15558659221879623, -9.493356078915999419 ) ) ;
#39799=CARTESIAN_POINT ( 'NONE',  ( 12.00000000000000000, -79.65624999999998579, 0.9424777960769732399 ) ) ;
#39813=ORIENTED_EDGE ( 'NONE', *, *, #49245, .F. ) ;
#39817=ORIENTED_EDGE ( 'NONE', *, *, #35451, .T. ) ;
#39825=CARTESIAN_POINT ( 'NONE',  ( 12.14581882086999975, -76.92655382554799814, -2.250985356504000112 ) ) ;
#39827=CARTESIAN_POINT ( 'NONE',  ( -9.532031226582633465, -78.63842284804186988, -4.970339354283964894 ) ) ;
#39834=CARTESIAN_POINT ( 'NONE',  ( -11.14038684213999630, -78.24070234355004061, 1.307628137226999998 ) ) ;
#39837=CARTESIAN_POINT ( 'NONE',  ( -10.71602610194999805, -79.87781303454870852, 3.314346869870000489 ) ) ;
#39856=CIRCLE ( 'NONE', #3096, 11.05000000000000071 ) ;
#39862=FACE_OUTER_BOUND ( 'NONE', #1721, .T. ) ;
#39866=CARTESIAN_POINT ( 'NONE',  ( -1.828203654226000063, -77.96382883426899468, 11.79377691179999843 ) ) ;
#39874=CONICAL_SURFACE ( 'NONE', #8775, 11.80312499993000053, 0.7853981633972997312 ) ;
#39881=CARTESIAN_POINT ( 'NONE',  ( 9.325195487021998630, -76.70256541335099598, -7.974226357216999794 ) ) ;
#39885=CARTESIAN_POINT ( 'NONE',  ( -11.13698119474000059, -79.71223007984299613, -0.4714344481541999921 ) ) ;
#39889=DIRECTION ( 'NONE',  ( 0.000000000000000000, 0.7071067811866525998, -0.7071067811864425456 ) ) ;
#39892=CARTESIAN_POINT ( 'NONE',  ( 12.27743704900000132, -78.07818225714999016, 0.2455986337158999888 ) ) ;
#39907=CARTESIAN_POINT ( 'NONE',  ( -0.9355429176084000265, -78.02289305516799800, 10.99211052673000033 ) ) ;
#39911=CARTESIAN_POINT ( 'NONE',  ( -0.2291600886666000092, -78.32170900562999805, -11.06898422383999936 ) ) ;
#39928=CARTESIAN_POINT ( 'NONE',  ( 8.704926853273999399, -78.81797727176099500, 7.993911894783999550 ) ) ;
#39930=CARTESIAN_POINT ( 'NONE',  ( -7.614885234455580409, -78.03764472252724715, 7.587876194577269473 ) ) ;
#39931=CARTESIAN_POINT ( 'NONE',  ( -11.86109855473999986, -78.64510676903400110, -1.682380905046999997 ) ) ;
#39938=CARTESIAN_POINT ( 'NONE',  ( -11.16978667388999824, -77.33360301469699039, -1.438690452479999937 ) ) ;
#39940=CARTESIAN_POINT ( 'NONE',  ( -9.186543509187998779, -80.37243427822239994, -6.503932264059000268 ) ) ;
#39948=CARTESIAN_POINT ( 'NONE',  ( 6.201912463541000342, -78.37059474947899673, -9.171216270948999494 ) ) ;
#39954=AXIS2_PLACEMENT_3D ( 'NONE', #40668, #32659, #10251 ) ;
#39960=CARTESIAN_POINT ( 'NONE',  ( 8.315675604772998497, -77.96769278298098982, -7.594965687514999786 ) ) ;
#39965=DIRECTION ( 'NONE',  ( 0.000000000000000000, 0.000000000000000000, -1.000000000000000000 ) ) ;
#39966=CARTESIAN_POINT ( 'NONE',  ( -3.988375677951307541, -80.19515755555565306, -9.982611414254499493 ) ) ;
#39968=CARTESIAN_POINT ( 'NONE',  ( 7.808727470805389537, -79.03618450172675125, -8.052663177511117709 ) ) ;
#39971=CYLINDRICAL_SURFACE ( 'NONE', #55789, 12.00000000000000000 ) ;
#39972=CARTESIAN_POINT ( 'NONE',  ( 5.948804865077000237, -80.22133913145148654, 9.426875752653000262 ) ) ;
#39982=CYLINDRICAL_SURFACE ( 'NONE', #48438, 10.25000000000000000 ) ;
#39983=CARTESIAN_POINT ( 'NONE',  ( -8.243938165231000426, -79.69897570143299959, -7.330703780023000604 ) ) ;
#39984=CARTESIAN_POINT ( 'NONE',  ( -9.596002108778161954, -76.35208333329295272, -7.374560639698982456 ) ) ;
#39990=ORIENTED_EDGE ( 'NONE', *, *, #32337, .T. ) ;
#39992=FACE_OUTER_BOUND ( 'NONE', #10894, .T. ) ;
#40000=CARTESIAN_POINT ( 'NONE',  ( 9.757498334186999855, -76.81312216313399688, 4.823034098846000539 ) ) ;
#40006=CARTESIAN_POINT ( 'NONE',  ( 11.22546153480763564, -77.52033577748665039, -4.386301564758395166 ) ) ;
#40027=CARTESIAN_POINT ( 'NONE',  ( -9.596002108778160178, -78.95208333333330586, -7.374560639698984232 ) ) ;
#40032=EDGE_LOOP ( 'NONE', ( #18436, #22626, #33621, #20324, #22691, #8916, #15236 ) ) ;
#40033=CARTESIAN_POINT ( 'NONE',  ( -2.363548001580171309, -77.20752253318963199, -10.48685899165801416 ) ) ;
#40042=CARTESIAN_POINT ( 'NONE',  ( 4.484759669696999573, -77.53578839696798752, 11.18403784080000030 ) ) ;
#40052=CIRCLE ( 'NONE', #53255, 10.74999999999999822 ) ;
#40060=CARTESIAN_POINT ( 'NONE',  ( -11.48784787867999846, -78.17288519146396197, -3.397854551190000461 ) ) ;
#40079=CARTESIAN_POINT ( 'NONE',  ( 6.261651594248000663, -77.70020226594600388, -8.942431733175999042 ) ) ;
#40080=CARTESIAN_POINT ( 'NONE',  ( 2.284509925729999669, -77.73351832560599917, 12.06552085823000020 ) ) ;
#40087=CARTESIAN_POINT ( 'NONE',  ( 7.584438660666999787, -79.44356212903799985, 9.203919974279001437 ) ) ;
#40089=CARTESIAN_POINT ( 'NONE',  ( -9.167119855300001063, -80.12061390621509815, -6.180331023587999795 ) ) ;
#40094=CARTESIAN_POINT ( 'NONE',  ( 11.19180402071999936, -77.58921497497100006, 0.7494220128532999015 ) ) ;
#40109=VERTEX_POINT ( 'NONE', #50505 ) ;
#40110=LINE ( 'NONE', #22400, #18148 ) ;
#40120=CARTESIAN_POINT ( 'NONE',  ( 3.079339082788000059, -77.26865414418398359, -11.84061610281999855 ) ) ;
#40121=CARTESIAN_POINT ( 'NONE',  ( -10.75000000000000000, -78.60000000000000853, 0.000000000000000000 ) ) ;
#40130=CARTESIAN_POINT ( 'NONE',  ( 11.08595418830999968, -76.98783056546687931, -1.708721840212999776 ) ) ;
#40133=CARTESIAN_POINT ( 'NONE',  ( -4.152600241220000044, -79.49650423252299447, -10.41988588363999924 ) ) ;
#40149=CARTESIAN_POINT ( 'NONE',  ( -1.407171709420418138, -79.61458333333331439, -10.75000000000000000 ) ) ;
#40158=FACE_OUTER_BOUND ( 'NONE', #30946, .T. ) ;
#40159=CARTESIAN_POINT ( 'NONE',  ( 2.220279159302000149, -77.93669951884498914, 11.72628939184999908 ) ) ;
#40162=CARTESIAN_POINT ( 'NONE',  ( 11.68767212001979594, -78.52916666666665435, -3.140974612311341563 ) ) ;
#40163=CARTESIAN_POINT ( 'NONE',  ( -10.17265785211000129, -78.92724904577400480, 4.268344714933999917 ) ) ;
#40168=CARTESIAN_POINT ( 'NONE',  ( -6.659468121095000193, -79.24723885956400693, 10.30708084445999972 ) ) ;
#40175=CARTESIAN_POINT ( 'NONE',  ( -7.771634306715999863, -77.01216573198799153, -9.645635764621999897 ) ) ;
#40179=CARTESIAN_POINT ( 'NONE',  ( 3.646964122112999807, -80.12495082227849252, 10.50067842184000000 ) ) ;
#40183=APPLICATION_CONTEXT ( 'automotive_design' ) ;
#40185=CARTESIAN_POINT ( 'NONE',  ( 8.035240866938423210, -76.30833333333333712, 7.229432123683737110 ) ) ;
#40187=CARTESIAN_POINT ( 'NONE',  ( 9.687205842286999768, -78.02392362630298805, -7.546775612817000045 ) ) ;
#40190=CIRCLE ( 'NONE', #2501, 0.2000000000000005107 ) ;
#40191=CARTESIAN_POINT ( 'NONE',  ( -9.393203674808288994, -79.45833333333331439, 5.413904038987134015 ) ) ;
#40193=DIRECTION ( 'NONE',  ( 1.000000000000000000, 0.000000000000000000, 0.000000000000000000 ) ) ;
#40209=CARTESIAN_POINT ( 'NONE',  ( 0.9578316561260999951, -78.83012074166400396, -11.17589679220000143 ) ) ;
#40212=ORIENTED_EDGE ( 'NONE', *, *, #24747, .T. ) ;
#40225=ORIENTED_EDGE ( 'NONE', *, *, #8627, .T. ) ;
#40226=CARTESIAN_POINT ( 'NONE',  ( -5.117891248972000540, -79.85094018418639905, 10.91715234938999934 ) ) ;
#40227=CARTESIAN_POINT ( 'NONE',  ( 1.549833839051000028, -76.27701249839499553, -11.26909137997999899 ) ) ;
#40228=CARTESIAN_POINT ( 'NONE',  ( -6.833799251793511331, -78.02991085507407831, 8.298221944495866254 ) ) ;
#40229=CARTESIAN_POINT ( 'NONE',  ( 3.249499231398999655, -78.78075334615299141, -11.53069031867000049 ) ) ;
#40231=AXIS2_PLACEMENT_3D ( 'NONE', #52527, #30647, #3232 ) ;
#40237=CARTESIAN_POINT ( 'NONE',  ( 7.461283454533999659, -77.07449396308798839, -8.281536679888001018 ) ) ;
#40239=CARTESIAN_POINT ( 'NONE',  ( 9.818658714980999846, -80.61406345225509540, 5.503422351864000639 ) ) ;
#40240=CIRCLE ( 'NONE', #9145, 12.09999999999999964 ) ;
#40257=CARTESIAN_POINT ( 'NONE',  ( 7.183928826236000376, -78.45794695701400201, -8.388570749380001246 ) ) ;
#40262=DIRECTION ( 'NONE',  ( 0.9805806756909162258, 0.1961161351382035567, -2.366546780594040249E-11 ) ) ;
#40263=CARTESIAN_POINT ( 'NONE',  ( 2.213099632718122045, -80.24184156219480712, -10.51960425961281587 ) ) ;
#40265=CARTESIAN_POINT ( 'NONE',  ( -4.019865671108900251, -79.25407524574178808, 10.47197636312916735 ) ) ;
#40271=DIRECTION ( 'NONE',  ( 1.000000000000000000, 0.000000000000000000, 0.000000000000000000 ) ) ;
#40272=CARTESIAN_POINT ( 'NONE',  ( 5.587778422887999419, -80.05792107344059616, -9.645275144704999803 ) ) ;
#40277=ORIENTED_EDGE ( 'NONE', *, *, #26920, .F. ) ;
#40284=CARTESIAN_POINT ( 'NONE',  ( 9.221778727104000595, -79.34490324240999826, -6.054794091447999627 ) ) ;
#40312=CARTESIAN_POINT ( 'NONE',  ( 0.1701061709968674784, -80.97413665117370840, 10.75656394733976029 ) ) ;
#40313=CARTESIAN_POINT ( 'NONE',  ( -11.26045488449999965, -80.89932530880696504, 0.3336940576009999604 ) ) ;
#40330=CARTESIAN_POINT ( 'NONE',  ( 10.48543666025110355, -79.10833333333332007, -6.043427764450775008 ) ) ;
#40337=CARTESIAN_POINT ( 'NONE',  ( -4.710391155546546749, -77.18893069641463001, -9.663071856776335622 ) ) ;
#40344=CARTESIAN_POINT ( 'NONE',  ( 10.43959491470999978, -79.91030549489470047, -5.976816984917999953 ) ) ;
#40346=CARTESIAN_POINT ( 'NONE',  ( -7.987959636959824472, -80.44130578457811964, 7.262045713485346887 ) ) ;
#40348=CARTESIAN_POINT ( 'NONE',  ( 4.400069678882000623, -77.34588318900199511, -11.21761009915999985 ) ) ;
#40350=ORIENTED_EDGE ( 'NONE', *, *, #6832, .T. ) ;
#40353=CARTESIAN_POINT ( 'NONE',  ( -3.140526010065456397, -76.50359585998626244, -11.68633867987707298 ) ) ;
#40384=CARTESIAN_POINT ( 'NONE',  ( -3.535896000267000350, -77.42783883592798588, 10.32825277893000226 ) ) ;
#40386=CARTESIAN_POINT ( 'NONE',  ( 4.527593368978999777, -77.28578839696798752, 11.29085598690000047 ) ) ;
#40393=CARTESIAN_POINT ( 'NONE',  ( -6.333362933179000009, -79.20385945140999695, -10.10566012912000033 ) ) ;
#40394=CARTESIAN_POINT ( 'NONE',  ( -10.92553478716000015, -80.08564122021149956, -1.692710837394999945 ) ) ;
#40396=DIRECTION ( 'NONE',  ( 0.000000000000000000, 1.000000000000000000, 0.000000000000000000 ) ) ;
#40397=CARTESIAN_POINT ( 'NONE',  ( 10.79417609527999922, -77.56197863196899789, -3.050225076229999832 ) ) ;
#40419=EDGE_CURVE ( 'NONE', #27418, #28917, #22629, .T. ) ;
#40420=( LENGTH_UNIT ( ) NAMED_UNIT ( * ) SI_UNIT ( .MILLI., .METRE. ) );
#40424=CARTESIAN_POINT ( 'NONE',  ( -3.182876184981000112, -77.29539847029199962, -11.93563171605999962 ) ) ;
#40434=CARTESIAN_POINT ( 'NONE',  ( 2.179295889402999897, -78.76112297147399488, 11.00312592022000047 ) ) ;
#40435=B_SPLINE_CURVE_WITH_KNOTS ( 'NONE', 3,
 ( #12632, #43081, #2640, #24775, #53081, #20633, #57219, #29754, #43653, #43939, #38635, #42788, #56653, #56937, #33902, #2352, #16209, #34187 ),
 .UNSPECIFIED., .F., .F.,
 ( 4, 2, 2, 2, 2, 2, 2, 2, 4 ),
 ( 0.000000000000000000, 0.1250000000000000000, 0.2500000000000000000, 0.3750000000000000000, 0.5000000000000000000, 0.6250000000000000000, 0.7500000000000000000, 0.8750000000000000000, 1.000000000000000000 ),
 .UNSPECIFIED. ) ;
#40448=CARTESIAN_POINT ( 'NONE',  ( -11.80208112487999905, -77.22397935580299588, -3.396125071686999952 ) ) ;
#40453=DIRECTION ( 'NONE',  ( 0.000000000000000000, 1.000000000000000000, 0.000000000000000000 ) ) ;
#40454=CARTESIAN_POINT ( 'NONE',  ( -6.606377239730371720, -77.92708333333332860, 8.596418555780411808 ) ) ;
#40459=VECTOR ( 'NONE', #16731, 1000.000000000000000 ) ;
#40461=DIRECTION ( 'NONE',  ( -1.000000000000000000, 0.000000000000000000, 0.000000000000000000 ) ) ;
#40463=CARTESIAN_POINT ( 'NONE',  ( -4.725986768004000638, -78.66919103528699964, -10.95903971673999955 ) ) ;
#40467=CARTESIAN_POINT ( 'NONE',  ( 1.984688374631000007, -80.16613885926460625, -10.73482082212999877 ) ) ;
#40469=ORIENTED_EDGE ( 'NONE', *, *, #11263, .T. ) ;
#40474=CARTESIAN_POINT ( 'NONE',  ( 12.14319089506000005, -76.64257676113498974, 2.982765578692999853 ) ) ;
#40476=CARTESIAN_POINT ( 'NONE',  ( -10.07979664880000037, -76.97175206120299151, 3.736335038366999761 ) ) ;
#40477=ORIENTED_EDGE ( 'NONE', *, *, #8560, .T. ) ;
#40479=CARTESIAN_POINT ( 'NONE',  ( 4.624113774747000249, -78.86790344678600206, -10.14259199460999916 ) ) ;
#40485=CARTESIAN_POINT ( 'NONE',  ( 4.392572548563236090, -76.34166666666665435, 9.875985572401184243 ) ) ;
#40487=AXIS2_PLACEMENT_3D ( 'NONE', #3083, #30210, #52955 ) ;
#40500=ORIENTED_EDGE ( 'NONE', *, *, #26750, .F. ) ;
#40502=CARTESIAN_POINT ( 'NONE',  ( -4.570437647871999687, -78.05012939816998596, 10.04055945087000090 ) ) ;
#40507=CARTESIAN_POINT ( 'NONE',  ( 10.05828973332000054, -78.91182977066900150, -4.964767691657000270 ) ) ;
#40508=CARTESIAN_POINT ( 'NONE',  ( 3.699382908057097907, -81.00000000000004263, 10.19579882665893322 ) ) ;
#40510=ORIENTED_EDGE ( 'NONE', *, *, #25781, .T. ) ;
#40526=CARTESIAN_POINT ( 'NONE',  ( 10.43594335123000150, -79.16914397480000787, 6.758781668662000364 ) ) ;
#40527=CARTESIAN_POINT ( 'NONE',  ( 11.00455182153999978, -76.34027708591699479, 2.368156917827000107 ) ) ;
#40528=CARTESIAN_POINT ( 'NONE',  ( -5.986584471844802025, -78.02217473519631596, 8.928664031516637678 ) ) ;
#40529=CARTESIAN_POINT ( 'NONE',  ( 11.81379047889000056, -77.46494681281700423, 1.987564636421000008 ) ) ;
#40534=CARTESIAN_POINT ( 'NONE',  ( 4.048470932312206116, -80.94447786405585532, 9.958435342381811495 ) ) ;
#40537=CARTESIAN_POINT ( 'NONE',  ( -0.8202502003661999996, -77.51027545111699624, -11.11673469052999863 ) ) ;
#40539=CARTESIAN_POINT ( 'NONE',  ( 4.185745002111000090, -80.73548588867527087, 10.32456989385000057 ) ) ;
#40545=CARTESIAN_POINT ( 'NONE',  ( 6.201912463541000342, -78.43838330275499970, -9.171216270948999494 ) ) ;
#40555=CARTESIAN_POINT ( 'NONE',  ( -11.75000000000000000, -76.04999999999999716, -3.652443742841000169E-09 ) ) ;
#40558=CARTESIAN_POINT ( 'NONE',  ( -6.940497389897999803, -77.13734811451699613, 8.722619821570999576 ) ) ;
#40566=CARTESIAN_POINT ( 'NONE',  ( -0.4146376617620515237, -79.47196598975578752, -11.20935700980288452 ) ) ;
#40571=CARTESIAN_POINT ( 'NONE',  ( 11.26184072110999779, -78.57390417293299834, 0.07002095171032998722 ) ) ;
#40600=CARTESIAN_POINT ( 'NONE',  ( 1.505173492811999969, -76.66263051119899785, -10.77983693663999887 ) ) ;
#40603=CARTESIAN_POINT ( 'NONE',  ( -10.58783149161999937, -80.86163444153436330, -3.847989116766000084 ) ) ;
#40610=CARTESIAN_POINT ( 'NONE',  ( 10.78853149093999875, -80.62844613477429334, -3.242959171380999983 ) ) ;
#40636=CARTESIAN_POINT ( 'NONE',  ( -0.2278969726611020374, -77.22338849210305511, -10.75220085459532449 ) ) ;
#40637=CARTESIAN_POINT ( 'NONE',  ( 10.00716890277181470, -79.09696047196752033, 6.699252482690748245 ) ) ;
#40641=FACE_OUTER_BOUND ( 'NONE', #28803, .T. ) ;
#40644=CARTESIAN_POINT ( 'NONE',  ( 0.000000000000000000, -75.15999999999999659, 0.000000000000000000 ) ) ;
#40646=CARTESIAN_POINT ( 'NONE',  ( 11.95316821454999889, -78.43105580595199910, -1.522347302216999987 ) ) ;
#40660=DIRECTION ( 'NONE',  ( 1.000000000000000000, 0.000000000000000000, 0.000000000000000000 ) ) ;
#40662=CARTESIAN_POINT ( 'NONE',  ( -11.61454496413000115, -77.63029888298812864, 2.935712811417999557 ) ) ;
#40664=CARTESIAN_POINT ( 'NONE',  ( -9.302993349864850714, -76.89708402442933277, -6.267052156691077514 ) ) ;
#40668=CARTESIAN_POINT ( 'NONE',  ( 0.000000000000000000, -76.14999999992500079, 0.000000000000000000 ) ) ;
#40672=CARTESIAN_POINT ( 'NONE',  ( -3.708203932498999933, -76.29999999999999716, 11.41267819554000162 ) ) ;
#40685=CARTESIAN_POINT ( 'NONE',  ( -10.84231296956000001, -78.51729255600099577, 1.272641041331999956 ) ) ;
#40686=CARTESIAN_POINT ( 'NONE',  ( 11.99915429782999965, -78.14045805696299851, 2.610761444098000261 ) ) ;
#40694=CARTESIAN_POINT ( 'NONE',  ( 7.404330972381000464, -80.89001299829502045, 8.210251132378001415 ) ) ;
#40697=LINE ( 'NONE', #16804, #41786 ) ;
#40708=DIRECTION ( 'NONE',  ( 0.000000000000000000, 1.000000000000000000, 0.000000000000000000 ) ) ;
#40716=AXIS2_PLACEMENT_3D ( 'NONE', #40644, #1097, #14058 ) ;
#40722=CARTESIAN_POINT ( 'NONE',  ( -9.764287472051000449, -76.57194759300099918, 7.371956487538999347 ) ) ;
#40723=CARTESIAN_POINT ( 'NONE',  ( -10.45242846958592331, -78.61880728566940491, -2.511674934066081555 ) ) ;
#40725=VERTEX_POINT ( 'NONE', #18406 ) ;
#40730=CARTESIAN_POINT ( 'NONE',  ( -7.374560639698971798, -78.87291666666666856, -9.596002108778163731 ) ) ;
#40741=CARTESIAN_POINT ( 'NONE',  ( -12.27595451887999900, -76.19941089817999114, 0.3505736730271999391 ) ) ;
#40751=CARTESIAN_POINT ( 'NONE',  ( 0.3864029911681999829, -77.12593457586999079, -11.74364478040999948 ) ) ;
#40753=CARTESIAN_POINT ( 'NONE',  ( 9.752895431365999457, -78.77770829698199861, -6.878701514737999290 ) ) ;
#40757=CARTESIAN_POINT ( 'NONE',  ( 10.95738943370000129, -79.19961247579199437, -1.279590238973999927 ) ) ;
#40766=CARTESIAN_POINT ( 'NONE',  ( -11.42547184184000031, -76.90670592927000371, -5.080618559187000116 ) ) ;
#40769=ORIENTED_EDGE ( 'NONE', *, *, #7707, .T. ) ;
#40770=CARTESIAN_POINT ( 'NONE',  ( -10.75919966670999983, -79.75272080125398588, 3.327699969971999572 ) ) ;
#40780=CARTESIAN_POINT ( 'NONE',  ( 6.606377239730313988, -79.32291666666665719, 8.596418555780454440 ) ) ;
#40786=CARTESIAN_POINT ( 'NONE',  ( 12.00000000000000000, -79.54999999999999716, 0.000000000000000000 ) ) ;
#40792=CARTESIAN_POINT ( 'NONE',  ( 10.12138908678999982, -77.42369350912798609, 4.388532480841000449 ) ) ;
#40797=CARTESIAN_POINT ( 'NONE',  ( -9.066796825632000179, -78.81620026593400041, -6.603885667862000375 ) ) ;
#40798=CARTESIAN_POINT ( 'NONE',  ( 0.8000647195480976581, -81.00000000000001421, 10.77406987238426872 ) ) ;
#40811=CARTESIAN_POINT ( 'NONE',  ( 3.113304451009999863, -78.39783470746900207, -10.55022916317000181 ) ) ;
#40818=ORIENTED_EDGE ( 'NONE', *, *, #42083, .F. ) ;
#40819=CARTESIAN_POINT ( 'NONE',  ( 7.619787310138999459, -79.61921597853599053, -9.677026921773000723 ) ) ;
#40820=CARTESIAN_POINT ( 'NONE',  ( 2.940128815575000054, -76.49533191828599854, 10.98859724391999926 ) ) ;
#40821=CARTESIAN_POINT ( 'NONE',  ( -7.602035473967630352, -78.03750729326660007, 7.600743598855997263 ) ) ;
#40822=CARTESIAN_POINT ( 'NONE',  ( 10.99419336675999936, -78.91639992327199593, 4.758540471090999979 ) ) ;
#40824=DIRECTION ( 'NONE',  ( 0.000000000000000000, 1.000000000000000000, 1.322413929418000086E-13 ) ) ;
#40827=CARTESIAN_POINT ( 'NONE',  ( 3.718021618522670213, -80.94702727586427216, 10.08698426341377008 ) ) ;
#40830=CARTESIAN_POINT ( 'NONE',  ( -5.715586620248999772, -77.97329328214799204, -9.570092484259999921 ) ) ;
#40831=CARTESIAN_POINT ( 'NONE',  ( -10.60034922676000058, -80.48104072104460727, -3.033110234585999709 ) ) ;
#40837=CARTESIAN_POINT ( 'NONE',  ( 7.199825537761999961, -77.01785638038899151, 8.601198917431998936 ) ) ;
#40842=CARTESIAN_POINT ( 'NONE',  ( -10.26995137457921992, -78.52463911791149087, -3.283750080291026219 ) ) ;
#40845=CARTESIAN_POINT ( 'NONE',  ( -5.911015991908509903, -76.05000000000002558, 10.22919423390550442 ) ) ;
#40849=CARTESIAN_POINT ( 'NONE',  ( -10.89229298341999908, -77.19182080052098627, 2.369082973246999568 ) ) ;
#40856=B_SPLINE_CURVE_WITH_KNOTS ( 'NONE', 3,
 ( #692, #32221, #9811, #50263, #5375, #2129, #30116, #47878, #52009, #16277, #20985, #34257, #6828, #33685, #7409, #47010, #25123, #56142 ),
 .UNSPECIFIED., .F., .F.,
 ( 4, 2, 2, 2, 2, 2, 2, 2, 4 ),
 ( 0.000000000000000000, 0.1250000000000000000, 0.2500000000000000000, 0.3750000000000000000, 0.5000000000000000000, 0.6250000000000000000, 0.7500000000000000000, 0.8750000000000000000, 1.000000000000000000 ),
 .UNSPECIFIED. ) ;
#40862=CARTESIAN_POINT ( 'NONE',  ( 4.624113774747000249, -79.05017638237299593, -10.14259199460999916 ) ) ;
#40865=ORIENTED_EDGE ( 'NONE', *, *, #1247, .T. ) ;
#40867=ORIENTED_EDGE ( 'NONE', *, *, #16382, .F. ) ;
#40875=CARTESIAN_POINT ( 'NONE',  ( -10.75000000000000000, -78.00000000000000000, 2.252154972635999871E-14 ) ) ;
#40880=EDGE_CURVE ( 'NONE', #45004, #4724, #9875, .T. ) ;
#40888=CONICAL_SURFACE ( 'NONE', #23933, 13.94999999993999928, 0.7853981633972997312 ) ;
#40892=CARTESIAN_POINT ( 'NONE',  ( -6.474781754604000739, -80.27459204492750189, -9.218806710208998112 ) ) ;
#40900=CARTESIAN_POINT ( 'NONE',  ( -2.895922040489999905, -80.22958303545810566, 10.88681414971999928 ) ) ;
#40902=CARTESIAN_POINT ( 'NONE',  ( 12.00000000000000000, -79.04999999999999716, 0.000000000000000000 ) ) ;
#40907=B_SPLINE_CURVE_WITH_KNOTS ( 'NONE', 3,
 ( #22756, #23627, #10064, #41352, #10349, #647, #50805, #360, #36330, #68, #28332, #54355, #46383, #5907, #18046, #45798, #54063, #41061 ),
 .UNSPECIFIED., .F., .F.,
 ( 4, 2, 2, 2, 2, 2, 2, 2, 4 ),
 ( 0.000000000000000000, 0.1250000000000000278, 0.2500000000000000555, 0.3750000000000000000, 0.5000000000000000000, 0.6250000000000000000, 0.7500000000000000000, 0.8750000000000001110, 1.000000000000000000 ),
 .UNSPECIFIED. ) ;
#40912=CARTESIAN_POINT ( 'NONE',  ( -7.627497484503559910, -79.53793217095720536, 7.575070705985291752 ) ) ;
#40913=CARTESIAN_POINT ( 'NONE',  ( 2.853743189566999534E-14, -82.05000000008600125, 0.000000000000000000 ) ) ;
#40922=ADVANCED_FACE ( 'NONE', ( #12442 ), #30435, .F. ) ;
#40929=CARTESIAN_POINT ( 'NONE',  ( -3.442070086358578695, -77.19916421208671409, -10.18408852963041156 ) ) ;
#40930=CARTESIAN_POINT ( 'NONE',  ( -8.359900899578630415E-07, -76.12787248224110215, -11.82848710057588626 ) ) ;
#40937=CARTESIAN_POINT ( 'NONE',  ( -3.928999787110243336, -80.40462189993948527, 10.05523583907100260 ) ) ;
#40939=CARTESIAN_POINT ( 'NONE',  ( -11.55487901120999972, -78.21402128256200115, -3.417680896482000019 ) ) ;
#40953=EDGE_CURVE ( 'NONE', #31986, #25175, #25727, .T. ) ;
#40956=CARTESIAN_POINT ( 'NONE',  ( 10.46934363224000109, -77.44039367502212201, 5.823135730236001173 ) ) ;
#40983=VERTEX_POINT ( 'NONE', #3016 ) ;
#40985=CARTESIAN_POINT ( 'NONE',  ( -9.932608425312000833, -79.57673028327599241, 6.601450038057999237 ) ) ;
#40986=CARTESIAN_POINT ( 'NONE',  ( -6.853378677884999881, -80.64520419626960290, -8.675469944580999737 ) ) ;
#40987=DIRECTION ( 'NONE',  ( 0.000000000000000000, -1.000000000000000000, -4.543461426100999533E-13 ) ) ;
#40989=CARTESIAN_POINT ( 'NONE',  ( -10.96060824219999930, -77.31685154495198731, 2.383941600041999731 ) ) ;
#40993=FACE_OUTER_BOUND ( 'NONE', #11399, .T. ) ;
#40995=CARTESIAN_POINT ( 'NONE',  ( 4.508375518195298248, -81.00000000000001421, -10.10122446274072772 ) ) ;
#41002=AXIS2_PLACEMENT_3D ( 'NONE', #28028, #27735, #1488 ) ;
#41008=EDGE_CURVE ( 'NONE', #51194, #41515, #15400, .T. ) ;
#41016=ORIENTED_EDGE ( 'NONE', *, *, #29620, .T. ) ;
#41018=CARTESIAN_POINT ( 'NONE',  ( 2.269106295766999856E-14, -92.33215535459000023, -9.760776772971999193 ) ) ;
#41046=CARTESIAN_POINT ( 'NONE',  ( 9.148490208346998998, -77.80416746146400442, 7.734416031130999514 ) ) ;
#41049=CARTESIAN_POINT ( 'NONE',  ( 11.75393452337000078, -77.31272526409898660, -2.068948229565000130 ) ) ;
#41053=CARTESIAN_POINT ( 'NONE',  ( -2.637902738039999750, -79.92101177224829200, 10.59324478783000067 ) ) ;
#41058=CARTESIAN_POINT ( 'NONE',  ( 1.407171709420391936, -77.36458333333330017, 10.75000000000000178 ) ) ;
#41061=CARTESIAN_POINT ( 'NONE',  ( 12.00000000000000000, -77.64999999999999147, 0.000000000000000000 ) ) ;
#41066=CARTESIAN_POINT ( 'NONE',  ( -9.010285311145000975, -78.75895807477898813, -6.562724981485000164 ) ) ;
#41068=CARTESIAN_POINT ( 'NONE',  ( -1.356476828458505590, -79.66581317784307714, -11.75740360620952352 ) ) ;
#41078=VERTEX_POINT ( 'NONE', #6490 ) ;
#41080=CARTESIAN_POINT ( 'NONE',  ( 9.963291278272981444, -78.81944231393819678, -4.036724254922090083 ) ) ;
#41083=CARTESIAN_POINT ( 'NONE',  ( -9.831705185582000794, -76.21046601319852698, 5.330239850319000716 ) ) ;
#41085=CARTESIAN_POINT ( 'NONE',  ( -10.95663201459999847, -78.13183842717499772, 1.286059498161999937 ) ) ;
#41089=CARTESIAN_POINT ( 'NONE',  ( -11.96294582457251110, -78.04565904830035095, 0.6386850134296362391 ) ) ;
#41090=CARTESIAN_POINT ( 'NONE',  ( 10.49311453041000064, -80.05515156828879242, -3.963918880051000126 ) ) ;
#41091=CARTESIAN_POINT ( 'NONE',  ( 9.536720110793080352, -80.99999999999998579, 5.361087519179783101 ) ) ;
#41100=CARTESIAN_POINT ( 'NONE',  ( 2.269106295766999856E-14, -92.56607767729998670, 0.000000000000000000 ) ) ;
#41109=CARTESIAN_POINT ( 'NONE',  ( -6.630296030920000305, -79.79479933005599435, 10.05508639755000111 ) ) ;
#41110=CARTESIAN_POINT ( 'NONE',  ( 6.004377887672999847, -75.90363824613500299, 9.521041246372998756 ) ) ;
#41111=CARTESIAN_POINT ( 'NONE',  ( -2.099635473158307786, -77.99077376007581108, 10.54287097477208412 ) ) ;
#41112=CARTESIAN_POINT ( 'NONE',  ( 4.899854808515000215, -78.29242566852499863, -10.93194800986000104 ) ) ;
#41118=CARTESIAN_POINT ( 'NONE',  ( -10.11369910513000114, -76.85660321907299419, 4.686934626122000402 ) ) ;
#41120=CARTESIAN_POINT ( 'NONE',  ( -10.13082369059000065, -80.99114675511358996, -4.351272007672999820 ) ) ;
#41121=ORIENTED_EDGE ( 'NONE', *, *, #14932, .T. ) ;
#41124=CARTESIAN_POINT ( 'NONE',  ( 4.013660496580000903, -78.42022574075399177, -10.47417304634999979 ) ) ;
#41129=CARTESIAN_POINT ( 'NONE',  ( 2.244456003428818125, -78.64167492799113290, -10.54596288039670959 ) ) ;
#41137=CARTESIAN_POINT ( 'NONE',  ( -10.03906427447999938, -77.31402055093700199, -5.104033018226999729 ) ) ;
#41142=CARTESIAN_POINT ( 'NONE',  ( -10.75000000000000000, -80.50000000000000000, -1.711887504597999906E-14 ) ) ;
#41147=CARTESIAN_POINT ( 'NONE',  ( 6.233047529871999615, -78.98050366622999263, 9.960502923565000444 ) ) ;
#41148=CARTESIAN_POINT ( 'NONE',  ( 5.888733633253000477, -78.49219514392800079, -9.599841314972998418 ) ) ;
#41162=ORIENTED_EDGE ( 'NONE', *, *, #3583, .F. ) ;
#41168=CIRCLE ( 'NONE', #40231, 11.59999999999999964 ) ;
#41182=CARTESIAN_POINT ( 'NONE',  ( -9.421357847594000745, -80.31228291220008941, -6.176342950743000770 ) ) ;
#41184=DIRECTION ( 'NONE',  ( -1.000000000000000000, 0.000000000000000000, 0.000000000000000000 ) ) ;
#41185=CARTESIAN_POINT ( 'NONE',  ( 10.38043817655364442, -76.18020833308295892, -5.983885801651409153 ) ) ;
#41197=CARTESIAN_POINT ( 'NONE',  ( -8.938323291245980684, -79.55317274765927493, 5.972287786095013651 ) ) ;
#41200=VERTEX_POINT ( 'NONE', #15055 ) ;
#41210=ORIENTED_EDGE ( 'NONE', *, *, #37643, .F. ) ;
#41220=VECTOR ( 'NONE', #35393, 1000.000000000000000 ) ;
#41222=CARTESIAN_POINT ( 'NONE',  ( -7.660291894363999710, -78.62096101391799152, 9.301381605274000819 ) ) ;
#41227=CARTESIAN_POINT ( 'NONE',  ( -6.014612645882658093, -76.48278618361135273, -10.41488065623265946 ) ) ;
#41232=EDGE_CURVE ( 'NONE', #53789, #31838, #51959, .T. ) ;
#41238=CARTESIAN_POINT ( 'NONE',  ( 5.177752511601999785, -76.53501262057798726, 9.912858493839999952 ) ) ;
#41239=PLANE ( 'NONE',  #23000 ) ;
#41242=ADVANCED_FACE ( 'NONE', ( #53382 ), #42053, .F. ) ;
#41254=CARTESIAN_POINT ( 'NONE',  ( 0.000000000000000000, -90.35000000009100063, -9.649999999909001147 ) ) ;
#41275=CARTESIAN_POINT ( 'NONE',  ( 7.666466404017000968, -80.02291679501679766, 7.955254905497999296 ) ) ;
#41294=CARTESIAN_POINT ( 'NONE',  ( -3.162453476786999840, -78.43086335765900685, -11.86569286591000072 ) ) ;
#41305=ORIENTED_EDGE ( 'NONE', *, *, #17291, .T. ) ;
#41311=CARTESIAN_POINT ( 'NONE',  ( -9.596002108778161954, -78.85208333333332575, -7.374560639698982456 ) ) ;
#41338=CARTESIAN_POINT ( 'NONE',  ( 1.714448272638999793, -77.21325110754499121, -11.65560625356000024 ) ) ;
#41343=CARTESIAN_POINT ( 'NONE',  ( -8.150086036219999386, -78.90001270277200263, 7.434906319739000402 ) ) ;
#41352=CARTESIAN_POINT ( 'NONE',  ( -10.48543666025111776, -77.85833333333330586, 6.043427764450754580 ) ) ;
#41357=CARTESIAN_POINT ( 'NONE',  ( -7.255688098778000139, -79.14026687680399164, 8.462245020330000145 ) ) ;
#41359=CARTESIAN_POINT ( 'NONE',  ( 2.813789756862229652, -79.85416666666667140, 10.47020627418440064 ) ) ;
#41375=CARTESIAN_POINT ( 'NONE',  ( 7.561064631405968406, -78.78706913947456769, -7.641704783336303208 ) ) ;
#41382=CARTESIAN_POINT ( 'NONE',  ( 11.70610040787851780, -78.31695220253838841, 2.546999134027124967 ) ) ;
#41383=CARTESIAN_POINT ( 'NONE',  ( -1.472820794058999905, -78.38041877790499257, -10.90095403661999995 ) ) ;
#41386=CARTESIAN_POINT ( 'NONE',  ( 10.75000000000000000, -77.75000000000000000, 0.000000000000000000 ) ) ;
#41390=CARTESIAN_POINT ( 'NONE',  ( 10.10565965566643065, -76.04999999999999716, 4.494725398156579566 ) ) ;
#41392=CARTESIAN_POINT ( 'NONE',  ( -3.140974612311352221, -77.50416666666666288, -11.68767212001979061 ) ) ;
#41404=CARTESIAN_POINT ( 'NONE',  ( -10.63167128756999880, -76.62632357022098972, 2.002204529075000128 ) ) ;
#41405=CARTESIAN_POINT ( 'NONE',  ( 10.53071379481334979, -77.86619273895507831, 2.161785647016301493 ) ) ;
#41406=CARTESIAN_POINT ( 'NONE',  ( -10.86788298907000083, -77.66845141377899608, -5.040355520269000245 ) ) ;
#41411=FACE_OUTER_BOUND ( 'NONE', #6376, .T. ) ;
#41413=CARTESIAN_POINT ( 'NONE',  ( -7.664623337597000763, -77.45580276511299189, -8.093710500358000104 ) ) ;
#41415=CARTESIAN_POINT ( 'NONE',  ( 9.718307120666999310, -80.68179051666800206, 5.447174627686000470 ) ) ;
#41420=CARTESIAN_POINT ( 'NONE',  ( 10.75916580684000046, -77.97112838545299951, 3.171507801093999657 ) ) ;
#41434=CARTESIAN_POINT ( 'NONE',  ( -10.48543666025109111, -79.34166666666665435, -6.043427764450793660 ) ) ;
#41444=CARTESIAN_POINT ( 'NONE',  ( -10.69024338110999928, -78.91399466736399404, -3.158052726529999799 ) ) ;
#41450=ORIENTED_EDGE ( 'NONE', *, *, #33377, .F. ) ;
#41456=CARTESIAN_POINT ( 'NONE',  ( -10.47020627418439354, -78.02083333333335702, -2.813789756862263847 ) ) ;
#41471=CARTESIAN_POINT ( 'NONE',  ( 3.862060628231000159, -80.61325977223638972, 10.58270681924999934 ) ) ;
#41473=CARTESIAN_POINT ( 'NONE',  ( -10.48543666025111420, -76.75833333333331154, 6.043427764450754580 ) ) ;
#41487=CARTESIAN_POINT ( 'NONE',  ( 7.085755085285039279, -79.41772239509739961, 8.085164613341476070 ) ) ;
#41491=DIRECTION ( 'NONE',  ( -1.000000000000000000, 0.000000000000000000, 0.000000000000000000 ) ) ;
#41504=CARTESIAN_POINT ( 'NONE',  ( -8.593369277392113759, -77.15225396531909041, -6.609291488178449470 ) ) ;
#41509=CARTESIAN_POINT ( 'NONE',  ( 7.652056849482000267, -79.45402974060098700, 9.281873293285000770 ) ) ;
#41512=CARTESIAN_POINT ( 'NONE',  ( -1.033815393572557806, -80.38261156915623928, 10.74597751898181741 ) ) ;
#41514=CARTESIAN_POINT ( 'NONE',  ( -10.82689242272999941, -77.65796654052100223, -5.021344731552000340 ) ) ;
#41515=VERTEX_POINT ( 'NONE', #27025 ) ;
#41531=CARTESIAN_POINT ( 'NONE',  ( -9.831705185582000794, -76.22657204401799902, 5.330239850318999828 ) ) ;
#41533=CARTESIAN_POINT ( 'NONE',  ( 2.084841536542000107, -76.18354795607999108, 11.03345659225000119 ) ) ;
#41538=FACE_OUTER_BOUND ( 'NONE', #14280, .T. ) ;
#41547=CARTESIAN_POINT ( 'NONE',  ( -11.68767212001980127, -79.37916666666666288, 3.140974612311317138 ) ) ;
#41552=DIRECTION ( 'NONE',  ( 0.000000000000000000, -1.000000000000000000, 0.000000000000000000 ) ) ;
#41556=CARTESIAN_POINT ( 'NONE',  ( 0.3960817336853000303, -77.00102680916499764, -12.03780325391999995 ) ) ;
#41564=CARTESIAN_POINT ( 'NONE',  ( 2.381660037360000537, -80.91833076151569060, -11.15416238136999993 ) ) ;
#41569=CARTESIAN_POINT ( 'NONE',  ( 10.75916580684000046, -78.17449404528099421, 3.171507801093999657 ) ) ;
#41574=CARTESIAN_POINT ( 'NONE',  ( 9.237675586264554539, -81.00000000000000000, -5.974098161736779211 ) ) ;
#41584=B_SPLINE_CURVE_WITH_KNOTS ( 'NONE', 3,
 ( #46645, #51655, #15328, #42198, #29181, #20338, #51356, #28892, #47228, #14441, #32436, #55186, #1768, #46061, #19761, #23594, #1188, #37758 ),
 .UNSPECIFIED., .F., .F.,
 ( 4, 2, 2, 2, 2, 2, 2, 2, 4 ),
 ( 0.000000000000000000, 0.1250000000000000000, 0.2499999999999999722, 0.3750000000000000000, 0.5000000000000000000, 0.6250000000000000000, 0.7500000000000000000, 0.8750000000000000000, 1.000000000000000000 ),
 .UNSPECIFIED. ) ;
#41585=CARTESIAN_POINT ( 'NONE',  ( -11.77559907170000031, -78.34947541138799920, -3.482965070681999897 ) ) ;
#41595=CARTESIAN_POINT ( 'NONE',  ( 5.825949712413000192, -79.90361206703849462, 9.232191225927998346 ) ) ;
#41599=CIRCLE ( 'NONE', #52931, 9.700000000000001066 ) ;
#41612=CARTESIAN_POINT ( 'NONE',  ( 11.13784153760999907, -76.35071295976199224, 5.174080857020999957 ) ) ;
#41613=CARTESIAN_POINT ( 'NONE',  ( 13.89999999994000035, -80.79999999994112159, 2.316525911784000115E-09 ) ) ;
#41618=B_SPLINE_CURVE_WITH_KNOTS ( 'NONE', 3,
 ( #1661, #6654, #11390, #1959, #42092, #42969, #38815, #2526, #42675, #11102, #43258, #19952, #20528, #2243, #15805, #37940, #34082, #2814, #19651, #15514, #51545, #55667, #7527, #51835, #29938, #38526, #52406, #47415, #20808, #11961, #37653, #16388, #56541, #51255, #56832, #20241, #6945, #42388, #16102, #56255, #34373, #47991, #15216, #10806, #28787, #46833, #6359, #55963, #33509, #29082, #47127, #24667, #48555, #49128, #3952, #8679, #7813, #35526, #53555, #12808, #17241, #52977, #26097, #16679, #48277, #40263, #13094, #58276, #35827, #31091, #30524, #8382, #57405, #26668, #13389, #39105, #44700, #30807, #25814, #4255, #8101, #57980, #43541, #39677, #22252, #17839, #3671, #21671, #52688, #3105, #53856, #16963, #34660, #49429, #31388, #25524, #21100, #35228, #39966, #57113, #17535, #12243, #30234, #43842, #21954, #21384, #57684, #3389, #39397, #34945, #12526, #48840, #44122, #53259, #26380, #44399, #19296, #1023, #46179, #13980, #27257, #36996, #50308, #45296, #54723, #14850, #36709, #9858, #447, #10151, #14266, #5704, #37288, #1303, #32263, #26965, #31976, #27840, #4847, #8980, #45885, #55304, #9564, #5417 ),
 .UNSPECIFIED., .F., .F.,
 ( 4, 2, 2, 2, 2, 2, 2, 1, 1, 1, 1, 1, 2, 2, 2, 2, 1, 2, 2, 2, 2, 1, 1, 1, 2, 2, 2, 2, 2, 1, 1, 1, 1, 1, 2, 2, 2, 2, 2, 1, 1, 1, 1, 2, 2, 2, 2, 1, 1, 1, 2, 2, 2, 1, 1, 1, 1, 2, 2, 2, 2, 1, 1, 1, 1, 1, 2, 2, 2, 2, 2, 1, 1, 1, 1, 1, 2, 2, 2, 2, 2, 1, 1, 1, 1, 1, 2, 2, 2, 2, 2, 4 ),
 ( 0.000000000000000000, 0.06250000000004092560, 0.1250000000000818512, 0.1875000000001227907, 0.2187500000001432188, 0.2343750000001534051, 0.2421875000001585121, 0.2460937500001610101, 0.2480468750001622313, 0.2490234375001628142, 0.2495117187501630918, 0.2497558593751632583, 0.2498779296876633416, 0.2500000000001634248, 0.2656250000001660339, 0.2734375000001672551, 0.2773437500001679212, 0.2792968750001681988, 0.2812500000001684763, 0.2968750000001711964, 0.3046875000001724731, 0.3085937500001730283, 0.3105468750001733613, 0.3115234375001734723, 0.3120117187501735279, 0.3125000000001736389, 0.3437500000001835754, 0.3593750000001884604, 0.3671875000001909584, 0.3710937500001921796, 0.3730468750001927902, 0.3740234375001931788, 0.3745117187501933453, 0.3747558593751934009, 0.3748779296876934009, 0.3750000000001934009, 0.4062500000001655343, 0.4218750000001516010, 0.4296875000001446621, 0.4335937500001411649, 0.4355468750001393885, 0.4365234375001385003, 0.4370117187501380562, 0.4372558593751378342, 0.4375000000001376121, 0.4687500000001073586, 0.4843750000000923150, 0.4921875000000847655, 0.4960937500000809908, 0.4980468750000791034, 0.4990234375000781042, 0.5000000000000771605, 0.5312500000000467404, 0.5468750000000315303, 0.5546875000000239808, 0.5585937500000202061, 0.5605468750000182077, 0.5615234375000173195, 0.5625000000000164313, 0.5937499999999860112, 0.6093749999999708011, 0.6171874999999632516, 0.6210937499999593658, 0.6230468749999575895, 0.6240234374999565903, 0.6245117187499561462, 0.6247558593749559241, 0.6249999999999555911, 0.6562499999999220623, 0.6718749999999052980, 0.6796874999998968603, 0.6835937499998927525, 0.6855468749998905320, 0.6865234374998895328, 0.6870117187498890887, 0.6872558593748887557, 0.6873779296873886446, 0.6874999999998885336, 0.7187499999998622213, 0.7343749999998491207, 0.7421874999998425704, 0.7460937499998392397, 0.7480468749998375744, 0.7490234374998366862, 0.7495117187498362421, 0.7497558593748360201, 0.7498779296873361311, 0.7499999999998361311, 0.8124999999998770983, 0.8749999999999180655, 0.9374999999999589217, 1.000000000000000000 ),
 .UNSPECIFIED. ) ;
#41619=AXIS2_PLACEMENT_3D ( 'NONE', #4853, #31686, #50024 ) ;
#41626=CARTESIAN_POINT ( 'NONE',  ( -11.57073820100000106, -77.55688910291300431, 2.924640136927000089 ) ) ;
#41639=CARTESIAN_POINT ( 'NONE',  ( -12.48473257364000055, -76.86897319096500780, 0.6967103256584999960 ) ) ;
#41645=CARTESIAN_POINT ( 'NONE',  ( -0.2300833467695000134, -78.39998243216399487, -11.11357981391999949 ) ) ;
#41647=CARTESIAN_POINT ( 'NONE',  ( -11.02119874838501801, -79.57957167422193834, -4.309175828380967133 ) ) ;
#41651=CARTESIAN_POINT ( 'NONE',  ( 0.000000000000000000, -87.59999999999999432, 0.000000000000000000 ) ) ;
#41662=CARTESIAN_POINT ( 'NONE',  ( 6.218583900441460699, -78.77425322109141348, -8.769005864712987375 ) ) ;
#41663=ORIENTED_EDGE ( 'NONE', *, *, #58241, .T. ) ;
#41664=CARTESIAN_POINT ( 'NONE',  ( -5.007180289739999068, -76.66194096900252930, 10.00009952528999868 ) ) ;
#41669=CARTESIAN_POINT ( 'NONE',  ( -12.17523484611175100, -76.55441792555106417, -0.7718671096416708233 ) ) ;
#41670=CARTESIAN_POINT ( 'NONE',  ( 10.42518013479882022, -77.25890890101139519, -5.902164117432179502 ) ) ;
#41671=CARTESIAN_POINT ( 'NONE',  ( -7.408849624938999234, -79.33369078296900057, -8.421820339245000397 ) ) ;
#41672=ORIENTED_EDGE ( 'NONE', *, *, #3355, .T. ) ;
#41689=DIRECTION ( 'NONE',  ( 2.044033345360999863E-13, 0.000000000000000000, -1.000000000000000000 ) ) ;
#41692=CARTESIAN_POINT ( 'NONE',  ( 7.374560639698994002, -79.57708333333330586, -9.596002108778151296 ) ) ;
#41693=CARTESIAN_POINT ( 'NONE',  ( 0.1615182143923999947, -76.15048332335200598, 11.61153150973999892 ) ) ;
#41694=CARTESIAN_POINT ( 'NONE',  ( -0.1351391521504822224, -77.97607996944202569, 10.74916312770440818 ) ) ;
#41695=CARTESIAN_POINT ( 'NONE',  ( -0.7928179559538000021, -78.68583547745299711, -11.95355612866999984 ) ) ;
#41703=CARTESIAN_POINT ( 'NONE',  ( -6.550114462690999950, -77.03327565549399480, -8.876808543633000426 ) ) ;
#41704=CARTESIAN_POINT ( 'NONE',  ( -8.987350104473000201, -77.09032746636262345, 8.369597699504998545 ) ) ;
#41705=CARTESIAN_POINT ( 'NONE',  ( 9.617955526353000550, -80.74951758108093713, 5.390926903509000390 ) ) ;
#41709=CARTESIAN_POINT ( 'NONE',  ( 5.387639657779031310, -80.43347167844690659, 9.329096843696712327 ) ) ;
#41710=CARTESIAN_POINT ( 'NONE',  ( -10.58728162385000005, -77.67152861243299355, 3.705074683290000337 ) ) ;
#41719=CARTESIAN_POINT ( 'NONE',  ( -2.318770996637999904, -77.66809300996099807, 11.02076520135999971 ) ) ;
#41722=CARTESIAN_POINT ( 'NONE',  ( -6.043427764450786555, -79.38333333333332575, -10.48543666025110177 ) ) ;
#41732=CARTESIAN_POINT ( 'NONE',  ( -4.084105282113999813, -79.55368493481499570, -10.24801534084000032 ) ) ;
#41735=ORIENTED_EDGE ( 'NONE', *, *, #8883, .T. ) ;
#41751=ORIENTED_EDGE ( 'NONE', *, *, #21169, .F. ) ;
#41753=CARTESIAN_POINT ( 'NONE',  ( 6.586108526242999694, -80.07391735373440156, 8.810401493720998900 ) ) ;
#41759=CARTESIAN_POINT ( 'NONE',  ( -1.570796326794937636, -76.78541666666666288, 11.99999999999999467 ) ) ;
#41764=CARTESIAN_POINT ( 'NONE',  ( 3.228614917279000185, -80.91423663227269003, -10.79283437469000084 ) ) ;
#41767=CARTESIAN_POINT ( 'NONE',  ( 10.48543666025108045, -77.19166666666664867, 6.043427764450817641 ) ) ;
#41772=ADVANCED_FACE ( 'NONE', ( #14661 ), #32404, .T. ) ;
#41774=CARTESIAN_POINT ( 'NONE',  ( -9.599999999916001059, -87.30000000008399752, 6.531558194539000517E-10 ) ) ;
#41783=CARTESIAN_POINT ( 'NONE',  ( 7.588639323636114931, -79.41262821244031045, 7.614128156161688032 ) ) ;
#41786=VECTOR ( 'NONE', #52813, 1000.000000000000114 ) ;
#41793=DIRECTION ( 'NONE',  ( -0.7071067811865969777, -0.7071067811864980568, 8.468117720049969248E-09 ) ) ;
#41798=CARTESIAN_POINT ( 'NONE',  ( -10.75000000000000000, -80.59999999999999432, 0.000000000000000000 ) ) ;
#41800=EDGE_LOOP ( 'NONE', ( #50222, #20392, #53563, #23039 ) ) ;
#41801=CARTESIAN_POINT ( 'NONE',  ( -2.112861425255000203, -79.24484432466799433, -11.84242215301999934 ) ) ;
#41820=CARTESIAN_POINT ( 'NONE',  ( -10.98928341260028674, -79.80000000000001137, -4.685202055221748374 ) ) ;
#41825=CARTESIAN_POINT ( 'NONE',  ( 10.12567350656000009, -76.05099845009399928, 4.748118780173999909 ) ) ;
#41850=CARTESIAN_POINT ( 'NONE',  ( 12.09396573961999799, -77.10954407085999662, -2.128801122353999986 ) ) ;
#41858=CARTESIAN_POINT ( 'NONE',  ( 8.557023385002000992, -79.94353216860270095, 6.619562533252000947 ) ) ;
#41861=CARTESIAN_POINT ( 'NONE',  ( -5.859445663532000914, -77.82042158625800710, 9.564779511708000115 ) ) ;
#41866=CARTESIAN_POINT ( 'NONE',  ( -7.341957592364786400, -76.13333333332644770, 8.159497658145225429 ) ) ;
#41869=DIRECTION ( 'NONE',  ( 0.7071067811865975328, 0.7071067811864976127, -1.669585032811993884E-09 ) ) ;
#41871=ORIENTED_EDGE ( 'NONE', *, *, #2708, .T. ) ;
#41875=CARTESIAN_POINT ( 'NONE',  ( -11.92228046151999976, -78.74294670917899452, 2.416973144693999931 ) ) ;
#41889=CARTESIAN_POINT ( 'NONE',  ( 10.75000000000000000, -80.84999999999999432, -1.053639850055999980E-14 ) ) ;
#41894=CARTESIAN_POINT ( 'NONE',  ( -10.07979664880000037, -76.57175206120300004, 3.736335038366999761 ) ) ;
#41908=CARTESIAN_POINT ( 'NONE',  ( 9.406806676749999596, -76.76054034281098382, -7.895227358184000899 ) ) ;
#41912=CARTESIAN_POINT ( 'NONE',  ( -0.4146318973826840226, -79.37205812977910568, -11.20920117498000046 ) ) ;
#41921=CARTESIAN_POINT ( 'NONE',  ( 6.958153983328000614, -78.68285191714500115, -9.837675768602998971 ) ) ;
#41929=CONICAL_SURFACE ( 'NONE', #55110, 11.80312499993000053, 0.7853981633972997312 ) ;
#41938=VERTEX_POINT ( 'NONE', #23461 ) ;
#41940=CARTESIAN_POINT ( 'NONE',  ( 10.74999999999999645, -79.76041666666667140, 1.407171709420451666 ) ) ;
#41945=CARTESIAN_POINT ( 'NONE',  ( 11.21680614116372610, -78.60040301369775761, 0.06974094738193595266 ) ) ;
#41948=ADVANCED_FACE ( 'NONE', ( #58318 ), #1058, .T. ) ;
#41952=CARTESIAN_POINT ( 'NONE',  ( -6.043427764450832740, -77.21666666666666856, 10.48543666025107512 ) ) ;
#41956=CARTESIAN_POINT ( 'NONE',  ( 7.609106138680006737, -78.78758249396523183, -7.593667575104682932 ) ) ;
#41961=CARTESIAN_POINT ( 'NONE',  ( -1.035649530420586162, -76.66761614046610873, -12.15563870979175576 ) ) ;
#41962=CARTESIAN_POINT ( 'NONE',  ( -0.08519494393186054226, -78.42546946423334475, 11.97968001115087056 ) ) ;
#41963=CARTESIAN_POINT ( 'NONE',  ( 8.822637088635000069, -80.13686059729418787, 6.926713255916000733 ) ) ;
#41974=CARTESIAN_POINT ( 'NONE',  ( 10.75000000000000000, -80.75000000000000000, 3.489821576044999869E-14 ) ) ;
#41975=CARTESIAN_POINT ( 'NONE',  ( -3.140974612311352221, -78.50416666666664867, -11.68767212001979061 ) ) ;
#41985=CARTESIAN_POINT ( 'NONE',  ( -9.596002108778160178, -79.45208333333332007, -7.374560639698984232 ) ) ;
#41987=CARTESIAN_POINT ( 'NONE',  ( -2.105778458517339580, -77.99082079685921087, 10.54164563490564177 ) ) ;
#41989=CARTESIAN_POINT ( 'NONE',  ( 2.697636866285999968, -77.77696867547399506, -11.67213861177999945 ) ) ;
#41993=CARTESIAN_POINT ( 'NONE',  ( 10.49291542331330085, -80.86792101652982012, 2.341975711254098425 ) ) ;
#41996=CARTESIAN_POINT ( 'NONE',  ( -5.762797186001000327, -77.87760228854999411, 9.407013499219999630 ) ) ;
#41997=CARTESIAN_POINT ( 'NONE',  ( -3.699256142337000064, -77.04934472805763335, 11.71059914860999918 ) ) ;
#41999=ORIENTED_EDGE ( 'NONE', *, *, #11708, .F. ) ;
#42002=CARTESIAN_POINT ( 'NONE',  ( 8.547245099307286154, -80.40224407770602966, 6.556889745432177286 ) ) ;
#42003=CARTESIAN_POINT ( 'NONE',  ( 9.668944085725000193, -77.05840859066300652, 5.685915129398999568 ) ) ;
#42018=CARTESIAN_POINT ( 'NONE',  ( -10.48543666025111420, -77.75833333333331154, 6.043427764450754580 ) ) ;
#42028=CARTESIAN_POINT ( 'NONE',  ( 5.887377288745000214, -80.28906619586439319, 9.329533489291000237 ) ) ;
#42044=DIRECTION ( 'NONE',  ( 1.000000000000000000, 0.000000000000000000, 0.000000000000000000 ) ) ;
#42047=CARTESIAN_POINT ( 'NONE',  ( 10.99999999987063326, -76.04999999999999716, -1.151917307345635244 ) ) ;
#42052=CARTESIAN_POINT ( 'NONE',  ( 3.370554742410902804, -77.44759005475501112, -11.56126178251549064 ) ) ;
#42053=B_SPLINE_SURFACE_WITH_KNOTS ( 'NONE', 3, 3, ( 
 ( #26224, #58104, #36258, #30926, #40694, #13816, #54280, #22078, #21793, #22977, #12929, #40986, #36550, #49857, #13223, #578, #3792, #45426, #54571, #44239, #18557, #9106, #27392, #22682, #14111, #39798, #40089, #40394, #32108, #8507, #50149, #4683, #13522, #49562, #27095 ),
 ( #17667, #286, #53982, #31514, #26501, #44525, #58403, #31217, #53684, #26799, #31816, #17966, #4080, #57811, #45132, #17370, #18264, #35357, #35654, #9401, #49255, #8807, #4967, #44828, #4382, #22383, #35957, #14684, #28256, #2018, #20016, #5833, #37999, #55437, #41858 ),
 ( #56025, #5540, #6421, #24136, #46310, #55735, #37713, #10872, #23550, #19132, #32684, #15573, #46602, #14979, #27681, #28843, #15279, #23840, #32977, #33568, #33272, #14396, #51313, #46893, #51023, #9691, #1435, #24435, #5261, #42450, #54849, #45726, #23268, #41275, #55138 ),
 ( #860, #18844, #36837, #32394, #10572, #50438, #6129, #9990, #27968, #41564, #19426, #46019, #1145, #37127, #42154, #28554, #1724, #19716, #50735, #37417, #10275, #2301, #52747, #43603, #39160, #38871, #43313, #34429, #47758, #7869, #20587, #51606, #56314, #57167, #3442 ) ),
 .UNSPECIFIED., .F., .F., .F.,
 ( 4, 4 ),
 ( 4, 1, 1, 1, 1, 1, 1, 1, 1, 1, 1, 1, 1, 1, 1, 1, 1, 1, 1, 1, 1, 1, 1, 1, 1, 1, 1, 1, 1, 1, 1, 1, 4 ),
 ( -0.1772706441294000235, 1.177270644128999955 ),
 ( 0.3451371257638000123, 0.3660028545997999760, 0.3868685834356999642, 0.4077343122716999835, 0.4286000411075999716, 0.4494657699435999909, 0.4703314987795000346, 0.4911972276154999983, 0.5120629564514999066, 0.5329286852874000058, 0.5537944141233999140, 0.5746601429593000132, 0.5955258717953000325, 0.6163916006312000206, 0.6372573294671999289, 0.6581230583032000592, 0.6789887871390999363, 0.6998545159750999556, 0.7207202448110000548, 0.7415859736469999630, 0.7624517024829000622, 0.7833174313188999704, 0.8041831601548999897, 0.8250488889907999779, 0.8459146178267999971, 0.8667803466626999853, 0.8876460754987000046, 0.9085118043345999927, 0.9293775331706000120, 0.9502432620066000313, 0.9711089908424999084, 0.9919747196785000387, 1.012840448513999903 ),
 .UNSPECIFIED. ) ;
#42069=CARTESIAN_POINT ( 'NONE',  ( -9.495603837127998048, -78.36858404876599593, -6.055366803880999349 ) ) ;
#42079=CARTESIAN_POINT ( 'NONE',  ( 7.593872865574214259, -79.41257358862213778, 7.608910733373231317 ) ) ;
#42080=EDGE_CURVE ( 'NONE', #31055, #38125, #51396, .T. ) ;
#42081=CARTESIAN_POINT ( 'NONE',  ( -11.05000000000000071, -82.00000000000000000, 0.000000000000000000 ) ) ;
#42083=EDGE_CURVE ( 'NONE', #28871, #52300, #2761, .T. ) ;
#42092=CARTESIAN_POINT ( 'NONE',  ( 10.66047430956388098, -80.33875064089707507, -1.546821364917390085 ) ) ;
#42097=CARTESIAN_POINT ( 'NONE',  ( 10.52307592342000042, -79.49193466302899935, 5.828552047478999576 ) ) ;
#42102=CARTESIAN_POINT ( 'NONE',  ( 11.16572056546000091, -77.90213037933499152, 4.214520933710000250 ) ) ;
#42104=ORIENTED_EDGE ( 'NONE', *, *, #3583, .T. ) ;
#42110=DIRECTION ( 'NONE',  ( 0.000000000000000000, 1.000000000000000000, 0.000000000000000000 ) ) ;
#42120=CARTESIAN_POINT ( 'NONE',  ( 2.796280611080251166, -79.79999999999998295, -11.45656887133994672 ) ) ;
#42121=CARTESIAN_POINT ( 'NONE',  ( -10.61761725430558378, -80.08783922550021828, 1.680617290028606270 ) ) ;
#42124=CARTESIAN_POINT ( 'NONE',  ( 1.546553306619000256, -76.33435708466599579, -11.07619323537999989 ) ) ;
#42126=CARTESIAN_POINT ( 'NONE',  ( 10.06614130400000029, -76.60994096989499269, 4.975593240213999735 ) ) ;
#42132=ADVANCED_FACE ( 'NONE', ( #34049 ), #6217, .F. ) ;
#42135=CARTESIAN_POINT ( 'NONE',  ( -10.54622262059968918, -78.08456485334055230, 2.082890139455574552 ) ) ;
#42139=CARTESIAN_POINT ( 'NONE',  ( 7.374560639698954922, -79.22291666666669130, 9.596002108778179718 ) ) ;
#42146=CONICAL_SURFACE ( 'NONE', #9141, 10.29999999990999981, 0.7853981633972997312 ) ;
#42154=CARTESIAN_POINT ( 'NONE',  ( -10.43174122427000050, -80.74346733149751287, 4.611552680554001249 ) ) ;
#42159=DIRECTION ( 'NONE',  ( 0.000000000000000000, 0.000000000000000000, -1.000000000000000000 ) ) ;
#42161=VECTOR ( 'NONE', #40262, 1000.000000000000227 ) ;
#42164=CARTESIAN_POINT ( 'NONE',  ( 8.217893303462044940, -76.05520833333133623, 7.394497070576632858 ) ) ;
#42165=VERTEX_POINT ( 'NONE', #35418 ) ;
#42167=CARTESIAN_POINT ( 'NONE',  ( 11.02326530841000007, -80.95680626100980248, 1.187788371667000131 ) ) ;
#42174=ORIENTED_EDGE ( 'NONE', *, *, #8560, .F. ) ;
#42175=CARTESIAN_POINT ( 'NONE',  ( 11.88669912479000068, -78.52591218578899657, 2.586293583890999948 ) ) ;
#42179=ORIENTED_EDGE ( 'NONE', *, *, #42567, .T. ) ;
#42183=ADVANCED_FACE ( 'NONE', ( #39862 ), #12992, .T. ) ;
#42184=ORIENTED_EDGE ( 'NONE', *, *, #25781, .F. ) ;
#42198=CARTESIAN_POINT ( 'NONE',  ( 9.393203674808285442, -77.70833333333332860, -5.413904038987152667 ) ) ;
#42205=CARTESIAN_POINT ( 'NONE',  ( -4.885220488697999741, -76.47366117467699098, 11.26753068192000029 ) ) ;
#42210=CARTESIAN_POINT ( 'NONE',  ( -8.286771986066998608, -78.69114955473354200, 7.559597915363999832 ) ) ;
#42219=CARTESIAN_POINT ( 'NONE',  ( 2.974124060854000273, -78.86371401997000419, 11.51680281503000103 ) ) ;
#42228=CARTESIAN_POINT ( 'NONE',  ( -7.352179367232999141, -79.68555078125399405, 9.680938187455000232 ) ) ;
#42230=CARTESIAN_POINT ( 'NONE',  ( 10.75000000000000000, -77.25000000000000000, 0.000000000000000000 ) ) ;
#42232=CARTESIAN_POINT ( 'NONE',  ( -10.75000000000000000, -79.00000000000000000, 0.000000000000000000 ) ) ;
#42237=CARTESIAN_POINT ( 'NONE',  ( 1.546579669427540882, -76.48592740986445904, -11.07638204203961863 ) ) ;
#42257=CARTESIAN_POINT ( 'NONE',  ( 9.008675998456572742, -78.80421538511130564, -5.865726045448368176 ) ) ;
#42264=CARTESIAN_POINT ( 'NONE',  ( 6.036049492268414696, -77.88288315575839249, 10.34824129380889168 ) ) ;
#42265=CARTESIAN_POINT ( 'NONE',  ( 7.910349975595998728, -79.64660642326199991, 7.952639426948999279 ) ) ;
#42266=ORIENTED_EDGE ( 'NONE', *, *, #52837, .T. ) ;
#42267=DIRECTION ( 'NONE',  ( 0.000000000000000000, 1.000000000000000000, 0.000000000000000000 ) ) ;
#42271=CARTESIAN_POINT ( 'NONE',  ( -9.457632199924459471, -78.39508288952933412, -6.031152209911234685 ) ) ;
#42283=CARTESIAN_POINT ( 'NONE',  ( 4.740509660090000743, -78.71728177378300018, 11.49416549648999819 ) ) ;
#42285=CARTESIAN_POINT ( 'NONE',  ( 10.75000000000000000, -77.85000000000000853, 0.000000000000000000 ) ) ;
#42287=CARTESIAN_POINT ( 'NONE',  ( -0.08519377839585000334, -78.44167163863899361, 11.97951611939999950 ) ) ;
#42294=DIRECTION ( 'NONE',  ( 0.000000000000000000, -1.000000000000000000, 0.000000000000000000 ) ) ;
#42296=CARTESIAN_POINT ( 'NONE',  ( -5.656567264032000608, -78.04102034656098397, -9.471271359694998893 ) ) ;
#42297=CARTESIAN_POINT ( 'NONE',  ( -1.925872869407999843, -76.76246555992319998, -12.12904120624999926 ) ) ;
#42303=CARTESIAN_POINT ( 'NONE',  ( 5.263131812197999970, -77.92997156672200276, -9.905430536777000583 ) ) ;
#42307=CARTESIAN_POINT ( 'NONE',  ( -9.626240109848000159, -76.12883592657999543, -7.417705737357999318 ) ) ;
#42313=CARTESIAN_POINT ( 'NONE',  ( -0.8287201338969000242, -77.39572957994299429, -11.23152649900999833 ) ) ;
#42317=CARTESIAN_POINT ( 'NONE',  ( -12.00000000000000000, -78.29999999999999716, 0.000000000000000000 ) ) ;
#42323=ORIENTED_EDGE ( 'NONE', *, *, #9988, .T. ) ;
#42326=CARTESIAN_POINT ( 'NONE',  ( 5.709935245961999861, -78.72334026635199677, 9.573465417320001336 ) ) ;
#42330=EDGE_LOOP ( 'NONE', ( #21967, #42323 ) ) ;
#42332=EDGE_CURVE ( 'NONE', #51603, #7386, #5075, .T. ) ;
#42340=CARTESIAN_POINT ( 'NONE',  ( 10.48543666025110710, -76.50833333332482766, -6.043427764450776785 ) ) ;
#42342=CARTESIAN_POINT ( 'NONE',  ( 10.63562707217000103, -79.97404714773999501, 3.563914325689000240 ) ) ;
#42352=CARTESIAN_POINT ( 'NONE',  ( -2.653227710365042125, -77.40733822163998923, -11.74665041585867975 ) ) ;
#42358=CARTESIAN_POINT ( 'NONE',  ( 1.570796326794856590, -77.26458333333336270, 12.00000000000000711 ) ) ;
#42366=CARTESIAN_POINT ( 'NONE',  ( -4.665811493887000339, -78.23240233375699404, 10.25008134894000023 ) ) ;
#42369=ORIENTED_EDGE ( 'NONE', *, *, #13845, .F. ) ;
#42376=CARTESIAN_POINT ( 'NONE',  ( -0.1055445576787907014, -79.47591176498374921, 10.74947584515206600 ) ) ;
#42380=B_SPLINE_CURVE_WITH_KNOTS ( 'NONE', 3,
 ( #15122, #5975, #6562, #51162, #1863, #37853, #15424, #33416, #51454, #11007, #28991, #53757, #39586, #17741, #30710, #40162, #35137, #39298 ),
 .UNSPECIFIED., .F., .F.,
 ( 4, 2, 2, 2, 2, 2, 2, 2, 4 ),
 ( 0.000000000000000000, 0.1250000000000000000, 0.2500000000000000000, 0.3750000000000000000, 0.5000000000000000000, 0.6250000000000000000, 0.7500000000000000000, 0.8750000000000000000, 1.000000000000000000 ),
 .UNSPECIFIED. ) ;
#42388=CARTESIAN_POINT ( 'NONE',  ( 6.016754219673178028, -80.27273110789552391, -8.908175812766630841 ) ) ;
#42389=CARTESIAN_POINT ( 'NONE',  ( -7.559222841336621812, -77.16294525579797892, -7.643355431292909508 ) ) ;
#42394=CARTESIAN_POINT ( 'NONE',  ( 4.847151869481000297, -78.97589164704000098, 11.00961342987999991 ) ) ;
#42398=CARTESIAN_POINT ( 'NONE',  ( 10.14226539039000130, -78.41758737238698984, 6.290465419776000822 ) ) ;
#42412=CARTESIAN_POINT ( 'NONE',  ( 6.606377239730347739, -80.67708333333331439, -8.596418555780422466 ) ) ;
#42420=CARTESIAN_POINT ( 'NONE',  ( 5.177752511601999785, -76.73837828040700515, 9.912858493839999952 ) ) ;
#42421=CARTESIAN_POINT ( 'NONE',  ( 1.459540817232405363, -76.46516187205870096, 10.67798020080688381 ) ) ;
#42431=CARTESIAN_POINT ( 'NONE',  ( 1.490799555696999956, -79.37411536532098921, 12.10894905701999846 ) ) ;
#42432=CARTESIAN_POINT ( 'NONE',  ( -8.590066394520892601, -78.04883425186237389, 6.463634606814313344 ) ) ;
#42450=CARTESIAN_POINT ( 'NONE',  ( -8.447960142255000804, -80.15114997703010147, 7.488267305661000961 ) ) ;
#42453=CARTESIAN_POINT ( 'NONE',  ( -9.524774638983998898, -77.35740375522699708, 5.924253427062000199 ) ) ;
#42468=CARTESIAN_POINT ( 'NONE',  ( -6.882647548562999873, -78.33600697782200939, -10.03053803679000033 ) ) ;
#42470=CARTESIAN_POINT ( 'NONE',  ( 4.145634294517788199, -78.65634848184657812, -9.984937452013063819 ) ) ;
#42474=CARTESIAN_POINT ( 'NONE',  ( 2.813607249808706801, -77.74586376683228650, -10.46960172016192558 ) ) ;
#42478=CARTESIAN_POINT ( 'NONE',  ( 8.325251318307000048, -79.76743035202900955, -7.061554902978000037 ) ) ;
#42495=CARTESIAN_POINT ( 'NONE',  ( -8.598496321198998871, -77.12938498755599426, -8.768570137950998600 ) ) ;
#42506=CARTESIAN_POINT ( 'NONE',  ( 1.730980777285999972, -77.14552404313198508, -11.76800180821999930 ) ) ;
#42508=EDGE_CURVE ( 'NONE', #28917, #46546, #23868, .T. ) ;
#42511=CARTESIAN_POINT ( 'NONE',  ( -5.128001663057999870, -78.94050342418300659, 9.637373342098999984 ) ) ;
#42525=VERTEX_POINT ( 'NONE', #12352 ) ;
#42526=CARTESIAN_POINT ( 'NONE',  ( 10.12584611049472905, -76.13478022201745432, 4.748199717408892795 ) ) ;
#42543=CARTESIAN_POINT ( 'NONE',  ( -1.085832016961150392, -78.71718408877019613, -10.71637321867290282 ) ) ;
#42552=CARTESIAN_POINT ( 'NONE',  ( -1.780884232981000181, -80.01399474955769620, -11.07459082487999957 ) ) ;
#42554=CARTESIAN_POINT ( 'NONE',  ( 12.00000000000000000, -79.14999999999999147, 0.000000000000000000 ) ) ;
#42556=ORIENTED_EDGE ( 'NONE', *, *, #50594, .T. ) ;
#42559=CARTESIAN_POINT ( 'NONE',  ( 11.69999999991999928, -75.99999999992400035, 2.424609313239000216E-09 ) ) ;
#42567=EDGE_CURVE ( 'NONE', #30430, #8440, #5567, .T. ) ;
#42574=CARTESIAN_POINT ( 'NONE',  ( -12.00000000000000000, -79.39999999999999147, 0.000000000000000000 ) ) ;
#42578=CARTESIAN_POINT ( 'NONE',  ( 0.3864029911681999829, -77.26151168242199674, -11.74364478040999948 ) ) ;
#42582=CARTESIAN_POINT ( 'NONE',  ( 9.571814930552291045, -80.88775658398785140, 4.892930331445250580 ) ) ;
#42584=CARTESIAN_POINT ( 'NONE',  ( -10.69099419661866612, -76.59160594794379051, 1.136506249403649749 ) ) ;
#42585=CARTESIAN_POINT ( 'NONE',  ( 3.906270390259000358, -78.68071061401199984, -10.19392449069000151 ) ) ;
#42587=CARTESIAN_POINT ( 'NONE',  ( 7.244718558131000741, -80.34293552609639733, 7.973405301998999661 ) ) ;
#42595=CARTESIAN_POINT ( 'NONE',  ( 11.08595418830999968, -77.00393590465999694, -1.708721840212999998 ) ) ;
#42599=CARTESIAN_POINT ( 'NONE',  ( -7.698110069955000689, -77.07989279640000291, -9.554382370588998086 ) ) ;
#42616=EDGE_LOOP ( 'NONE', ( #7367, #23786, #12425, #36573 ) ) ;
#42619=ORIENTED_EDGE ( 'NONE', *, *, #11855, .F. ) ;
#42629=CARTESIAN_POINT ( 'NONE',  ( 7.910349975595998728, -79.51102931670899920, 7.952639426948999279 ) ) ;
#42634=CARTESIAN_POINT ( 'NONE',  ( 0.000000000000000000, -75.15999999999999659, 0.000000000000000000 ) ) ;
#42638=CARTESIAN_POINT ( 'NONE',  ( -9.404538367151719314, -77.35366911081999319, -7.521839627126677641 ) ) ;
#42650=CARTESIAN_POINT ( 'NONE',  ( 12.00000000000000000, -78.14999999999999147, 0.000000000000000000 ) ) ;
#42662=CARTESIAN_POINT ( 'NONE',  ( -0.2079424137668072214, -79.47668210426643043, 10.74817616777493079 ) ) ;
#42675=CARTESIAN_POINT ( 'NONE',  ( 9.169614940969610828, -80.30620290186523391, -5.640497885845999981 ) ) ;
#42681=CARTESIAN_POINT ( 'NONE',  ( -0.9103933733443999587, -79.68507749579998745, -11.99492895764000089 ) ) ;
#42685=CARTESIAN_POINT ( 'NONE',  ( -5.241653689492999924, -77.71222517136899910, -10.72196665943000049 ) ) ;
#42687=EDGE_LOOP ( 'NONE', ( #56754, #26231, #17395, #33743 ) ) ;
#42689=CARTESIAN_POINT ( 'NONE',  ( 1.407171709420391936, -78.86458333333331439, 10.75000000000000178 ) ) ;
#42696=ORIENTED_EDGE ( 'NONE', *, *, #23897, .T. ) ;
#42701=AXIS2_PLACEMENT_3D ( 'NONE', #5240, #50714, #46288 ) ;
#42702=CARTESIAN_POINT ( 'NONE',  ( -2.902572068143752571, -79.79999999999998295, -11.46568512432220643 ) ) ;
#42705=CARTESIAN_POINT ( 'NONE',  ( -5.279550234765999939, -76.48755886051600328, -9.859017853534000508 ) ) ;
#42706=CARTESIAN_POINT ( 'NONE',  ( -2.378576911058957855, -76.49343170455809116, 10.59748283465861363 ) ) ;
#42710=CARTESIAN_POINT ( 'NONE',  ( 9.815664359364999925, -76.03305630414600103, -5.453095817054999905 ) ) ;
#42717=CARTESIAN_POINT ( 'NONE',  ( 12.19481035159000015, -79.75646030464399416, -0.3683939141165000208 ) ) ;
#42719=CARTESIAN_POINT ( 'NONE',  ( -9.939585253895419470, -78.06897173951264790, 4.094651989779796608 ) ) ;
#42740=DIRECTION ( 'NONE',  ( -1.000000000000000000, 0.000000000000000000, -3.332495962870000189E-11 ) ) ;
#42741=CARTESIAN_POINT ( 'NONE',  ( 5.263131812197999970, -78.06554867327399450, -9.905430536777000583 ) ) ;
#42757=CARTESIAN_POINT ( 'NONE',  ( 11.38106369370999893, -78.03758450816098957, 4.295802577524999499 ) ) ;
#42760=VERTEX_POINT ( 'NONE', #37193 ) ;
#42766=VECTOR ( 'NONE', #58407, 1000.000000000000000 ) ;
#42770=CARTESIAN_POINT ( 'NONE',  ( 5.592013246121999792, -78.40561320193899064, 9.375753510130000024 ) ) ;
#42772=CARTESIAN_POINT ( 'NONE',  ( 1.407328957790502599, -80.73545652690489760, -10.68057248400399928 ) ) ;
#42785=CARTESIAN_POINT ( 'NONE',  ( 1.298131932841000147, -76.50046698964798964, 12.21218573294999921 ) ) ;
#42788=CARTESIAN_POINT ( 'NONE',  ( 6.043427764450807871, -77.96666666666668277, -10.48543666025108934 ) ) ;
#42795=CARTESIAN_POINT ( 'NONE',  ( 10.00716890277181292, -78.69696047196750044, 6.699252482690747357 ) ) ;
#42798=CARTESIAN_POINT ( 'NONE',  ( -12.14750708673999924, -77.93689196713800982, 0.6485384821269000177 ) ) ;
#42802=CARTESIAN_POINT ( 'NONE',  ( 5.708176239699000121, -78.69537633716700498, -9.305495801267001710 ) ) ;
#42803=CARTESIAN_POINT ( 'NONE',  ( -10.16542146597221041, -79.57365022831298518, 3.500767233281877555 ) ) ;
#42804=ORIENTED_EDGE ( 'NONE', *, *, #28150, .T. ) ;
#42811=CARTESIAN_POINT ( 'NONE',  ( -9.596002108778160178, -77.95208333333332007, -7.374560639698984232 ) ) ;
#42815=CARTESIAN_POINT ( 'NONE',  ( -0.5111749199061261795, -78.92796920241946168, 11.82469092913801489 ) ) ;
#42819=EDGE_CURVE ( 'NONE', #5899, #55147, #22863, .T. ) ;
#42826=CARTESIAN_POINT ( 'NONE',  ( -8.596685113910227827, -78.54795705239990866, 6.606654461210803575 ) ) ;
#42832=CARTESIAN_POINT ( 'NONE',  ( -10.77438703219000082, -76.28333592657999418, 6.510590034606999588 ) ) ;
#42833=CARTESIAN_POINT ( 'NONE',  ( 0.7522352506039718945, -78.73061799086674739, -10.72516942589862765 ) ) ;
#42841=CARTESIAN_POINT ( 'NONE',  ( 2.787211053772591374, -79.74585132458871328, -10.40613102138284418 ) ) ;
#42843=CARTESIAN_POINT ( 'NONE',  ( 6.879576957522999692, -79.15635224922900193, 8.859431780707000215 ) ) ;
#42851=CARTESIAN_POINT ( 'NONE',  ( -2.185822373836047827, -77.95930140150034049, -11.00199025239787431 ) ) ;
#42853=DIRECTION ( 'NONE',  ( 0.000000000000000000, -1.000000000000000000, 0.000000000000000000 ) ) ;
#42859=CARTESIAN_POINT ( 'NONE',  ( -6.309004353333000026, -79.23106629041299698, -10.24224633278999796 ) ) ;
#42866=CARTESIAN_POINT ( 'NONE',  ( -2.814022724594611002, -79.20431978241809645, -10.47055871344663736 ) ) ;
#42867=CARTESIAN_POINT ( 'NONE',  ( 7.851705946354000432, -77.24798175999399064, -9.048036745432998629 ) ) ;
#42872=CARTESIAN_POINT ( 'NONE',  ( 8.977835961907908668, -80.89677031670710505, 5.915845532768282844 ) ) ;
#42875=CARTESIAN_POINT ( 'NONE',  ( -0.9355429176084000265, -78.34062011958100413, 10.99211052673000033 ) ) ;
#42877=CARTESIAN_POINT ( 'NONE',  ( -6.401221879440000428, -80.95148307551198741, 8.835606657229000405 ) ) ;
#42879=ORIENTED_EDGE ( 'NONE', *, *, #38692, .F. ) ;
#42885=CARTESIAN_POINT ( 'NONE',  ( 6.329984427697000093, -78.09338962473199786, 9.260097609460000712 ) ) ;
#42905=EDGE_CURVE ( 'NONE', #20755, #10164, #44999, .T. ) ;
#42914=CARTESIAN_POINT ( 'NONE',  ( -0.8918451245034728636, -81.00000000000001421, -10.91351453700477947 ) ) ;
#42915=CARTESIAN_POINT ( 'NONE',  ( -8.418448289622000758, -77.62832987473298374, -6.950186643912999784 ) ) ;
#42933=CARTESIAN_POINT ( 'NONE',  ( 10.48543666025108045, -76.69166666666666288, 6.043427764450817641 ) ) ;
#42938=CARTESIAN_POINT ( 'NONE',  ( -3.140974612311405512, -77.29583333333333428, 11.68767212001977640 ) ) ;
#42960=CARTESIAN_POINT ( 'NONE',  ( 0.000000000000000000, -75.15999999999999659, 0.000000000000000000 ) ) ;
#42963=CARTESIAN_POINT ( 'NONE',  ( 1.623230447552999944, -77.84549303256399355, -11.02813327291000078 ) ) ;
#42969=CARTESIAN_POINT ( 'NONE',  ( 10.36861781779881220, -80.32830027787916549, -2.923430239069336078 ) ) ;
#42970=CARTESIAN_POINT ( 'NONE',  ( -7.956214544937700417, -76.13333333331455322, 8.846276171663262744 ) ) ;
#42972=CARTESIAN_POINT ( 'NONE',  ( -10.65106809510000119, -79.02763761715399937, 5.591232889670999739 ) ) ;
#42994=CARTESIAN_POINT ( 'NONE',  ( 0.6398064034500148267, -79.79999999999999716, -11.76818875537070319 ) ) ;
#42996=CARTESIAN_POINT ( 'NONE',  ( -10.35066237538938871, -80.07823043094967375, 2.909028927936140541 ) ) ;
#42999=CARTESIAN_POINT ( 'NONE',  ( -9.939389728518001732, -76.86378799035300347, 5.126617716248000001 ) ) ;
#43002=CARTESIAN_POINT ( 'NONE',  ( 7.439409605643000134, -76.07570142656899748, -8.009466158711999739 ) ) ;
#43008=CARTESIAN_POINT ( 'NONE',  ( 11.65955775483000068, -79.23508084193099421, -3.592192024490000080 ) ) ;
#43009=CARTESIAN_POINT ( 'NONE',  ( -10.57218038258165116, -78.08557172664846746, 1.947236671181371337 ) ) ;
#43027=CARTESIAN_POINT ( 'NONE',  ( 1.618170588614999961, -80.38646948174221052, -11.14857479085000058 ) ) ;
#43034=CARTESIAN_POINT ( 'NONE',  ( 1.757484578084819615, -79.96227339042748383, 10.60516276134810987 ) ) ;
#43038=CARTESIAN_POINT ( 'NONE',  ( 10.75336441781152175, -77.34819408117270712, -0.2553265604148902690 ) ) ;
#43057=CARTESIAN_POINT ( 'NONE',  ( 5.887377288745000214, -79.97133913145148654, 9.329533489291000237 ) ) ;
#43067=CARTESIAN_POINT ( 'NONE',  ( 2.946656154917213222, -80.99641046095393904, -10.60865452211998772 ) ) ;
#43068=CARTESIAN_POINT ( 'NONE',  ( 11.70594025892000012, -78.41704903027755336, 2.546964289010999583 ) ) ;
#43081=CARTESIAN_POINT ( 'NONE',  ( -12.00000000000000178, -77.81041666666665435, -1.570796326794897890 ) ) ;
#43087=CARTESIAN_POINT ( 'NONE',  ( 11.87139580924463189, -78.66341727770496561, 2.023209039049198132 ) ) ;
#43090=CARTESIAN_POINT ( 'NONE',  ( 0.3886576371541999864, -77.13648093799099570, -11.81216847760999933 ) ) ;
#43095=CARTESIAN_POINT ( 'NONE',  ( -9.938393956912895177, -79.56898363239373850, 4.097518548705139096 ) ) ;
#43099=CARTESIAN_POINT ( 'NONE',  ( 1.316424014360000116, -79.32485377751800115, -11.96909690421999883 ) ) ;
#43105=CARTESIAN_POINT ( 'NONE',  ( 10.48543666025110355, -78.10833333333330586, -6.043427764450775008 ) ) ;
#43108=DIRECTION ( 'NONE',  ( -0.7071067811864980568, 0.7071067811865969777, -6.606096994262980545E-09 ) ) ;
#43109=CARTESIAN_POINT ( 'NONE',  ( -9.500996395764293112, -79.10045220966165402, -7.058099219916003086 ) ) ;
#43111=B_SPLINE_CURVE_WITH_KNOTS ( 'NONE', 3,
 ( #18103, #9242, #36098, #27227, #45266, #4814, #46738, #32815, #15704, #1856, #6844, #33113, #50862, #33985, #23973, #52024, #47611, #2427, #24273, #11577, #14818, #10999, #28984, #37548 ),
 .UNSPECIFIED., .F., .F.,
 ( 4, 2, 2, 2, 2, 2, 2, 2, 2, 2, 2, 4 ),
 ( 0.000000000000000000, 0.06249999999999998612, 0.1249999999999999722, 0.2499999999999998890, 0.3749999999999998890, 0.4999999999999998890, 0.6249999999999998890, 0.7499999999999997780, 0.8124999999999997780, 0.8749999999999997780, 0.9374999999999998890, 1.000000000000000000 ),
 .UNSPECIFIED. ) ;
#43112=ORIENTED_EDGE ( 'NONE', *, *, #45014, .F. ) ;
#43117=AXIS2_PLACEMENT_3D ( 'NONE', #4362, #16287, #52299 ) ;
#43123=CARTESIAN_POINT ( 'NONE',  ( 8.260736141417000411, -77.07624636657099870, 9.342201263974001080 ) ) ;
#43124=CARTESIAN_POINT ( 'NONE',  ( -4.744750002824204671, -78.68878635233461694, -9.646253556620013825 ) ) ;
#43134=CARTESIAN_POINT ( 'NONE',  ( 3.463650534536347969, -79.75105914263811258, -10.20053198629427449 ) ) ;
#43137=CARTESIAN_POINT ( 'NONE',  ( 10.54265532893000135, -78.61162538919300857, 3.830212845596999927 ) ) ;
#43139=DIRECTION ( 'NONE',  ( -1.776356839400000238E-14, 1.000000000000000000, 0.000000000000000000 ) ) ;
#43143=CARTESIAN_POINT ( 'NONE',  ( 10.29127903888148587, -77.63246528547833236, 4.462195054874572797 ) ) ;
#43145=DIRECTION ( 'NONE',  ( 0.000000000000000000, -1.000000000000000000, 0.000000000000000000 ) ) ;
#43158=CYLINDRICAL_SURFACE ( 'NONE', #16273, 10.75000000000000000 ) ;
#43159=CARTESIAN_POINT ( 'NONE',  ( -11.74098051674999965, -78.48240034705800383, 2.380218674853999961 ) ) ;
#43160=CARTESIAN_POINT ( 'NONE',  ( 8.899186938124000079, -76.04999999999999716, -6.465637775218000094 ) ) ;
#43167=CARTESIAN_POINT ( 'NONE',  ( -9.786314039287999478, -78.49005621299899360, 4.837708502169000724 ) ) ;
#43169=CARTESIAN_POINT ( 'NONE',  ( 8.124492283498000234, -80.26625923301560306, 7.143800282656999734 ) ) ;
#43176=CARTESIAN_POINT ( 'NONE',  ( 1.633411169670999863, -77.90273522372000059, -11.09730050697999992 ) ) ;
#43180=CARTESIAN_POINT ( 'NONE',  ( -1.031652589152999955, -76.69482700115399609, -12.10872576042000048 ) ) ;
#43195=CARTESIAN_POINT ( 'NONE',  ( -11.75000000000000000, -76.04999999999999716, -3.652443742841000169E-09 ) ) ;
#43202=CARTESIAN_POINT ( 'NONE',  ( -10.12544791843921921, -81.00000000000000000, -3.792049412059997238 ) ) ;
#43203=CARTESIAN_POINT ( 'NONE',  ( -10.64055841416000092, -78.09134770576399376, -2.440058154124999934 ) ) ;
#43206=CARTESIAN_POINT ( 'NONE',  ( 4.138892081263878531, -76.27265625027465035, -9.986824818711193430 ) ) ;
#43224=CARTESIAN_POINT ( 'NONE',  ( 1.634596122093999959, -79.06557642282000131, 11.63574645295999943 ) ) ;
#43229=PRESENTATION_STYLE_ASSIGNMENT (( #34918 ) ) ;
#43241=CARTESIAN_POINT ( 'NONE',  ( 6.606680517516895890, -76.92308210898984555, 8.596804040872029873 ) ) ;
#43252=CARTESIAN_POINT ( 'NONE',  ( -6.868829560331000117, -77.06962105010399000, 8.632549730677999023 ) ) ;
#43258=CARTESIAN_POINT ( 'NONE',  ( 8.471468067312940775, -80.29723165198882384, -6.624523487606162497 ) ) ;
#43259=CARTESIAN_POINT ( 'NONE',  ( 8.779306384098170213, -79.89934045272630669, 6.259721701839533914 ) ) ;
#43262=CARTESIAN_POINT ( 'NONE',  ( 10.52307592342000042, -79.28856900320100465, 5.828552047478999576 ) ) ;
#43264=CARTESIAN_POINT ( 'NONE',  ( 9.492027143945000134, -79.11863103297000066, 6.060972302936999512 ) ) ;
#43282=CARTESIAN_POINT ( 'NONE',  ( -6.933401639485825108, -80.03115928570328208, 8.214959689914797636 ) ) ;
#43286=CARTESIAN_POINT ( 'NONE',  ( -11.08400893143999966, -76.41231303454900115, -1.489506537590000068 ) ) ;
#43288=CARTESIAN_POINT ( 'NONE',  ( -9.545928121132844169, -76.56127930255610181, 5.170097460472787176 ) ) ;
#43295=CARTESIAN_POINT ( 'NONE',  ( -10.71959597024094357, -78.09352535383699490, 0.8823199016135090389 ) ) ;
#43296=AXIS2_PLACEMENT_3D ( 'NONE', #55037, #19322, #45618 ) ;
#43301=CARTESIAN_POINT ( 'NONE',  ( -5.413904038987176648, -80.08333333333331439, -9.393203674808267678 ) ) ;
#43312=CARTESIAN_POINT ( 'NONE',  ( -9.578166812159000898, -80.20588336572043886, 5.930253639819999201 ) ) ;
#43313=CARTESIAN_POINT ( 'NONE',  ( -9.457088349255998949, -80.32379509945388918, -6.375823316407999819 ) ) ;
#43347=CARTESIAN_POINT ( 'NONE',  ( 3.399186938124000079, -81.00000000000000000, -10.46162167925000119 ) ) ;
#43356=CARTESIAN_POINT ( 'NONE',  ( 0.000000000000000000, -76.00000000000000000, 0.000000000000000000 ) ) ;
#43361=CARTESIAN_POINT ( 'NONE',  ( -10.75000000000000000, -77.10000000000000853, 0.000000000000000000 ) ) ;
#43363=CARTESIAN_POINT ( 'NONE',  ( 7.223234266884169585, -78.72379502737751977, 9.635782272402776627 ) ) ;
#43366=CARTESIAN_POINT ( 'NONE',  ( 2.263099670254000273, -77.80124539001899109, 11.95244370277000101 ) ) ;
#43373=CARTESIAN_POINT ( 'NONE',  ( -9.584887312353000510, -79.20614542599899721, 7.476966992689000335 ) ) ;
#43385=CARTESIAN_POINT ( 'NONE',  ( 0.9255272111422516712, -78.91838681312817982, 11.79783862488386426 ) ) ;
#43399=CARTESIAN_POINT ( 'NONE',  ( -2.034297237242999934, -76.21503136273899770, 12.04999153458000016 ) ) ;
#43400=CARTESIAN_POINT ( 'NONE',  ( -4.627611545769539703, -78.68975661043700143, -9.702900749146444070 ) ) ;
#43411=CARTESIAN_POINT ( 'NONE',  ( 0.7035937412390291801, -79.73022787044054382, -10.74960056497591232 ) ) ;
#43412=DIRECTION ( 'NONE',  ( 1.776356839400000238E-14, -1.000000000000000000, -1.361873576872999870E-13 ) ) ;
#43414=CARTESIAN_POINT ( 'NONE',  ( 3.507155896972999898, -79.18358859223100410, 10.65448112794999957 ) ) ;
#43423=CARTESIAN_POINT ( 'NONE',  ( 11.19968485648553091, -78.09548311650934238, -0.6234324976954068731 ) ) ;
#43425=CYLINDRICAL_SURFACE ( 'NONE', #56862, 12.00000000000000000 ) ;
#43441=CARTESIAN_POINT ( 'NONE',  ( -0.7928179559538000021, -78.61804692417699414, -11.95355612866999984 ) ) ;
#43448=CARTESIAN_POINT ( 'NONE',  ( -10.30400671801000101, -77.99980203896599562, 3.605941145585999763 ) ) ;
#43454=CARTESIAN_POINT ( 'NONE',  ( 4.819843862223000208, -79.98410264634560463, -11.11936209286999855 ) ) ;
#43459=CARTESIAN_POINT ( 'NONE',  ( -4.647088938219000376, -78.24288720701400734, 10.20895072913000057 ) ) ;
#43469=CARTESIAN_POINT ( 'NONE',  ( 4.752670204043000446, -79.54881202183199207, 10.08299194199999960 ) ) ;
#43483=CIRCLE ( 'NONE', #18022, 9.599999999999999645 ) ;
#43487=CARTESIAN_POINT ( 'NONE',  ( -10.49277749691416162, -81.00000000000000000, -2.475435402500910431 ) ) ;
#43488=CARTESIAN_POINT ( 'NONE',  ( 8.899710312955001257, -77.27425741570898765, -6.322224476856000308 ) ) ;
#43509=CARTESIAN_POINT ( 'NONE',  ( -10.52074280999000067, -76.55859650580799780, 1.981313975351000289 ) ) ;
#43511=CARTESIAN_POINT ( 'NONE',  ( 6.035966914210000311, -78.03466243671600466, 10.34809972146999968 ) ) ;
#43516=FILL_AREA_STYLE_COLOUR ( '', #31614 ) ;
#43518=CARTESIAN_POINT ( 'NONE',  ( 10.38236180178000012, -78.04174793274400201, -4.363545344708000151 ) ) ;
#43526=AXIS2_PLACEMENT_3D ( 'NONE', #45889, #10156, #14564 ) ;
#43535=CARTESIAN_POINT ( 'NONE',  ( -4.618124570880000057, -78.11785646258199733, 10.14532039989999923 ) ) ;
#43541=CARTESIAN_POINT ( 'NONE',  ( -0.3522963194903876993, -80.22251540029562022, -10.74992595684041596 ) ) ;
#43547=CARTESIAN_POINT ( 'NONE',  ( 7.313768098873999257, -78.82039211992298533, 9.313141831727000053 ) ) ;
#43549=CARTESIAN_POINT ( 'NONE',  ( 4.671862542492999815, -78.98244931796000401, -10.24732477002999964 ) ) ;
#43550=CARTESIAN_POINT ( 'NONE',  ( -5.387453234146290626, -77.51668997339311318, 9.329326193316637372 ) ) ;
#43566=DIRECTION ( 'NONE',  ( -1.000000000000000000, 0.000000000000000000, 0.000000000000000000 ) ) ;
#43567=CARTESIAN_POINT ( 'NONE',  ( 8.395720671197342000, -79.79999999999999716, 8.420963863932922067 ) ) ;
#43569=CARTESIAN_POINT ( 'NONE',  ( -10.22053362743914739, -80.07494894966288257, 3.332092116523411640 ) ) ;
#43572=CARTESIAN_POINT ( 'NONE',  ( 8.332845033087998843, -75.95903132946799019, -7.273191856730000460 ) ) ;
#43577=CARTESIAN_POINT ( 'NONE',  ( 5.092348204433999825, -76.79555898269899217, 9.749351101430999478 ) ) ;
#43584=CARTESIAN_POINT ( 'NONE',  ( -4.723605729682391008, -78.01121116410763534, 9.658205987086651234 ) ) ;
#43591=CARTESIAN_POINT ( 'NONE',  ( 2.445294723173425666, -79.15875305519165295, 11.79638544041784698 ) ) ;
#43595=EDGE_CURVE ( 'NONE', #26455, #56437, #47449, .T. ) ;
#43597=DIRECTION ( 'NONE',  ( 0.000000000000000000, 1.000000000000000000, 0.000000000000000000 ) ) ;
#43602=CARTESIAN_POINT ( 'NONE',  ( 9.755626371838998168, -80.95832551581119674, -5.633583086437001342 ) ) ;
#43603=CARTESIAN_POINT ( 'NONE',  ( 3.812565921075000031, -80.42871315746478444, -10.74951088042000080 ) ) ;
#43610=DIRECTION ( 'NONE',  ( -1.000000000000000000, 0.000000000000000000, 0.000000000000000000 ) ) ;
#43612=EDGE_LOOP ( 'NONE', ( #1269, #51549, #54230, #27859, #50902 ) ) ;
#43620=CARTESIAN_POINT ( 'NONE',  ( 3.268459929338999981, -78.83799553730899845, -11.59797143510999895 ) ) ;
#43626=VECTOR ( 'NONE', #53745, 1000.000000000000000 ) ;
#43631=CARTESIAN_POINT ( 'NONE',  ( -6.606539651197500973, -80.67294684482473599, -8.596716473525578550 ) ) ;
#43641=CARTESIAN_POINT ( 'NONE',  ( 0.6431793725385238636, -80.47942011144077412, -11.19244995239323082 ) ) ;
#43642=ADVANCED_FACE ( 'NONE', ( #4465 ), #40888, .T. ) ;
#43643=CARTESIAN_POINT ( 'NONE',  ( -10.61596739836999959, -78.68834218451513607, -5.551333230058001611 ) ) ;
#43650=CARTESIAN_POINT ( 'NONE',  ( -4.885220488697999741, -76.40587262140100222, 11.26753068192000029 ) ) ;
#43653=CARTESIAN_POINT ( 'NONE',  ( -1.570796326794885012, -77.91458333333332575, -12.00000000000000178 ) ) ;
#43661=CARTESIAN_POINT ( 'NONE',  ( -6.882647548562999873, -78.01827991340999802, -10.03053803679000033 ) ) ;
#43666=CARTESIAN_POINT ( 'NONE',  ( -8.963728694014600151, -79.55351885351645080, 5.934108186058405288 ) ) ;
#43670=CARTESIAN_POINT ( 'NONE',  ( -2.877117145850999869, -79.15287816430300438, 11.81089489835999906 ) ) ;
#43673=CARTESIAN_POINT ( 'NONE',  ( -2.828679940991994712, -76.24010416705776549, -10.52886932951727950 ) ) ;
#43687=AXIS2_PLACEMENT_3D ( 'NONE', #5122, #43597, #23118 ) ;
#43698=VERTEX_POINT ( 'NONE', #35740 ) ;
#43700=CARTESIAN_POINT ( 'NONE',  ( -4.960656284159999707, -76.66641898352099815, 11.44151978677999892 ) ) ;
#43701=CARTESIAN_POINT ( 'NONE',  ( 5.478873870300920323, -78.76767635739062712, -9.249568154307317158 ) ) ;
#43705=CARTESIAN_POINT ( 'NONE',  ( -12.00000000000000000, -79.79999999999999716, 6.639246269807000381E-13 ) ) ;
#43714=EDGE_LOOP ( 'NONE', ( #219, #41121, #16179, #4028, #33692 ) ) ;
#43731=CARTESIAN_POINT ( 'NONE',  ( -8.850953919802000414, -79.70920438397355667, -8.146641040006999290 ) ) ;
#43733=CARTESIAN_POINT ( 'NONE',  ( 10.74999999999999645, -77.76041666666667140, 1.407171709420451666 ) ) ;
#43738=CARTESIAN_POINT ( 'NONE',  ( 5.537129384246000541, -78.83508144756699210, 10.62336504503000079 ) ) ;
#43739=CARTESIAN_POINT ( 'NONE',  ( 11.00000000000000000, -76.04999999999999716, -1.235097113410999977E-09 ) ) ;
#43741=CARTESIAN_POINT ( 'NONE',  ( -8.070845824547967950, -76.33295874851062024, 8.970534776983710046 ) ) ;
#43751=CARTESIAN_POINT ( 'NONE',  ( -10.21995024406999875, -79.77991147651499659, 6.792424309783999803 ) ) ;
#43756=CARTESIAN_POINT ( 'NONE',  ( 11.59326225177000147, -76.21977822758400123, 4.362717408256999718 ) ) ;
#43761=CARTESIAN_POINT ( 'NONE',  ( 10.05750832943000006, -79.49433933582800194, 4.806363154649000435 ) ) ;
#43773=DIRECTION ( 'NONE',  ( 1.000000000000000000, 0.000000000000000000, 0.000000000000000000 ) ) ;
#43775=ORIENTED_EDGE ( 'NONE', *, *, #47982, .F. ) ;
#43782=CARTESIAN_POINT ( 'NONE',  ( -3.419437234775999812, -78.17305673476900552, -10.36738907398999920 ) ) ;
#43786=CARTESIAN_POINT ( 'NONE',  ( 4.653115705712000505, -78.85735708466600613, -10.20620521156999949 ) ) ;
#43794=DIRECTION ( 'NONE',  ( 0.000000000000000000, 0.000000000000000000, -1.000000000000000000 ) ) ;
#43816=CARTESIAN_POINT ( 'NONE',  ( -2.194598275924000141, -77.93280256073698808, -11.04616236372000060 ) ) ;
#43832=EDGE_CURVE ( 'NONE', #16988, #22076, #34740, .T. ) ;
#43836=CARTESIAN_POINT ( 'NONE',  ( 7.384237969039999072, -76.82449396308798839, -8.196021229627000082 ) ) ;
#43842=CARTESIAN_POINT ( 'NONE',  ( -4.109332157379601114, -80.19416283618738817, -9.933321846854338943 ) ) ;
#43844=CARTESIAN_POINT ( 'NONE',  ( 1.099834709382747855, -79.71709307677275547, 11.16297328563665126 ) ) ;
#43845=CARTESIAN_POINT ( 'NONE',  ( -6.309004353333000026, -79.07938358726799777, -10.24224633278999796 ) ) ;
#43848=CARTESIAN_POINT ( 'NONE',  ( -2.721343196572999723, -79.71783057900900360, 10.92832355692000057 ) ) ;
#43850=CARTESIAN_POINT ( 'NONE',  ( 6.606255055572026080, -77.42296540801065419, 8.596106853357831312 ) ) ;
#43866=CARTESIAN_POINT ( 'NONE',  ( -4.017030179565191261, -80.00544080255656354, 9.987515399741488054 ) ) ;
#43869=CARTESIAN_POINT ( 'NONE',  ( 2.076475668830000121, -76.26182138261400212, 10.98918251355999942 ) ) ;
#43873=CARTESIAN_POINT ( 'NONE',  ( -7.647058570136000100, -76.32652084646099411, 8.064869325795999799 ) ) ;
#43880=VECTOR ( 'NONE', #41552, 1000.000000000000000 ) ;
#43906=CARTESIAN_POINT ( 'NONE',  ( -10.75000000000000000, -80.00000000000000000, 0.000000000000000000 ) ) ;
#43920=EDGE_LOOP ( 'NONE', ( #3735, #6162, #34449, #45892 ) ) ;
#43928=CARTESIAN_POINT ( 'NONE',  ( 11.04260898239051514, -80.61365854145890353, 1.935304240822113275 ) ) ;
#43929=CARTESIAN_POINT ( 'NONE',  ( 4.899854808515000215, -78.30853176858254017, -10.93194800986000459 ) ) ;
#43936=CARTESIAN_POINT ( 'NONE',  ( 11.13784153760999907, -76.28292440648600348, 5.174080857020999957 ) ) ;
#43939=CARTESIAN_POINT ( 'NONE',  ( 1.570796326794909881, -77.93541666666664014, -11.99999999999999822 ) ) ;
#43947=CARTESIAN_POINT ( 'NONE',  ( 12.16237383090999913, -77.69272812832399211, 0.2432969017631999853 ) ) ;
#43952=CARTESIAN_POINT ( 'NONE',  ( -7.803105408193176551, -79.53977973565120863, 7.394832696508047754 ) ) ;
#43957=CARTESIAN_POINT ( 'NONE',  ( -4.882675258918448336, -78.80818948587457839, 11.01334000465016061 ) ) ;
#43958=CARTESIAN_POINT ( 'NONE',  ( -1.773463207542000042, -79.73653206836100082, -11.79367842281000023 ) ) ;
#43981=CARTESIAN_POINT ( 'NONE',  ( 11.41682566273999910, -76.61119783301998609, 5.303682846453999566 ) ) ;
#43991=CIRCLE ( 'NONE', #18554, 9.700000000000001066 ) ;
#43992=CARTESIAN_POINT ( 'NONE',  ( 5.151324428776999476, -77.58703011150687701, 9.964033682248000900 ) ) ;
#43995=CARTESIAN_POINT ( 'NONE',  ( -1.639962962630000076, -78.78835931447599705, 11.09633417262999977 ) ) ;
#44012=CARTESIAN_POINT ( 'NONE',  ( -10.65106809510000119, -79.11153176702256928, 5.591232889670999739 ) ) ;
#44018=CARTESIAN_POINT ( 'NONE',  ( 3.925078296951999501, -78.34675376993899931, 11.31856107452000160 ) ) ;
#44021=CARTESIAN_POINT ( 'NONE',  ( 11.16572056546000091, -77.85531157257399570, 4.214520933710000250 ) ) ;
#44031=CARTESIAN_POINT ( 'NONE',  ( 8.620724302459001009, -79.51357516803899728, -8.733127930375998105 ) ) ;
#44032=DIRECTION ( 'NONE',  ( 0.000000000000000000, 1.000000000000000000, 0.000000000000000000 ) ) ;
#44037=CARTESIAN_POINT ( 'NONE',  ( -12.24519951262000106, -76.51390172182600224, -0.7763026236661999535 ) ) ;
#44041=CARTESIAN_POINT ( 'NONE',  ( -10.88242774903000054, -79.15424884139699202, -1.809558141819000099 ) ) ;
#44052=CARTESIAN_POINT ( 'NONE',  ( -5.830174433585000315, -78.24095814969300022, 10.80762903023000021 ) ) ;
#44054=CARTESIAN_POINT ( 'NONE',  ( -6.606377239730371720, -79.42708333333332860, 8.596418555780411808 ) ) ;
#44059=CARTESIAN_POINT ( 'NONE',  ( 10.54844216519820321, -78.83464910448034857, -2.071644353491631119 ) ) ;
#44063=CARTESIAN_POINT ( 'NONE',  ( -4.037131867638475313, -81.00000000000001421, -10.13568147781903406 ) ) ;
#44064=CARTESIAN_POINT ( 'NONE',  ( -6.797161730763000342, -77.00189398569099808, 8.542479639784000156 ) ) ;
#44067=CARTESIAN_POINT ( 'NONE',  ( 10.89876807034000095, -79.42932028770400166, -2.652350870517000025 ) ) ;
#44084=CARTESIAN_POINT ( 'NONE',  ( -5.605966151088000338, -78.98998022871599289, 10.70477826589000081 ) ) ;
#44087=CARTESIAN_POINT ( 'NONE',  ( 2.956870837876000468, -79.05653331767798875, 11.44999256673999888 ) ) ;
#44093=CARTESIAN_POINT ( 'NONE',  ( -11.99999999994999911, -76.29999999994899440, 3.078392110872999642E-09 ) ) ;
#44095=CARTESIAN_POINT ( 'NONE',  ( 3.911191660715999774, -77.17018495668600053, 10.56108632439999973 ) ) ;
#44097=CARTESIAN_POINT ( 'NONE',  ( -5.396048678459999692, -80.23819584820419948, 9.878076380210000451 ) ) ;
#44113=B_SPLINE_SURFACE_WITH_KNOTS ( 'NONE', 3, 3, ( 
 ( #38788, #14894, #24926, #24640, #38210, #51231, #42069, #10783, #28762, #46811, #24354, #42366, #35203, #21356, #26356, #52664, #52381, #53528, #43518, #13068, #8654, #21929, #43816, #31066, #34345, #17508, #25500, #7501, #12501, #57086, #57954, #53235, #49104, #11935, #47965, #48528, #56807, #21647, #3361, #52951, #3079, #35498, #34636, #39373, #39938, #12783, #21073, #26640, #48815, #44375, #44095, #8073, #39654, #30499, #30781, #26069, #39079, #57379, #3927, #44675, #4228, #22226, #3644, #8358, #16364, #57659, #16652 ),
 ( #29914, #12217, #30206, #16939, #48251, #7788, #17215, #25788, #34920, #49405, #27232, #8954, #9833, #35798, #22819, #14535, #996, #18690, #36103, #36392, #27814, #49700, #28105, #40830, #18109, #26938, #45861, #422, #54120, #50572, #32239, #18982, #45271, #132, #5394, #23403, #9247, #32529, #22527, #5111, #40537, #13954, #41413, #36974, #54987, #10127, #36683, #13661, #50282, #4820, #46155, #18400, #17812, #4527, #31656, #53828, #40237, #31950, #54418, #49995, #23110, #5680, #58252, #712, #41118, #13363, #31361 ),
 ( #44971, #9541, #27524, #45566, #54699, #14243, #10714, #32822, #51743, #19272, #6263, #56448, #42875, #2149, #19556, #19856, #11292, #33118, #11582, #24278, #1564, #50867, #29272, #42296, #37554, #33990, #15709, #2433, #28692, #41996, #47320, #6849, #51160, #16003, #5973, #47030, #23977, #55871, #24859, #20435, #38430, #52029, #20150, #55571, #33704, #46743, #29561, #1861, #1279, #46445, #15120, #37263, #23690, #15422, #37851, #33414, #6560, #51452, #11005, #47616, #41703, #38138, #56160, #55277, #14823, #28989, #10413 ),
 ( #24568, #28399, #42585, #52313, #4675, #18255, #31505, #53370, #40685, #43167, #27085, #34278, #16300, #22070, #7430, #9095, #4371, #22673, #2724, #56741, #58095, #7140, #31206, #12920, #4067, #11869, #45124, #43448, #30917, #49550, #44817, #29846, #277, #58392, #53973, #53671, #17657, #49246, #40079, #22373, #35643, #47899, #48953, #13512, #36249, #54269, #13802, #13210, #40384, #8795, #39786, #35946, #31805, #26788, #17954, #25142, #20720, #38719, #25433, #8496, #3009, #21782, #57800, #17360, #35346, #26493, #44516 ) ),
 .UNSPECIFIED., .F., .F., .F.,
 ( 4, 4 ),
 ( 4, 1, 1, 1, 1, 1, 1, 1, 1, 1, 1, 1, 1, 1, 1, 1, 1, 1, 1, 1, 1, 1, 1, 1, 1, 1, 1, 1, 1, 1, 1, 1, 1, 1, 1, 1, 1, 1, 1, 1, 1, 1, 1, 1, 1, 1, 1, 1, 1, 1, 1, 1, 1, 1, 1, 1, 1, 1, 1, 1, 1, 1, 1, 1, 4 ),
 ( -0.1772706441294000235, 1.177270644128999955 ),
 ( -0.02000000000000000042, -0.003749999999999999861, 0.01250000000000000069, 0.02875000000000000125, 0.04499999999999999833, 0.06124999999999999889, 0.07749999999999999944, 0.09375000000000000000, 0.1100000000000000006, 0.1262500000000000011, 0.1424999999999999878, 0.1587500000000000022, 0.1749999999999999889, 0.1912500000000000033, 0.2074999999999999900, 0.2237500000000000044, 0.2399999999999999911, 0.2562499999999999778, 0.2725000000000000200, 0.2887500000000000067, 0.3049999999999999933, 0.3212499999999999800, 0.3375000000000000222, 0.3537500000000000089, 0.3699999999999999956, 0.3862499999999999822, 0.4025000000000000244, 0.4187500000000000111, 0.4349999999999999978, 0.4512499999999999845, 0.4675000000000000266, 0.4837500000000000133, 0.5000000000000000000, 0.5162499999999999867, 0.5324999999999999734, 0.5487499999999999600, 0.5649999999999999467, 0.5812500000000000444, 0.5975000000000000311, 0.6137500000000000178, 0.6300000000000000044, 0.6462499999999999911, 0.6624999999999999778, 0.6787499999999999645, 0.6949999999999999512, 0.7112500000000000488, 0.7275000000000000355, 0.7437500000000000222, 0.7600000000000000089, 0.7762499999999999956, 0.7924999999999999822, 0.8087499999999999689, 0.8249999999999999556, 0.8412500000000000533, 0.8575000000000000400, 0.8737500000000000266, 0.8900000000000000133, 0.9062500000000000000, 0.9224999999999999867, 0.9387499999999999734, 0.9549999999999999600, 0.9712499999999999467, 0.9875000000000000444, 1.003749999999999920, 1.020000000000000018 ),
 .UNSPECIFIED. ) ;
#44116=CARTESIAN_POINT ( 'NONE',  ( -3.224264963920000504, -76.81051199849498801, -10.67046002915000003 ) ) ;
#44122=CARTESIAN_POINT ( 'NONE',  ( -5.916486123000844088, -80.17868767483665238, -8.975394947010663316 ) ) ;
#44123=CARTESIAN_POINT ( 'NONE',  ( 5.413904038987179312, -77.16666666666664298, -9.393203674808262349 ) ) ;
#44125=CARTESIAN_POINT ( 'NONE',  ( -11.60111135005000094, -79.01961632557299708, -3.181408645392000523 ) ) ;
#44127=CARTESIAN_POINT ( 'NONE',  ( -1.788059198778999770, -79.93572132302399780, -11.11920900327000084 ) ) ;
#44128=CARTESIAN_POINT ( 'NONE',  ( 9.599999999999999645, -90.39999999999999147, 0.000000000000000000 ) ) ;
#44129=ORIENTED_EDGE ( 'NONE', *, *, #31581, .T. ) ;
#44137=CARTESIAN_POINT ( 'NONE',  ( -9.543280303650000462, -79.11375811998600227, -5.301053389303000074 ) ) ;
#44148=CARTESIAN_POINT ( 'NONE',  ( 9.567264450310133839, -79.79999999999999716, 6.968530294715381324 ) ) ;
#44150=CARTESIAN_POINT ( 'NONE',  ( -8.446513303087588298, -80.04704965811107797, 6.650504277378666451 ) ) ;
#44157=CARTESIAN_POINT ( 'NONE',  ( 1.800245306220000119, -76.88836798910099901, 10.73450256003999925 ) ) ;
#44179=CARTESIAN_POINT ( 'NONE',  ( -11.26045488450000143, -80.74764171378579647, 0.3336940576009999604 ) ) ;
#44194=ORIENTED_EDGE ( 'NONE', *, *, #33929, .F. ) ;
#44210=CIRCLE ( 'NONE', #43296, 12.00000000000000178 ) ;
#44222=CARTESIAN_POINT ( 'NONE',  ( 3.090997446795999970, -77.14356191088999992, -11.88544462247999967 ) ) ;
#44224=CARTESIAN_POINT ( 'NONE',  ( -10.34999999999999964, -82.00000000000000000, 0.000000000000000000 ) ) ;
#44229=CARTESIAN_POINT ( 'NONE',  ( -11.79389253715000052, -77.42143497408700625, 2.981045019388999684 ) ) ;
#44235=CARTESIAN_POINT ( 'NONE',  ( -7.653399028025074102, -79.53820228785095026, 7.548941424443766479 ) ) ;
#44238=CARTESIAN_POINT ( 'NONE',  ( -10.02838903155999972, -79.64445734768898433, 6.665108128633999485 ) ) ;
#44239=CARTESIAN_POINT ( 'NONE',  ( 9.550506292781999917, -80.36542270824050149, 5.569596721165000375 ) ) ;
#44246=CARTESIAN_POINT ( 'NONE',  ( 6.365665562422999635, -79.13050366622999832, 10.17242851768000023 ) ) ;
#44254=ORIENTED_EDGE ( 'NONE', *, *, #27902, .F. ) ;
#44265=CARTESIAN_POINT ( 'NONE',  ( -3.685303599376999806, -77.02275771435500928, 11.66643009639000006 ) ) ;
#44266=CARTESIAN_POINT ( 'NONE',  ( -10.43384097447730419, -78.61940185271862447, -2.589511503229956713 ) ) ;
#44272=CARTESIAN_POINT ( 'NONE',  ( 8.282307197233999219, -77.94110257053002044, -7.564489280984999731 ) ) ;
#44275=CARTESIAN_POINT ( 'NONE',  ( -0.2721098858049000313, -79.27861348850899503, 11.21356619464000026 ) ) ;
#44283=CARTESIAN_POINT ( 'NONE',  ( -10.64937091039521988, -76.82864424258517033, 2.917955610043998504 ) ) ;
#44288=EDGE_CURVE ( 'NONE', #47573, #31099, #26902, .T. ) ;
#44300=CARTESIAN_POINT ( 'NONE',  ( -8.557169117579000783, -77.56000362265000092, -8.383968101560000719 ) ) ;
#44303=CARTESIAN_POINT ( 'NONE',  ( 10.65351345285000129, -78.28938061935399162, -5.379419444189999844 ) ) ;
#44314=CARTESIAN_POINT ( 'NONE',  ( -8.649885944100999424, -77.88881474799100602, -7.141259254888000285 ) ) ;
#44318=CARTESIAN_POINT ( 'NONE',  ( 11.91558074863000094, -76.77803088996098779, 2.926857068649999949 ) ) ;
#44322=CARTESIAN_POINT ( 'NONE',  ( -3.953505135776000046, -79.04530346938999230, 10.29910343295999908 ) ) ;
#44328=CARTESIAN_POINT ( 'NONE',  ( -6.947761447124999989, -78.40373404223500131, -10.12543283296999874 ) ) ;
#44336=DIRECTION ( 'NONE',  ( 0.000000000000000000, -1.000000000000000000, -1.820765760384999999E-13 ) ) ;
#44342=CARTESIAN_POINT ( 'NONE',  ( -3.157677208335999630, -76.67505786966898995, -10.45009290908999944 ) ) ;
#44345=CARTESIAN_POINT ( 'NONE',  ( -6.206245474241999460, -79.68776324199299665, 9.343480492029000217 ) ) ;
#44348=EDGE_CURVE ( 'NONE', #3688, #10604, #51974, .T. ) ;
#44364=CARTESIAN_POINT ( 'NONE',  ( 7.469016288970999895, -78.89729054645600570, 9.172865387330000786 ) ) ;
#44367=CARTESIAN_POINT ( 'NONE',  ( -11.74098051674999965, -78.68576600688699330, 2.380218674853999961 ) ) ;
#44375=CARTESIAN_POINT ( 'NONE',  ( 0.1398360057836000037, -77.19742129968800270, 11.26119045437999944 ) ) ;
#44376=CARTESIAN_POINT ( 'NONE',  ( 6.043427764450761686, -78.13333333333331154, 10.48543666025110888 ) ) ;
#44377=CARTESIAN_POINT ( 'NONE',  ( -10.34222918238999966, -80.85569262628774823, -4.442072403260000080 ) ) ;
#44390=CARTESIAN_POINT ( 'NONE',  ( 0.000000000000000000, -75.15999999999999659, 0.000000000000000000 ) ) ;
#44393=CARTESIAN_POINT ( 'NONE',  ( 2.866472250631999952, -78.13111084099200809, 10.89115702734000024 ) ) ;
#44399=CARTESIAN_POINT ( 'NONE',  ( -5.965906064879229476, -80.17825941931280909, -8.942563257856061654 ) ) ;
#44406=CARTESIAN_POINT ( 'NONE',  ( 0.000000000000000000, -75.15999999999999659, 0.000000000000000000 ) ) ;
#44407=CARTESIAN_POINT ( 'NONE',  ( 10.42771306556999988, -80.11239375944418839, -3.939212573787000515 ) ) ;
#44410=ORIENTED_EDGE ( 'NONE', *, *, #40953, .F. ) ;
#44418=CARTESIAN_POINT ( 'NONE',  ( 7.698699457163000304, -79.38612155000399184, 7.739857405570000459 ) ) ;
#44420=ADVANCED_FACE ( 'NONE', ( #44858 ), #53407, .T. ) ;
#44436=CARTESIAN_POINT ( 'NONE',  ( -1.616093070969999879, -76.91344993108998551, 10.76376729404999999 ) ) ;
#44445=CARTESIAN_POINT ( 'NONE',  ( -11.03620408507000050, -80.34997377947260588, -2.260839449595000161 ) ) ;
#44469=CARTESIAN_POINT ( 'NONE',  ( 8.166441406547827242, -77.29381170557186920, -6.992710802927438962 ) ) ;
#44480=CARTESIAN_POINT ( 'NONE',  ( -10.32936100969000037, -78.64809032934199706, 6.204842689816000068 ) ) ;
#44483=CARTESIAN_POINT ( 'NONE',  ( 11.38757821100306522, -76.62325149914207145, -3.866458184269738307 ) ) ;
#44493=CARTESIAN_POINT ( 'NONE',  ( -10.67244467921999984, -76.67714362518299254, 2.904229794498999873 ) ) ;
#44497=CARTESIAN_POINT ( 'NONE',  ( -8.885616033064000163, -78.09149724519254221, 8.035041515002001589 ) ) ;
#44511=CARTESIAN_POINT ( 'NONE',  ( -9.983732787439539180, -78.13092931071430769, -4.071056266153238568 ) ) ;
#44516=CARTESIAN_POINT ( 'NONE',  ( -7.639223145873000220, -76.96482100489700429, 7.500260266847000423 ) ) ;
#44517=CARTESIAN_POINT ( 'NONE',  ( -5.830174433585000315, -77.78777695645399604, 10.80762903023000021 ) ) ;
#44523=ORIENTED_EDGE ( 'NONE', *, *, #21169, .T. ) ;
#44525=CARTESIAN_POINT ( 'NONE',  ( 10.30142167872999970, -80.92276737670430009, 4.324873734307999484 ) ) ;
#44536=EDGE_CURVE ( 'NONE', #30361, #23662, #18300, .T. ) ;
#44553=SHAPE_REPRESENTATION_RELATIONSHIP ( 'NONE' , 'NONE' ,  #7879, #11003 ) ;
#44557=CARTESIAN_POINT ( 'NONE',  ( 11.56754288844999934, -76.89980949943999633, 3.984846766858999967 ) ) ;
#44565=CARTESIAN_POINT ( 'NONE',  ( 7.199825537761999961, -77.06953959447203317, 8.601198917431998936 ) ) ;
#44568=CARTESIAN_POINT ( 'NONE',  ( -11.06493808903000087, -79.41479520351799692, -1.839906431680000010 ) ) ;
#44581=DIRECTION ( 'NONE',  ( 0.000000000000000000, -1.000000000000000000, 0.000000000000000000 ) ) ;
#44586=DIRECTION ( 'NONE',  ( 0.7071067811865975328, 0.7071067811864976127, 5.769403951028974600E-09 ) ) ;
#44587=CARTESIAN_POINT ( 'NONE',  ( 8.962106380668664940, -80.05087147346051779, 6.668020604379202965 ) ) ;
#44594=CARTESIAN_POINT ( 'NONE',  ( -3.545645331619000196, -77.39722773010799983, 11.44309676683000099 ) ) ;
#44598=CARTESIAN_POINT ( 'NONE',  ( 11.90740810048999876, -78.83196692782999548, 0.8057021066547999100 ) ) ;
#44611=CARTESIAN_POINT ( 'NONE',  ( 8.282307197233999219, -78.02499646299999370, -7.564489280985000619 ) ) ;
#44614=CARTESIAN_POINT ( 'NONE',  ( 9.264606868682999874, -76.81576362826599791, 8.044539538861000594 ) ) ;
#44618=CARTESIAN_POINT ( 'NONE',  ( 2.392795665116000059, -80.06630253886619641, 10.66634390655999987 ) ) ;
#44628=CARTESIAN_POINT ( 'NONE',  ( -1.394284273676999808, -77.94253568003099986, -12.20048157021999913 ) ) ;
#44629=ADVANCED_FACE ( 'NONE', ( #23580 ), #25094, .F. ) ;
#44633=EDGE_CURVE ( 'NONE', #38125, #40983, #14765, .T. ) ;
#44643=CARTESIAN_POINT ( 'NONE',  ( 10.58169901997000117, -77.91394768316000352, 3.119195446298999919 ) ) ;
#44646=CARTESIAN_POINT ( 'NONE',  ( -10.75729140709000120, -78.72117536965599527, -3.177859684493999914 ) ) ;
#44659=DIRECTION ( 'NONE',  ( -1.000000000000000000, 0.000000000000000000, 0.000000000000000000 ) ) ;
#44663=VERTEX_POINT ( 'NONE', #38011 ) ;
#44664=CARTESIAN_POINT ( 'NONE',  ( -8.484929685468999949, -79.30817849819099763, 9.088234785002999416 ) ) ;
#44665=DIRECTION ( 'NONE',  ( 0.000000000000000000, 1.000000000000000000, 0.000000000000000000 ) ) ;
#44666=CARTESIAN_POINT ( 'NONE',  ( -3.610176697326359374, -78.00228815355546885, 10.14026356443288712 ) ) ;
#44667=CARTESIAN_POINT ( 'NONE',  ( 7.851705946354000432, -77.38355886654599658, -9.048036745432998629 ) ) ;
#44672=CARTESIAN_POINT ( 'NONE',  ( 6.169139874394665490, -80.92666250314678678, 8.803678268947257024 ) ) ;
#44675=CARTESIAN_POINT ( 'NONE',  ( -3.257558841711999609, -76.92505786966898995, -10.78064358917000121 ) ) ;
#44677=CARTESIAN_POINT ( 'NONE',  ( 8.294030550005999203, -80.13080510418970448, 7.292873907683000034 ) ) ;
#44694=CARTESIAN_POINT ( 'NONE',  ( 9.087383623426001478, -77.40971154453498571, -6.455544860934000262 ) ) ;
#44700=CARTESIAN_POINT ( 'NONE',  ( 0.3418130752321197896, -80.22786251027696380, -10.74510901840848121 ) ) ;
#44701=CARTESIAN_POINT ( 'NONE',  ( -10.47020627418439354, -77.02083333333335702, -2.813789756862263847 ) ) ;
#44702=CARTESIAN_POINT ( 'NONE',  ( -8.286887192105083955, -78.79105741471079227, 7.559703011935064332 ) ) ;
#44707=CARTESIAN_POINT ( 'NONE',  ( 2.325232682335999890, -78.46495880092599862, -11.01938817673000059 ) ) ;
#44717=DIRECTION ( 'NONE',  ( -1.000000000000000000, 0.000000000000000000, 0.000000000000000000 ) ) ;
#44718=CARTESIAN_POINT ( 'NONE',  ( 9.953654131039998632, -79.42661227141499580, 4.756732473150000473 ) ) ;
#44738=CARTESIAN_POINT ( 'NONE',  ( -9.910042757802999702, -76.49457567883000308, -4.772096900591000335 ) ) ;
#44741=CARTESIAN_POINT ( 'NONE',  ( 0.000000000000000000, -75.15999999999999659, 0.000000000000000000 ) ) ;
#44745=CARTESIAN_POINT ( 'NONE',  ( 5.365883907697000410, -80.16938766345090528, 9.905345355165000143 ) ) ;
#44749=CARTESIAN_POINT ( 'NONE',  ( -10.75000000000000000, -80.01041666666668561, -1.407171709420427019 ) ) ;
#44764=CARTESIAN_POINT ( 'NONE',  ( 12.00000000000000711, -79.13958333333332007, -1.570796326794872355 ) ) ;
#44771=CARTESIAN_POINT ( 'NONE',  ( -1.301360059616015308, -77.21547344162672744, -10.68678654117428195 ) ) ;
#44775=ORIENTED_EDGE ( 'NONE', *, *, #17197, .F. ) ;
#44777=EDGE_CURVE ( 'NONE', #20674, #57578, #48339, .T. ) ;
#44780=CARTESIAN_POINT ( 'NONE',  ( 10.53043183326000154, -77.48152976611999065, 5.857113494126000575 ) ) ;
#44792=CARTESIAN_POINT ( 'NONE',  ( -11.67929340176440078, -79.80000000000001137, -2.658825183345205456 ) ) ;
#44801=CARTESIAN_POINT ( 'NONE',  ( -10.15788409568143713, -76.92166188270672933, 3.765279467776149858 ) ) ;
#44812=CARTESIAN_POINT ( 'NONE',  ( -10.27011860311526092, -78.12477168548677753, -3.283755321494949087 ) ) ;
#44817=CARTESIAN_POINT ( 'NONE',  ( -2.247674004742000076, -77.91809300996099807, 10.68285203299000052 ) ) ;
#44818=CARTESIAN_POINT ( 'NONE',  ( 3.330893700617000075, -78.52026847289599232, -11.81951464247000061 ) ) ;
#44820=CARTESIAN_POINT ( 'NONE',  ( -2.813789756862251856, -79.10416666666665719, -10.47020627418439709 ) ) ;
#44828=CARTESIAN_POINT ( 'NONE',  ( 3.734633266582000122, -80.29325902863899955, -10.52978014402000007 ) ) ;
#44830=CARTESIAN_POINT ( 'NONE',  ( 0.000000000000000000, -75.15999999999999659, 0.000000000000000000 ) ) ;
#44857=CARTESIAN_POINT ( 'NONE',  ( 7.117776695569999923, -76.44899937808600043, 9.951095779506998085 ) ) ;
#44858=FACE_OUTER_BOUND ( 'NONE', #15755, .T. ) ;
#44865=CARTESIAN_POINT ( 'NONE',  ( -11.21668965365999959, -77.75044816951745474, -0.06311738993059996805 ) ) ;
#44868=CARTESIAN_POINT ( 'NONE',  ( 10.05828973332000054, -79.11519543049799097, -4.964767691657000270 ) ) ;
#44877=VECTOR ( 'NONE', #11937, 1000.000000000000000 ) ;
#44879=EDGE_CURVE ( 'NONE', #14636, #7888, #25186, .T. ) ;
#44882=CARTESIAN_POINT ( 'NONE',  ( 5.459501886381000091, -76.36334185139999420, -11.00074850082999767 ) ) ;
#44893=CARTESIAN_POINT ( 'NONE',  ( 11.97742283006000186, -77.74990883061599334, 0.2395971301470000148 ) ) ;
#44895=CARTESIAN_POINT ( 'NONE',  ( -6.752419751440000617, -78.15373404223500131, -9.840748444448999876 ) ) ;
#44899=CARTESIAN_POINT ( 'NONE',  ( -1.448527388915000103, -78.57317658674999450, -10.72114852740000046 ) ) ;
#44901=EDGE_LOOP ( 'NONE', ( #7241, #33074, #46331, #46684 ) ) ;
#44907=CARTESIAN_POINT ( 'NONE',  ( -11.31898586865000134, -75.98564338555699749, 3.399843791672999771 ) ) ;
#44909=CARTESIAN_POINT ( 'NONE',  ( 3.126548645920367520, -76.85163636138472043, 10.36074945036640393 ) ) ;
#44911=CARTESIAN_POINT ( 'NONE',  ( 10.86346900787000003, -78.97684881879399654, 2.497927478100999910 ) ) ;
#44924=AXIS2_PLACEMENT_3D ( 'NONE', #25729, #39022, #3307 ) ;
#44934=ORIENTED_EDGE ( 'NONE', *, *, #34117, .F. ) ;
#44936=CARTESIAN_POINT ( 'NONE',  ( -7.675142533464999417, -78.07736574117099337, 7.924261572595001191 ) ) ;
#44942=CARTESIAN_POINT ( 'NONE',  ( 2.407803015296000382, -80.12354473002160660, 10.73324203768999929 ) ) ;
#44959=EDGE_LOOP ( 'NONE', ( #18668, #29664, #26682, #13518, #1962, #16553, #18655, #51563, #32024, #57483, #17123 ) ) ;
#44960=CARTESIAN_POINT ( 'NONE',  ( -5.166309513786999652, -79.78321311977300923, 11.02043503902999966 ) ) ;
#44961=CARTESIAN_POINT ( 'NONE',  ( 8.910932162214999508, -76.00998311897500059, 6.639958018061999034 ) ) ;
#44962=CARTESIAN_POINT ( 'NONE',  ( -7.208993631127555979, -78.03351433546752958, 7.975374487723845718 ) ) ;
#44963=CARTESIAN_POINT ( 'NONE',  ( 7.919842512016999514, -77.51920544366500110, 8.988445846368000147 ) ) ;
#44971=CARTESIAN_POINT ( 'NONE',  ( 7.037082147462999870, -78.64021989260099588, -8.217099986793998667 ) ) ;
#44973=CARTESIAN_POINT ( 'NONE',  ( -3.110348726875999947, -80.42612965022969718, -10.81755274276999934 ) ) ;
#44974=VECTOR ( 'NONE', #50782, 1000.000000000000000 ) ;
#44980=CARTESIAN_POINT ( 'NONE',  ( 11.19952915612999966, -77.94389204245099734, -0.6234238306063999424 ) ) ;
#44989=CARTESIAN_POINT ( 'NONE',  ( 9.807952262865001103, -76.91945737050299670, -5.297043796141999827 ) ) ;
#44999=B_SPLINE_CURVE_WITH_KNOTS ( 'NONE', 3,
 ( #20080, #56948, #16508, #33634, #34490, #38357, #15352, #25641, #20647, #15930, #51676, #19786, #55801, #33345, #47248, #51378, #6780, #16221, #42803, #2365, #33917, #7070, #25072, #51956, #43095, #2653, #56665, #31738, #35352, #27319, #39793, #786, #12646, #43666, #48390, #50075, #54778, #14320, #41197, #16798, #26219, #9912, #25928, #21505, #21212, #18766, #43952, #18479, #44235, #40912, #36759, #3503, #23192, #39512, #53376, #52806, #39220, #32314, #57517, #50362, #502, #5188, #3225, #22899, #17077, #12359, #53094, #57233, #3788, #35059, #21789, #34782, #30348, #27606, #7928, #36470, #30639, #48673, #8217, #14035, #9618, #57806, #17366, #12925, #49782, #9328, #45351, #45648, #4901, #54497, #56244, #20230, #15204, #5760, #10494, #50657, #6643, #55952, #37049, #33496, #1945, #46822, #37638, #19939, #5472, #37928, #55066, #2230, #24651, #6347, #24363, #42662, #42376, #23768, #15501, #14615, #6053, #15794, #28774, #38223, #33194, #33782, #51822, #51534, #14904, #27893, #23476, #47113, #45940, #41487, #1074, #10793, #29068, #11090, #19062, #32609, #41783, #42079, #10203, #28182, #46235, #51240, #55361, #1356, #55655, #37345, #19351, #32902, #1649, #50946, #28479 ),
 .UNSPECIFIED., .F., .F.,
 ( 4, 2, 2, 2, 1, 1, 1, 1, 2, 2, 2, 2, 1, 1, 2, 2, 2, 2, 1, 1, 1, 1, 1, 1, 2, 2, 2, 2, 2, 1, 1, 1, 1, 1, 2, 2, 2, 2, 1, 2, 2, 2, 2, 2, 1, 2, 2, 2, 2, 1, 2, 2, 1, 2, 2, 2, 1, 2, 2, 1, 1, 2, 2, 2, 1, 2, 2, 2, 1, 1, 1, 1, 1, 2, 2, 2, 2, 2, 2, 2, 2, 1, 1, 1, 2, 2, 2, 2, 2, 2, 2, 4 ),
 ( 0.000000000000000000, 0.03124999999989156590, 0.04687499999983734539, 0.05468749999981020737, 0.05859374999979660714, 0.06054687499978983478, 0.06152343749978646248, 0.06201171874978477633, 0.06225585937478389509, 0.06249999999978301385, 0.09374999999967163766, 0.1093749999996159461, 0.1171874999995880934, 0.1210937499995741601, 0.1230468749995671379, 0.1249999999995601296, 0.1562499999994484690, 0.1718749999993926247, 0.1796874999993647304, 0.1835937499993507693, 0.1855468749993438027, 0.1865234374993403055, 0.1870117187493385569, 0.1872558593743376687, 0.1873779296868371969, 0.1874999999993367250, 0.2187499999993724187, 0.2343749999993903210, 0.2421874999993992861, 0.2460937499994036992, 0.2480468749994058919, 0.2490234374994070021, 0.2495117187494075572, 0.2497558593744078348, 0.2498779296869079181, 0.2499999999994080291, 0.2812499999994439448, 0.2968749999994619304, 0.2988281249994641509, 0.2998046874994652611, 0.3007812499994663713, 0.3046874999994701461, 0.3124999999994775290, 0.3437499999995065614, 0.3476562499995102251, 0.3496093749995120570, 0.3515624999995138888, 0.3593749999995208833, 0.3749999999995349276, 0.3828124999995419220, 0.3867187499995454192, 0.3876953124995463074, 0.3886718749995471955, 0.3906249999995489164, 0.4062499999995626832, 0.4218749999995764499, 0.4238281249995781708, 0.4248046874995791145, 0.4257812499995800581, 0.4296874999995837774, 0.4374999999995911604, 0.4531249999996059818, 0.4609374999996134203, 0.4628906249996153077, 0.4648437499996171951, 0.4687499999996209143, 0.4843749999996359024, 0.4921874999996433409, 0.4960937499996470601, 0.4980468749996489475, 0.4990234374996498912, 0.4995117187496503908, 0.4997558593746505573, 0.4998779296871507238, 0.4999999999996508349, 0.5624999999996962430, 0.6249999999997415401, 0.6874999999997869482, 0.7187499999998095968, 0.7343749999998209210, 0.7421874999998265832, 0.7460937499998294697, 0.7480468749998309130, 0.7490234374998315792, 0.7495117187498319122, 0.7499999999998321343, 0.7812499999998532285, 0.8124999999998742117, 0.8437499999998951949, 0.8749999999999162892, 0.9374999999999580336, 1.000000000000000000 ),
 .UNSPECIFIED. ) ;
#45002=CARTESIAN_POINT ( 'NONE',  ( -8.329953570067999635, -79.94897570143329801, -7.407190701775999919 ) ) ;
#45004=VERTEX_POINT ( 'NONE', #41798 ) ;
#45014=EDGE_CURVE ( 'NONE', #10331, #36154, #15987, .T. ) ;
#45016=CARTESIAN_POINT ( 'NONE',  ( -1.751509483276000090, -79.75344838743700393, -10.89192126806999994 ) ) ;
#45030=AXIS2_PLACEMENT_3D ( 'NONE', #22045, #4041, #17629 ) ;
#45036=CARTESIAN_POINT ( 'NONE',  ( -7.650190089120999737, -76.96361381506899590, 7.742423574132000219 ) ) ;
#45040=CARTESIAN_POINT ( 'NONE',  ( 3.228614917279000185, -80.98202518554889195, -10.79283437469000084 ) ) ;
#45042=DIRECTION ( 'NONE',  ( 0.000000000000000000, -1.000000000000000000, 0.000000000000000000 ) ) ;
#45044=B_SPLINE_CURVE_WITH_KNOTS ( 'NONE', 3,
 ( #37244, #10392, #6242, #24259, #54681, #28672, #46424, #55550, #977, #14223, #41975, #1546, #27796, #18960, #31931, #36372, #9518, #54398 ),
 .UNSPECIFIED., .F., .F.,
 ( 4, 2, 2, 2, 2, 2, 2, 2, 4 ),
 ( 0.000000000000000000, 0.1250000000000000000, 0.2500000000000000000, 0.3750000000000000000, 0.5000000000000000000, 0.6250000000000000000, 0.7500000000000000000, 0.8750000000000000000, 1.000000000000000000 ),
 .UNSPECIFIED. ) ;
#45047=CARTESIAN_POINT ( 'NONE',  ( -10.34138800174999950, -80.86922762280332222, 4.468208825537999473 ) ) ;
#45073=CARTESIAN_POINT ( 'NONE',  ( 0.4998953799361084971, -77.22882438990886556, -10.73929381184138698 ) ) ;
#45080=CARTESIAN_POINT ( 'NONE',  ( 1.939955037980729990, -80.36060123837306435, 10.61985788779979423 ) ) ;
#45082=CARTESIAN_POINT ( 'NONE',  ( 8.737371597357999065, -78.93304436543799341, 8.129823451939000023 ) ) ;
#45086=CARTESIAN_POINT ( 'NONE',  ( -10.78616240765133227, -76.43596441176799772, -5.318014019118542102 ) ) ;
#45093=CARTESIAN_POINT ( 'NONE',  ( -11.77412505557000699, -79.80000000000001137, -2.187958323471518973 ) ) ;
#45124=CARTESIAN_POINT ( 'NONE',  ( -10.91657421154000041, -78.02703838196799779, -0.06142861151470001280 ) ) ;
#45125=CARTESIAN_POINT ( 'NONE',  ( 11.99621472858000004, -77.20440045069699408, 2.018255885614000267 ) ) ;
#45132=CARTESIAN_POINT ( 'NONE',  ( -10.21850601694999838, -80.60801320267160008, 4.517287938863999486 ) ) ;
#45135=CARTESIAN_POINT ( 'NONE',  ( 11.08595418830999968, -77.07172445793599991, -1.708721840212999998 ) ) ;
#45158=( NAMED_UNIT ( * ) SI_UNIT ( $, .STERADIAN. ) SOLID_ANGLE_UNIT ( ) );
#45161=CARTESIAN_POINT ( 'NONE',  ( -11.75756702865000136, -77.14570592927000803, -3.383315852985000038 ) ) ;
#45162=CARTESIAN_POINT ( 'NONE',  ( -10.28385508244830149, -78.62383711279117904, -3.166186455522963072 ) ) ;
#45168=CARTESIAN_POINT ( 'NONE',  ( -7.712695008784000272, -77.31466668148844690, -8.144473358846001432 ) ) ;
#45182=CARTESIAN_POINT ( 'NONE',  ( 8.174587033571999228, -77.32012175574699597, -8.440297792765999674 ) ) ;
#45188=ORIENTED_EDGE ( 'NONE', *, *, #50760, .T. ) ;
#45195=CARTESIAN_POINT ( 'NONE',  ( 3.910274016995999968, -78.42502719647299614, 11.27587067850999958 ) ) ;
#45199=CARTESIAN_POINT ( 'NONE',  ( -8.157922760392999351, -80.08442983025919659, -7.254216858269000312 ) ) ;
#45206=CARTESIAN_POINT ( 'NONE',  ( -2.626391644478000220, -76.26524937808599702, 12.22522157430999989 ) ) ;
#45209=ORIENTED_EDGE ( 'NONE', *, *, #744, .F. ) ;
#45210=CARTESIAN_POINT ( 'NONE',  ( -6.285096537930999538, -78.78619441778099031, -9.206093747065001054 ) ) ;
#45215=B_SPLINE_CURVE_WITH_KNOTS ( 'NONE', 3,
 ( #53692, #23558, #13528, #32401, #50156, #18272, #45732, #27687, #865, #31520 ),
 .UNSPECIFIED., .F., .F.,
 ( 4, 2, 2, 2, 4 ),
 ( 0.000000000000000000, 0.2499999999999999445, 0.4999999999999998890, 0.7499999999999998890, 1.000000000000000000 ),
 .UNSPECIFIED. ) ;
#45221=VECTOR ( 'NONE', #51014, 1000.000000000000000 ) ;
#45224=CARTESIAN_POINT ( 'NONE',  ( 0.000000000000000000, -90.39999999999999147, 0.000000000000000000 ) ) ;
#45225=CARTESIAN_POINT ( 'NONE',  ( 7.374560639698954034, -77.12291666666664014, 9.596002108778181494 ) ) ;
#45226=ORIENTED_EDGE ( 'NONE', *, *, #20685, .T. ) ;
#45232=CARTESIAN_POINT ( 'NONE',  ( 5.380788203752000953, -76.08505630325268498, 9.804131929786001010 ) ) ;
#45235=CARTESIAN_POINT ( 'NONE',  ( -8.585712843602999911, -77.58711156713900436, 6.927284413728999724 ) ) ;
#45239=CARTESIAN_POINT ( 'NONE',  ( 0.9578316561260999951, -78.89790929493999272, -11.17589679220000143 ) ) ;
#45242=CARTESIAN_POINT ( 'NONE',  ( 2.321691164070382118, -79.80000000000001137, 11.71402344135003304 ) ) ;
#45244=EDGE_CURVE ( 'NONE', #19797, #30600, #30077, .T. ) ;
#45260=CARTESIAN_POINT ( 'NONE',  ( -9.700784073263999829, -78.95701179515099000, 7.398918521605999388 ) ) ;
#45261=CARTESIAN_POINT ( 'NONE',  ( -9.225865441558999791, -76.12195766602600600, -6.449166915282999568 ) ) ;
#45262=CARTESIAN_POINT ( 'NONE',  ( -4.239149814995500698, -78.00726517212316935, 9.879002636546259097 ) ) ;
#45264=CARTESIAN_POINT ( 'NONE',  ( -11.96278216175999987, -78.12964977598299754, 0.6386762756999999624 ) ) ;
#45266=CARTESIAN_POINT ( 'NONE',  ( -10.20076653041301817, -79.07412882710335111, 3.463740470522618242 ) ) ;
#45268=CARTESIAN_POINT ( 'NONE',  ( 3.922593800618577653, -80.94544671216375775, 10.00878386548077259 ) ) ;
#45271=CARTESIAN_POINT ( 'NONE',  ( 5.119217263405000828, -77.72816619513099567, 9.901929871541000239 ) ) ;
#45273=CARTESIAN_POINT ( 'NONE',  ( 4.240563026683999759, -80.61527915106279352, -10.17766115582000097 ) ) ;
#45278=CARTESIAN_POINT ( 'NONE',  ( -9.457500717944000712, -78.31128036874700626, -6.031068363571000290 ) ) ;
#45280=CONICAL_SURFACE ( 'NONE', #19818, 10.93038838648999977, 1.373400766944759877 ) ;
#45283=CARTESIAN_POINT ( 'NONE',  ( -5.045392105209124622, -78.58623691269025358, -9.528847481764330496 ) ) ;
#45285=CIRCLE ( 'NONE', #16992, 9.760776772971999193 ) ;
#45288=CARTESIAN_POINT ( 'NONE',  ( 5.173491034367821761, -77.36110484090335149, -10.64243316413162965 ) ) ;
#45290=CARTESIAN_POINT ( 'NONE',  ( -5.774605976465999824, -77.85874741097399010, -9.668913608825000949 ) ) ;
#45296=CARTESIAN_POINT ( 'NONE',  ( -7.311770087164275012, -80.16592078360770302, -7.880827117992419417 ) ) ;
#45303=CARTESIAN_POINT ( 'NONE',  ( 9.995598443669999611, -79.10464906837700028, -4.933823296771000955 ) ) ;
#45331=CARTESIAN_POINT ( 'NONE',  ( -4.671753383259999559, -76.43689303329699669, 9.830826615545998237 ) ) ;
#45334=CARTESIAN_POINT ( 'NONE',  ( 11.22355342542000045, -80.52296671422550389, 0.9700744431168999427 ) ) ;
#45340=CARTESIAN_POINT ( 'NONE',  ( 7.551392188974999975, -80.14932253944839147, 8.117862728809001283 ) ) ;
#45351=CARTESIAN_POINT ( 'NONE',  ( -3.276646979637814372, -79.49970999519690906, 10.24253291459318582 ) ) ;
#45356=ORIENTED_EDGE ( 'NONE', *, *, #18492, .T. ) ;
#45367=CARTESIAN_POINT ( 'NONE',  ( -0.04724284673262602735, -77.22472299400682516, -10.74995637182052022 ) ) ;
#45368=CARTESIAN_POINT ( 'NONE',  ( 11.36512682855729572, -79.07683455540997386, 3.982123233433208398 ) ) ;
#45374=CARTESIAN_POINT ( 'NONE',  ( -5.246265831776000255, -79.79077097150499753, -10.82514862071000117 ) ) ;
#45377=CARTESIAN_POINT ( 'NONE',  ( -0.03447279853675288414, -80.37527479222850957, 10.79553698213345925 ) ) ;
#45379=CARTESIAN_POINT ( 'NONE',  ( 6.071186539538999227, -78.02411607459599452, 10.40848046910999791 ) ) ;
#45380=ORIENTED_EDGE ( 'NONE', *, *, #18116, .F. ) ;
#45381=ORIENTED_EDGE ( 'NONE', *, *, #53262, .T. ) ;
#45383=EDGE_CURVE ( 'NONE', #8467, #28197, #11094, .T. ) ;
#45393=CARTESIAN_POINT ( 'NONE',  ( -11.51732033666299237, -79.79999999999996874, -3.285645309957324844 ) ) ;
#45398=CARTESIAN_POINT ( 'NONE',  ( -5.687706977064001634, -78.06436792976896299, 10.54353137131000118 ) ) ;
#45411=CARTESIAN_POINT ( 'NONE',  ( -12.00000000000000888, -79.38958333333330586, 1.570796326794847264 ) ) ;
#45413=CARTESIAN_POINT ( 'NONE',  ( -2.717095171052049007, -78.20482081344383118, -10.43411631404385354 ) ) ;
#45419=CARTESIAN_POINT ( 'NONE',  ( -11.90546970521999981, -77.35370790967400012, 3.009247460619000059 ) ) ;
#45426=CARTESIAN_POINT ( 'NONE',  ( 1.803762123692000063, -80.43536808024779816, 10.90775046864000153 ) ) ;
#45435=CARTESIAN_POINT ( 'NONE',  ( 10.55923481294568411, -81.00000000000001421, -3.083916981387107459 ) ) ;
#45455=CARTESIAN_POINT ( 'NONE',  ( 1.305706480705000061, -76.55770918080399667, 12.28344334786000047 ) ) ;
#45475=CARTESIAN_POINT ( 'NONE',  ( -12.00000000000000000, -78.39999999999999147, 0.000000000000000000 ) ) ;
#45485=DIRECTION ( 'NONE',  ( 0.000000000000000000, -1.000000000000000000, 0.000000000000000000 ) ) ;
#45488=CARTESIAN_POINT ( 'NONE',  ( 1.644133925033999910, -78.87275712511198833, 11.70364056775000172 ) ) ;
#45492=CARTESIAN_POINT ( 'NONE',  ( 8.325251318307000048, -80.22061154526829796, -7.061554902978000037 ) ) ;
#45498=CARTESIAN_POINT ( 'NONE',  ( -9.393203674808288994, -77.45833333333330017, 5.413904038987134015 ) ) ;
#45501=CARTESIAN_POINT ( 'NONE',  ( -12.08282522424999961, -75.86276683616600280, 1.641596703183000105 ) ) ;
#45505=CARTESIAN_POINT ( 'NONE',  ( 9.995598443669999611, -78.92237613279000641, -4.933823296771000955 ) ) ;
#45515=CARTESIAN_POINT ( 'NONE',  ( -9.875985572401248191, -76.46666666666662593, 4.392572548563077994 ) ) ;
#45518=CARTESIAN_POINT ( 'NONE',  ( -10.75000000000000000, -79.50000000000000000, 0.000000000000000000 ) ) ;
#45525=CARTESIAN_POINT ( 'NONE',  ( 8.024414491358506041, -78.79212767763318936, -7.157144857178496800 ) ) ;
#45532=CARTESIAN_POINT ( 'NONE',  ( 4.494525810343096950, -77.20555113919044743, -10.87989057085453837 ) ) ;
#45533=CARTESIAN_POINT ( 'NONE',  ( 6.445068773528756623, -77.72010726321535401, -10.09856820804314381 ) ) ;
#45535=CARTESIAN_POINT ( 'NONE',  ( 11.15679540746000065, -79.52434518398199259, 1.159321710118000004 ) ) ;
#45554=CARTESIAN_POINT ( 'NONE',  ( 3.562868568952000548, -79.72528206836099685, 11.91204729721000000 ) ) ;
#45555=CARTESIAN_POINT ( 'NONE',  ( -5.857867859648000497, -76.12642014291699866, 9.889045732754000895 ) ) ;
#45556=CARTESIAN_POINT ( 'NONE',  ( -1.272095873948303257, -77.98448913755433409, 10.68035095373946675 ) ) ;
#45557=CARTESIAN_POINT ( 'NONE',  ( -11.74098051674999965, -78.61797745361100453, 2.380218674853999961 ) ) ;
#45563=CARTESIAN_POINT ( 'NONE',  ( 1.664903097754173888, -80.96299215033094754, 10.62006420670805973 ) ) ;
#45566=CARTESIAN_POINT ( 'NONE',  ( 0.2611009988843999707, -78.58574720659700574, -11.02876811737000118 ) ) ;
#45568=CARTESIAN_POINT ( 'NONE',  ( 4.284808111760000315, -80.54755208664988686, -10.28385259334999979 ) ) ;
#45573=CARTESIAN_POINT ( 'NONE',  ( -3.244487197725999916, -76.79996563637499207, -10.73738397614000029 ) ) ;
#45585=CARTESIAN_POINT ( 'NONE',  ( -11.21475409559999825, -76.76929369090099442, 1.031226285144000165 ) ) ;
#45594=AXIS2_PLACEMENT_3D ( 'NONE', #34573, #44032, #21298 ) ;
#45598=FACE_BOUND ( 'NONE', #52131, .T. ) ;
#45599=CARTESIAN_POINT ( 'NONE',  ( -4.126717922116999837, -79.48595787040198957, -10.35494083817999922 ) ) ;
#45606=ORIENTED_EDGE ( 'NONE', *, *, #3241, .T. ) ;
#45618=DIRECTION ( 'NONE',  ( -0.3090169943748909964, 0.000000000000000000, 0.9510565162951718499 ) ) ;
#45622=ADVANCED_FACE ( 'NONE', ( #20175, #47347 ), #47927, .F. ) ;
#45630=CARTESIAN_POINT ( 'NONE',  ( -6.711381441964999972, -80.19189216818548971, 9.048015653393999713 ) ) ;
#45631=CARTESIAN_POINT ( 'NONE',  ( -12.00000000000000355, -76.78958333333331154, 1.570796326794848596 ) ) ;
#45632=CARTESIAN_POINT ( 'NONE',  ( 0.000000000000000000, -75.15999999999999659, 0.000000000000000000 ) ) ;
#45648=CARTESIAN_POINT ( 'NONE',  ( -3.053122078541150142, -79.49795925471170221, 10.30883018202370671 ) ) ;
#45651=ORIENTED_EDGE ( 'NONE', *, *, #39073, .T. ) ;
#45663=CARTESIAN_POINT ( 'NONE',  ( -2.429273012391383268, -77.20702660129524020, -10.47182961545118651 ) ) ;
#45673=CARTESIAN_POINT ( 'NONE',  ( -5.720894519599999839, -78.10550402086698796, 10.60505245481999914 ) ) ;
#45675=B_SPLINE_CURVE_WITH_KNOTS ( 'NONE', 3,
 ( #52590, #12140, #57301, #52875, #56152, #6551, #20142, #20427, #38129, #24851, #6840, #15701, #33695, #51734, #42866, #2424, #56440, #33982, #15994, #50, #57581, #8283, #8575, #18026 ),
 .UNSPECIFIED., .F., .F.,
 ( 4, 2, 2, 2, 2, 2, 2, 2, 2, 2, 2, 4 ),
 ( 0.000000000000000000, 0.06249999999999991673, 0.1249999999999998335, 0.1874999999999997780, 0.2499999999999997224, 0.3749999999999997224, 0.4999999999999997780, 0.6249999999999997780, 0.7499999999999998890, 0.8749999999999998890, 0.9375000000000000000, 1.000000000000000000 ),
 .UNSPECIFIED. ) ;
#45678=CARTESIAN_POINT ( 'NONE',  ( -8.538789269653864977, -76.46197650723648565, -8.538663626634152237 ) ) ;
#45687=ADVANCED_FACE ( 'NONE', ( #12456 ), #32057, .F. ) ;
#45688=CARTESIAN_POINT ( 'NONE',  ( 11.06808393496999976, -76.52755534788698810, 1.603559079323000125 ) ) ;
#45693=CARTESIAN_POINT ( 'NONE',  ( -11.04404426307000087, -76.30895766602598940, 2.028007672696999997 ) ) ;
#45696=DIRECTION ( 'NONE',  ( 0.000000000000000000, -1.000000000000000000, 0.000000000000000000 ) ) ;
#45714=CARTESIAN_POINT ( 'NONE',  ( -12.00000000000000000, -75.15999999999999659, 0.000000000000000000 ) ) ;
#45717=CARTESIAN_POINT ( 'NONE',  ( 8.048377923311001325, -77.05528544001199975, -9.274674788995000085 ) ) ;
#45718=DIRECTION ( 'NONE',  ( 0.000000000000000000, -1.000000000000000000, 1.021405182655000003E-13 ) ) ;
#45724=CARTESIAN_POINT ( 'NONE',  ( 8.378345960010999960, -79.31039397479999309, -8.487589272848000022 ) ) ;
#45726=CARTESIAN_POINT ( 'NONE',  ( 0.3771049344988000041, -80.08120460502280480, 11.28275838026000066 ) ) ;
#45729=CARTESIAN_POINT ( 'NONE',  ( -7.712695008784000272, -77.39856057395799382, -8.144473358846001432 ) ) ;
#45731=CARTESIAN_POINT ( 'NONE',  ( -10.75000000000000000, -77.50000000000000000, 0.000000000000000000 ) ) ;
#45732=CARTESIAN_POINT ( 'NONE',  ( 10.79124685046503451, -79.80000000000002558, -4.813060917148021645 ) ) ;
#45734=ORIENTED_EDGE ( 'NONE', *, *, #24747, .F. ) ;
#45740=CARTESIAN_POINT ( 'NONE',  ( 0.000000000000000000, -87.70000000000000284, -9.699999999999993960 ) ) ;
#45746=ORIENTED_EDGE ( 'NONE', *, *, #32564, .T. ) ;
#45753=CARTESIAN_POINT ( 'NONE',  ( -5.996189434307000354, -76.03917199503599988, 10.66434391554000172 ) ) ;
#45772=CARTESIAN_POINT ( 'NONE',  ( 12.07535958108000074, -76.93710018766900305, -2.237927141218000404 ) ) ;
#45777=CARTESIAN_POINT ( 'NONE',  ( -8.382198119002001846, -79.80783961780795721, -7.453647783897999979 ) ) ;
#45787=CARTESIAN_POINT ( 'NONE',  ( -5.720894519599999839, -77.92323108527999409, 10.60505245481999914 ) ) ;
#45790=CARTESIAN_POINT ( 'NONE',  ( 8.503062319121001522, -78.76383098776300073, 7.028489548493999983 ) ) ;
#45798=CARTESIAN_POINT ( 'NONE',  ( 11.68767212001978173, -77.67083333333334849, 3.140974612311388192 ) ) ;
#45803=CARTESIAN_POINT ( 'NONE',  ( -0.4120475804594999625, -79.33092127781698366, -11.13933648663000042 ) ) ;
#45805=CARTESIAN_POINT ( 'NONE',  ( -8.970887557736743290, -79.49333017060097006, 7.719903917865763354 ) ) ;
#45820=CARTESIAN_POINT ( 'NONE',  ( 6.916475164548741894, -78.78069308715726038, -8.229583957785196802 ) ) ;
#45827=CARTESIAN_POINT ( 'NONE',  ( 2.080730497819520242, -77.18813522852776998, -11.79602317567259995 ) ) ;
#45829=CARTESIAN_POINT ( 'NONE',  ( 10.89876807034000095, -79.49710884097999042, -2.652350870517000025 ) ) ;
#45830=CARTESIAN_POINT ( 'NONE',  ( 6.010274707836598118, -81.00000000000000000, 9.066665045992072791 ) ) ;
#45839=CARTESIAN_POINT ( 'NONE',  ( -9.596002108778160178, -77.45208333333332007, -7.374560639698984232 ) ) ;
#45851=CARTESIAN_POINT ( 'NONE',  ( 10.48543666025110355, -79.60833333333329165, -6.043427764450775008 ) ) ;
#45852=CARTESIAN_POINT ( 'NONE',  ( -9.946140829862999411, -76.03462989806899941, 5.270939064036999966 ) ) ;
#45853=CARTESIAN_POINT ( 'NONE',  ( -0.06653476265715067839, -77.97558014977887808, 10.74979742560490514 ) ) ;
#45854=CARTESIAN_POINT ( 'NONE',  ( -5.261498566940000288, -77.79049859790299593, -10.76255997729999869 ) ) ;
#45857=CARTESIAN_POINT ( 'NONE',  ( 0.000000000000000000, -87.64999999984398471, 0.000000000000000000 ) ) ;
#45861=CARTESIAN_POINT ( 'NONE',  ( -11.14677829112999952, -77.89158425314199974, -0.06272399197936999460 ) ) ;
#45863=CARTESIAN_POINT ( 'NONE',  ( 10.86022371085000060, -80.72266989507731694, 1.903339784773000032 ) ) ;
#45868=CARTESIAN_POINT ( 'NONE',  ( -11.14038684213999986, -78.25680768274300192, 1.307628137226999998 ) ) ;
#45882=CARTESIAN_POINT ( 'NONE',  ( -12.00000000000000000, -79.29999999999999716, 0.000000000000000000 ) ) ;
#45885=CARTESIAN_POINT ( 'NONE',  ( -10.57946111658618449, -80.11494313127583666, -1.988425045866919927 ) ) ;
#45889=CARTESIAN_POINT ( 'NONE',  ( 0.000000000000000000, 0.000000000000000000, 0.000000000000000000 ) ) ;
#45890=CARTESIAN_POINT ( 'NONE',  ( -5.236138783747000147, -78.80504929535699432, 9.840602177168999987 ) ) ;
#45892=ORIENTED_EDGE ( 'NONE', *, *, #30602, .T. ) ;
#45904=CARTESIAN_POINT ( 'NONE',  ( -2.813789756862251856, -78.10416666666665719, -10.47020627418439709 ) ) ;
#45905=ORIENTED_EDGE ( 'NONE', *, *, #46042, .T. ) ;
#45906=VERTEX_POINT ( 'NONE', #52699 ) ;
#45908=DIRECTION ( 'NONE',  ( -1.000000000000000000, 0.000000000000000000, 0.000000000000000000 ) ) ;
#45911=DIRECTION ( 'NONE',  ( 1.000000000000000000, 0.000000000000000000, 0.000000000000000000 ) ) ;
#45924=CARTESIAN_POINT ( 'NONE',  ( 5.365883907697000410, -80.10159911017460388, 9.905345355165000143 ) ) ;
#45929=CARTESIAN_POINT ( 'NONE',  ( 11.68767212001978173, -78.17083333333334849, 3.140974612311388192 ) ) ;
#45937=EDGE_CURVE ( 'NONE', #24195, #185, #8689, .T. ) ;
#45940=CARTESIAN_POINT ( 'NONE',  ( 6.772653575186247110, -79.42076571837985455, 8.352388374815941319 ) ) ;
#45955=CARTESIAN_POINT ( 'NONE',  ( -6.815894852583468833, -77.17042358260589197, -8.313150857696243179 ) ) ;
#45959=VECTOR ( 'NONE', #18759, 1000.000000000000114 ) ;
#45961=CARTESIAN_POINT ( 'NONE',  ( 10.43959491470999978, -79.84251694161849855, -5.976816984917999953 ) ) ;
#45962=CARTESIAN_POINT ( 'NONE',  ( -7.249533335624161801, -76.09557291620778585, -9.431925875569948658 ) ) ;
#45963=FACE_OUTER_BOUND ( 'NONE', #6657, .T. ) ;
#45966=CARTESIAN_POINT ( 'NONE',  ( 0.4826013546558999279, -77.49519064797900114, 11.92487309688999986 ) ) ;
#45979=CARTESIAN_POINT ( 'NONE',  ( 8.596418555780450887, -80.69791666666667140, -6.606377239730321982 ) ) ;
#45984=CARTESIAN_POINT ( 'NONE',  ( 4.903943924252999409, -76.42722757993099947, -10.05113017056000047 ) ) ;
#45985=FACE_BOUND ( 'NONE', #14290, .T. ) ;
#45986=CARTESIAN_POINT ( 'NONE',  ( -7.726022376260000435, -76.25879378204800219, 8.148147461043999229 ) ) ;
#45995=CYLINDRICAL_SURFACE ( 'NONE', #56054, 10.25000000000000000 ) ;
#46005=LINE ( 'NONE', #45714, #43880 ) ;
#46019=CARTESIAN_POINT ( 'NONE',  ( -7.070160385238000167, -80.84838538950840814, -8.949886881840999564 ) ) ;
#46022=CARTESIAN_POINT ( 'NONE',  ( -3.244487197725999916, -77.00333129620300099, -10.73738397614000029 ) ) ;
#46027=CARTESIAN_POINT ( 'NONE',  ( 7.415475502687034037, -81.00000000000000000, -8.207007851251338693 ) ) ;
#46037=CARTESIAN_POINT ( 'NONE',  ( 11.99915429782999965, -78.59363925020198849, 2.610761444098000261 ) ) ;
#46042=EDGE_CURVE ( 'NONE', #24385, #7885, #38462, .T. ) ;
#46061=CARTESIAN_POINT ( 'NONE',  ( -8.596418555780431348, -77.55208333333331439, -6.606377239730338857 ) ) ;
#46065=CARTESIAN_POINT ( 'NONE',  ( 2.548493721447000038, -76.92447129603100109, 12.01365081398999912 ) ) ;
#46070=CARTESIAN_POINT ( 'NONE',  ( 8.733858618705999888, -78.44602246771752618, -7.038306768505999678 ) ) ;
#46078=CARTESIAN_POINT ( 'NONE',  ( -11.12530226251999999, -77.97748971612699620, 4.628544181647000322 ) ) ;
#46082=CARTESIAN_POINT ( 'NONE',  ( 5.825949712413000192, -80.35679326027729985, 9.232191225927998346 ) ) ;
#46084=VERTEX_POINT ( 'NONE', #15654 ) ;
#46090=CARTESIAN_POINT ( 'NONE',  ( -11.53519992361999869, -75.85018925673099943, 3.464787243407999817 ) ) ;
#46095=CARTESIAN_POINT ( 'NONE',  ( 11.14673908614000020, -78.45935830175899639, 0.06930530262389000828 ) ) ;
#46110=CARTESIAN_POINT ( 'NONE',  ( 6.043427764450761686, -77.13333333333329733, 10.48543666025110888 ) ) ;
#46112=ORIENTED_EDGE ( 'NONE', *, *, #57691, .F. ) ;
#46114=CARTESIAN_POINT ( 'NONE',  ( 9.130635980787438655, -78.80587905097618773, -5.674270332481268220 ) ) ;
#46116=CARTESIAN_POINT ( 'NONE',  ( -10.31421052434999908, -76.72175206120299151, 3.823226550887000030 ) ) ;
#46123=CARTESIAN_POINT ( 'NONE',  ( -10.52651887844270640, -77.00721078521108609, 6.166402933938996966 ) ) ;
#46124=CARTESIAN_POINT ( 'NONE',  ( -7.615957885411051009, -78.47972809508038949, 9.247549774705609238 ) ) ;
#46125=CARTESIAN_POINT ( 'NONE',  ( -2.848564863371000122, -78.87067295193800476, -10.84913769893999991 ) ) ;
#46132=DIRECTION ( 'NONE',  ( 0.000000000000000000, -1.000000000000000000, 0.000000000000000000 ) ) ;
#46134=CARTESIAN_POINT ( 'NONE',  ( 6.043427764450807871, -77.56666666666667709, -10.48543666025108756 ) ) ;
#46144=CARTESIAN_POINT ( 'NONE',  ( -9.886087410963998678, -78.82155766632499194, 7.540251870238000365 ) ) ;
#46145=CARTESIAN_POINT ( 'NONE',  ( -10.85352824271999950, -76.76177769904698778, 2.043985636521999716 ) ) ;
#46146=CARTESIAN_POINT ( 'NONE',  ( 4.666043224853492433, -77.93943897360074402, 9.684446864717223491 ) ) ;
#46147=CARTESIAN_POINT ( 'NONE',  ( -5.261498566940000288, -77.72271004462599819, -10.76255997729999869 ) ) ;
#46152=CARTESIAN_POINT ( 'NONE',  ( 9.340454417440403390, -80.89149709199956817, 5.322469657822352929 ) ) ;
#46155=CARTESIAN_POINT ( 'NONE',  ( 3.871217329169000188, -77.23791202109900667, 10.45314674924000009 ) ) ;
#46157=CARTESIAN_POINT ( 'NONE',  ( 0.5267042291526000675, -80.83006063909182615, 11.01316230888000014 ) ) ;
#46160=CARTESIAN_POINT ( 'NONE',  ( -6.606862979243170564, -80.52715448066929582, 8.596965208648541079 ) ) ;
#46162=CARTESIAN_POINT ( 'NONE',  ( -11.12496554189999998, -77.20851078140199775, -1.432917402686000097 ) ) ;
#46172=CARTESIAN_POINT ( 'NONE',  ( -7.880862184694999328, -76.71482100489700429, 7.737503720428000165 ) ) ;
#46179=CARTESIAN_POINT ( 'NONE',  ( -5.971441230830989433, -80.17821172891612491, -8.938866158933542749 ) ) ;
#46187=CARTESIAN_POINT ( 'NONE',  ( 10.52346617262000095, -78.61439489434398808, -3.675769182893000142 ) ) ;
#46200=CARTESIAN_POINT ( 'NONE',  ( 6.606377239730347739, -78.17708333333328596, -8.596418555780422466 ) ) ;
#46216=CARTESIAN_POINT ( 'NONE',  ( 7.496935112050000072, -80.58316208623270427, 8.408636027568000770 ) ) ;
#46219=CARTESIAN_POINT ( 'NONE',  ( 10.20076089109330120, -76.82412226148122159, -3.463745884883634663 ) ) ;
#46222=CIRCLE ( 'NONE', #37, 9.700000000000001066 ) ;
#46223=CARTESIAN_POINT ( 'NONE',  ( 5.136988255280226845, -77.27767399912663393, -10.56734161811198369 ) ) ;
#46235=CARTESIAN_POINT ( 'NONE',  ( 9.171086888450156849, -79.39389370609096375, 5.639578953327716526 ) ) ;
#46253=CARTESIAN_POINT ( 'NONE',  ( -6.309004353333000026, -79.28274924709700144, -10.24224633278999796 ) ) ;
#46259=CARTESIAN_POINT ( 'NONE',  ( -10.57592698605000159, -78.66175121120100755, -5.530395178621999364 ) ) ;
#46262=AXIS2_PLACEMENT_3D ( 'NONE', #17465, #31023, #21033 ) ;
#46263=CARTESIAN_POINT ( 'NONE',  ( -8.596418555780466875, -78.94791666666665719, 6.606377239730298001 ) ) ;
#46277=CARTESIAN_POINT ( 'NONE',  ( 2.076475668830000121, -76.12624427606199617, 10.98918251355999942 ) ) ;
#46288=DIRECTION ( 'NONE',  ( -1.000000000000000000, 0.000000000000000000, 0.000000000000000000 ) ) ;
#46303=CARTESIAN_POINT ( 'NONE',  ( 6.187157694146999454, -77.70638901018298839, 10.60730214752000045 ) ) ;
#46310=CARTESIAN_POINT ( 'NONE',  ( 7.560470358556999670, -81.02546712712090482, 8.383385420532000865 ) ) ;
#46313=CARTESIAN_POINT ( 'NONE',  ( -5.751434148371999733, -77.98383964426899695, -9.630115047516998317 ) ) ;
#46318=CARTESIAN_POINT ( 'NONE',  ( -10.88020833321164638, -76.16979166665750256, 1.138827338097790687 ) ) ;
#46321=CARTESIAN_POINT ( 'NONE',  ( 11.14639666075000157, -80.93674113700730288, -1.632917082138999776 ) ) ;
#46325=CARTESIAN_POINT ( 'NONE',  ( 6.365665562422999635, -78.73050366622999263, 10.17242851768000023 ) ) ;
#46329=CARTESIAN_POINT ( 'NONE',  ( 1.764045786578000152, -77.46325110754499121, -11.99279291753999921 ) ) ;
#46331=ORIENTED_EDGE ( 'NONE', *, *, #22764, .F. ) ;
#46335=ORIENTED_EDGE ( 'NONE', *, *, #42508, .T. ) ;
#46338=CARTESIAN_POINT ( 'NONE',  ( 10.91479203715999979, -79.82190303803308495, -0.2066369003937000015 ) ) ;
#46347=CARTESIAN_POINT ( 'NONE',  ( -12.00000000000000000, -78.79999999999999716, 0.000000000000000000 ) ) ;
#46357=CARTESIAN_POINT ( 'NONE',  ( -6.620362748380999918, -76.21358782151399680, -10.34376132320999986 ) ) ;
#46364=DIRECTION ( 'NONE',  ( 0.000000000000000000, -1.000000000000000000, 0.000000000000000000 ) ) ;
#46370=CARTESIAN_POINT ( 'NONE',  ( 5.569438312554999548, -78.84562780968799700, 10.68535195481999978 ) ) ;
#46373=CARTESIAN_POINT ( 'NONE',  ( 9.200987374210999548, -79.32181222620799588, 5.875133813785999415 ) ) ;
#46379=CARTESIAN_POINT ( 'NONE',  ( 10.47020627418438643, -77.27083333333332860, 2.813789756862283387 ) ) ;
#46383=CARTESIAN_POINT ( 'NONE',  ( 7.374560639698954922, -77.72291666666666288, 9.596002108778179718 ) ) ;
#46390=CARTESIAN_POINT ( 'NONE',  ( -6.883054871632158900, -79.47416539201856267, 9.627400492276409594 ) ) ;
#46395=CARTESIAN_POINT ( 'NONE',  ( 4.653180395198093677, -79.00894815872477750, -10.20634710234630660 ) ) ;
#46406=CARTESIAN_POINT ( 'NONE',  ( 6.868809838215960362, -78.78024190471647614, -8.269304102357615704 ) ) ;
#46412=CARTESIAN_POINT ( 'NONE',  ( -11.06091447456626398, -78.01852973287638804, 4.601756440133207171 ) ) ;
#46413=CARTESIAN_POINT ( 'NONE',  ( -1.639962962630000076, -78.65278220792400532, 11.09633417262999977 ) ) ;
#46422=CARTESIAN_POINT ( 'NONE',  ( -12.00000000000000178, -77.41041666666669130, -1.570796326794897668 ) ) ;
#46423=EDGE_CURVE ( 'NONE', #41938, #8229, #54412, .T. ) ;
#46424=CARTESIAN_POINT ( 'NONE',  ( 6.043427764450807871, -78.56666666666666288, -10.48543666025108756 ) ) ;
#46430=AXIS2_PLACEMENT_3D ( 'NONE', #6241, #14222, #10391 ) ;
#46434=CARTESIAN_POINT ( 'NONE',  ( -0.5671522757914000401, -78.75204040462999444, 12.42051695972000047 ) ) ;
#46436=CARTESIAN_POINT ( 'NONE',  ( 4.167258872662748637, -77.94352344884244133, 9.911697996766440255 ) ) ;
#46437=CARTESIAN_POINT ( 'NONE',  ( 8.272973658470998970, -78.25176643067300120, -8.664523719228998999 ) ) ;
#46438=CYLINDRICAL_SURFACE ( 'NONE', #10846, 12.00000000000000000 ) ;
#46442=CARTESIAN_POINT ( 'NONE',  ( 9.565389234382577044, -80.88786508125609487, 4.905482548979066770 ) ) ;
#46445=CARTESIAN_POINT ( 'NONE',  ( 0.1369776181910999924, -77.33287542851299179, 11.03100047655000004 ) ) ;
#46446=CARTESIAN_POINT ( 'NONE',  ( 1.298131932841000147, -76.51656913009320249, 12.21218573294999921 ) ) ;
#46447=CARTESIAN_POINT ( 'NONE',  ( 5.335937065057000162, -81.19311224954469708, -9.281131934233000536 ) ) ;
#46451=CARTESIAN_POINT ( 'NONE',  ( 4.139857590833908141, -80.44388087869388926, 9.994141488024814279 ) ) ;
#46452=CARTESIAN_POINT ( 'NONE',  ( -0.8253947190445000137, -77.38524470668500044, -11.18645762290999990 ) ) ;
#46463=CARTESIAN_POINT ( 'NONE',  ( 10.83766451684999943, -77.50467495194999401, -3.062514061775999608 ) ) ;
#46466=CARTESIAN_POINT ( 'NONE',  ( -11.68767212001979594, -77.77916666666665435, 3.140974612311315806 ) ) ;
#46478=CARTESIAN_POINT ( 'NONE',  ( -10.88242774903000054, -79.47197590580999815, -1.809558141819000099 ) ) ;
#46479=LINE ( 'NONE', #24313, #32770 ) ;
#46494=CARTESIAN_POINT ( 'NONE',  ( -8.596418555780431348, -78.05208333333331439, -6.606377239730338857 ) ) ;
#46498=CARTESIAN_POINT ( 'NONE',  ( -12.00000000000000178, -76.90670863885249275, -1.011638905658492460 ) ) ;
#46500=CARTESIAN_POINT ( 'NONE',  ( 8.899186938124000079, -76.04999999999999716, -6.465637775218000094 ) ) ;
#46504=CARTESIAN_POINT ( 'NONE',  ( -11.36512682855694933, -77.32683455540997386, -3.982123233434258669 ) ) ;
#46512=CARTESIAN_POINT ( 'NONE',  ( -8.098718803560510437, -76.65741278108174583, -7.103718760442247593 ) ) ;
#46544=CARTESIAN_POINT ( 'NONE',  ( -6.307673058192007964, -77.17525117048977279, -8.704862286692511830 ) ) ;
#46546=VERTEX_POINT ( 'NONE', #32462 ) ;
#46548=CARTESIAN_POINT ( 'NONE',  ( 8.348735229153000148, -79.01379656946899388, 8.268078378528999295 ) ) ;
#46552=CARTESIAN_POINT ( 'NONE',  ( 9.414842545117998895, -77.82074243306399808, -7.334592169791999794 ) ) ;
#46553=EDGE_CURVE ( 'NONE', #41078, #8467, #15249, .T. ) ;
#46555=ORIENTED_EDGE ( 'NONE', *, *, #14177, .T. ) ;
#46556=CARTESIAN_POINT ( 'NONE',  ( 8.596418555780418913, -78.80208333333332860, 6.606377239730356621 ) ) ;
#46561=ORIENTED_EDGE ( 'NONE', *, *, #48378, .T. ) ;
#46571=CARTESIAN_POINT ( 'NONE',  ( 4.903943924252999409, -76.35943902665499650, -10.05113017056000047 ) ) ;
#46583=CARTESIAN_POINT ( 'NONE',  ( 7.783076670315924872, -76.24921875000657678, 9.115310453498814525 ) ) ;
#46587=CARTESIAN_POINT ( 'NONE',  ( 6.043427764450763462, -79.23333333333330586, 10.48543666025111065 ) ) ;
#46602=CARTESIAN_POINT ( 'NONE',  ( -10.10188948264000075, -80.74568563909183183, -5.039239965656999942 ) ) ;
#46606=CARTESIAN_POINT ( 'NONE',  ( -7.849238557987999521, -76.83991323819199692, 7.706455349885999340 ) ) ;
#46620=CARTESIAN_POINT ( 'NONE',  ( -10.21414511300999983, -77.77975978748899877, 6.816672119949999775 ) ) ;
#46626=CARTESIAN_POINT ( 'NONE',  ( -10.47049301042761016, -77.62083827941357583, -2.813954463924708271 ) ) ;
#46643=CARTESIAN_POINT ( 'NONE',  ( 0.000000000000000000, -75.15999999999999659, 0.000000000000000000 ) ) ;
#46645=CARTESIAN_POINT ( 'NONE',  ( 10.75000000000000000, -77.75000000000000000, 0.000000000000000000 ) ) ;
#46650=CARTESIAN_POINT ( 'NONE',  ( -9.801255020792000394, -76.51464391298200951, 7.399866681860999940 ) ) ;
#46654=CARTESIAN_POINT ( 'NONE',  ( 10.05828973332000054, -78.96351298475168790, -4.964767691657000270 ) ) ;
#46662=CARTESIAN_POINT ( 'NONE',  ( 8.821626479137000487, -78.81849849426399146, 8.208219718620000549 ) ) ;
#46670=CARTESIAN_POINT ( 'NONE',  ( -10.12416963781999968, -79.71218441210199046, 6.728766219208999644 ) ) ;
#46684=ORIENTED_EDGE ( 'NONE', *, *, #25590, .F. ) ;
#46685=CARTESIAN_POINT ( 'NONE',  ( 10.58513040395000004, -78.55432170917399048, 3.845644306921999878 ) ) ;
#46686=CARTESIAN_POINT ( 'NONE',  ( -5.007265642980745390, -76.76182877174545638, 10.00026998867437911 ) ) ;
#46687=CARTESIAN_POINT ( 'NONE',  ( -8.596418555780466875, -79.94791666666667140, 6.606377239730298001 ) ) ;
#46688=DIRECTION ( 'NONE',  ( 0.7071067811864976127, 0.7071067811865975328, -1.603641050304993672E-09 ) ) ;
#46692=CARTESIAN_POINT ( 'NONE',  ( -6.324603895332759684, -78.92723912971976574, -9.263962139975491894 ) ) ;
#46702=CARTESIAN_POINT ( 'NONE',  ( 8.379346636603999698, -77.51281807572799210, -8.651713001682999504 ) ) ;
#46703=CARTESIAN_POINT ( 'NONE',  ( 9.936221582198456304, -78.81890434637429621, -4.102805168011096626 ) ) ;
#46704=ORIENTED_EDGE ( 'NONE', *, *, #26215, .T. ) ;
#46709=EDGE_CURVE ( 'NONE', #39177, #21876, #4588, .T. ) ;
#46712=CARTESIAN_POINT ( 'NONE',  ( -5.687784790578547245, -77.96427110202938593, 10.54367561735933734 ) ) ;
#46713=CARTESIAN_POINT ( 'NONE',  ( 7.808618912244999599, -79.02017053422000004, -8.052551227705000869 ) ) ;
#46721=CARTESIAN_POINT ( 'NONE',  ( -11.12512020565017323, -77.36010185546032858, -1.432937323680165909 ) ) ;
#46722=UNCERTAINTY_MEASURE_WITH_UNIT (LENGTH_MEASURE( 1.000000000000000082E-05 ), #31315, 'distance_accuracy_value', 'NONE');
#46734=CARTESIAN_POINT ( 'NONE',  ( 9.898793482178998460, -76.06315555539499940, 4.898044527662000824 ) ) ;
#46735=CARTESIAN_POINT ( 'NONE',  ( 10.50208737532821246, -77.86721208996137022, 2.298434098163355088 ) ) ;
#46736=CARTESIAN_POINT ( 'NONE',  ( -11.74098051674999965, -78.55018890033399259, 2.380218674853999961 ) ) ;
#46738=CARTESIAN_POINT ( 'NONE',  ( -8.596128373981846593, -79.04808367254781842, 6.606141465317036499 ) ) ;
#46740=CARTESIAN_POINT ( 'NONE',  ( 8.619088907633837948, -80.90150449142340960, 6.437677892227573473 ) ) ;
#46743=CARTESIAN_POINT ( 'NONE',  ( -10.77981876821000107, -77.44182080052098627, 2.344619735928000104 ) ) ;
#46744=CARTESIAN_POINT ( 'NONE',  ( 4.438566736185393324, -77.30575194093574964, -10.90548974299855622 ) ) ;
#46745=CARTESIAN_POINT ( 'NONE',  ( -1.766199577971000023, -80.41452935543939873, 10.76680414263000074 ) ) ;
#46750=EDGE_CURVE ( 'NONE', #51790, #47018, #29699, .T. ) ;
#46751=CARTESIAN_POINT ( 'NONE',  ( 4.013660496580000903, -78.48801429402999474, -10.47417304634999979 ) ) ;
#46763=CARTESIAN_POINT ( 'NONE',  ( 9.909229536192000865, -76.98718443491598862, -5.351741263869000065 ) ) ;
#46775=CARTESIAN_POINT ( 'NONE',  ( 5.530078818784999406, -80.12564813785350282, -9.545677681241999224 ) ) ;
#46777=ORIENTED_EDGE ( 'NONE', *, *, #32881, .F. ) ;
#46780=EDGE_LOOP ( 'NONE', ( #50031, #45356, #6082, #9588 ) ) ;
#46788=CARTESIAN_POINT ( 'NONE',  ( 9.393203674808285442, -78.20833333333334281, -5.413904038987152667 ) ) ;
#46804=CARTESIAN_POINT ( 'NONE',  ( -10.24999999991999999, -82.10000000007899246, 6.817355505960000646E-10 ) ) ;
#46811=CARTESIAN_POINT ( 'NONE',  ( -10.09586848912000079, -78.28687501975998941, 4.990731814912999553 ) ) ;
#46822=CARTESIAN_POINT ( 'NONE',  ( -1.293318857230095320, -79.48473999591016081, 10.67184061187126431 ) ) ;
#46833=CARTESIAN_POINT ( 'NONE',  ( 4.993368691432944040, -80.26375664158507561, -9.522208454640370690 ) ) ;
#46834=CARTESIAN_POINT ( 'NONE',  ( -6.863878448621095529, -77.16995529938667175, -8.273635171295007140 ) ) ;
#46839=CARTESIAN_POINT ( 'NONE',  ( 2.377756013412999803, -79.27472795551499019, -11.79209151100000064 ) ) ;
#46843=CARTESIAN_POINT ( 'NONE',  ( 7.889971116623999414, -77.44093201713099006, 8.954543982858998774 ) ) ;
#46855=DIRECTION ( 'NONE',  ( 1.000000000000000000, 0.000000000000000000, 0.000000000000000000 ) ) ;
#46858=CARTESIAN_POINT ( 'NONE',  ( 11.75000000000000000, -79.79999999999999716, -4.009019365174000020E-13 ) ) ;
#46859=CARTESIAN_POINT ( 'NONE',  ( -10.60742839163532736, -80.08734568579502877, 1.743969048105956876 ) ) ;
#46862=CARTESIAN_POINT ( 'NONE',  ( 9.886069181790999139, -76.47739146390900089, -5.228720670581999741 ) ) ;
#46863=ADVANCED_FACE ( 'NONE', ( #53983 ), #14113, .F. ) ;
#46866=CARTESIAN_POINT ( 'NONE',  ( -1.971120042941999939, -76.43436737597099295, -11.05433917436000080 ) ) ;
#46873=CARTESIAN_POINT ( 'NONE',  ( 12.07833837140000099, -79.82418736905719925, -0.3648754035837999954 ) ) ;
#46874=CARTESIAN_POINT ( 'NONE',  ( -8.845454740156757367, -78.05205573245035566, 6.111140252778515247 ) ) ;
#46879=CARTESIAN_POINT ( 'NONE',  ( 0.000000000000000000, -91.29999999999999716, 0.000000000000000000 ) ) ;
#46893=CARTESIAN_POINT ( 'NONE',  ( 3.773599593829000121, -80.36098609305189200, -10.63964551222000132 ) ) ;
#46897=CARTESIAN_POINT ( 'NONE',  ( 9.070694317316998934, -78.20173038828299639, 6.598531290616000078 ) ) ;
#46912=CARTESIAN_POINT ( 'NONE',  ( -3.132815200277000223, -78.36313629324600072, -11.75448848339000030 ) ) ;
#46914=CARTESIAN_POINT ( 'NONE',  ( 5.195844325042688006, -78.66486225622416839, -9.480952556279184762 ) ) ;
#46919=CARTESIAN_POINT ( 'NONE',  ( 10.47018369756723288, -77.82921409177868100, -2.813855853172428478 ) ) ;
#46923=CARTESIAN_POINT ( 'NONE',  ( 10.26057445098000187, -78.35114051593500051, 3.727731092327000173 ) ) ;
#46941=DIRECTION ( 'NONE',  ( 1.000000000000000000, 0.000000000000000000, 0.000000000000000000 ) ) ;
#46944=CARTESIAN_POINT ( 'NONE',  ( -12.27595451887999900, -76.13162234490400238, 0.3505736730271999391 ) ) ;
#46945=DIRECTION ( 'NONE',  ( 0.000000000000000000, -1.000000000000000000, 0.000000000000000000 ) ) ;
#46955=CARTESIAN_POINT ( 'NONE',  ( -1.368150018649999966, -77.62480861561799372, -11.97179757597999838 ) ) ;
#46970=ORIENTED_EDGE ( 'NONE', *, *, #53943, .F. ) ;
#46972=CARTESIAN_POINT ( 'NONE',  ( 11.20174477810000013, -79.53483005723899169, 1.163992476170999879 ) ) ;
#46986=CARTESIAN_POINT ( 'NONE',  ( -10.48543666025111420, -77.25833333333331154, 6.043427764450754580 ) ) ;
#46988=VERTEX_POINT ( 'NONE', #579 ) ;
#46990=CARTESIAN_POINT ( 'NONE',  ( 1.669271706869820404, -78.73747607613988464, -10.62851245282890744 ) ) ;
#46991=EDGE_CURVE ( 'NONE', #47432, #15756, #50150, .T. ) ;
#46992=ORIENTED_EDGE ( 'NONE', *, *, #3886, .T. ) ;
#46996=CARTESIAN_POINT ( 'NONE',  ( 10.75000000000000000, -79.84999999999999432, -2.184490103126999767E-14 ) ) ;
#46999=CARTESIAN_POINT ( 'NONE',  ( 2.039250879084999912, -80.04123109255959889, -11.02993955029000084 ) ) ;
#47006=CARTESIAN_POINT ( 'NONE',  ( 2.855009615267027900, -78.20442848851632789, 10.84760476142250418 ) ) ;
#47010=CARTESIAN_POINT ( 'NONE',  ( 10.47020627418438643, -80.77083333333332860, 2.813789756862283387 ) ) ;
#47015=CARTESIAN_POINT ( 'NONE',  ( -0.7406579117306999471, -79.52990259888842672, 12.00660533699000077 ) ) ;
#47018=VERTEX_POINT ( 'NONE', #30927 ) ;
#47022=CARTESIAN_POINT ( 'NONE',  ( -11.92766985523999956, -77.64132209835500475, -1.116582401450000095 ) ) ;
#47030=CARTESIAN_POINT ( 'NONE',  ( 11.00720109383000000, -77.71418423053899005, 0.7370606905150999255 ) ) ;
#47032=CARTESIAN_POINT ( 'NONE',  ( -10.02512094469000026, -81.05887381952659609, -4.305871809879999290 ) ) ;
#47038=CARTESIAN_POINT ( 'NONE',  ( -10.93308570624999909, -78.35183257902099285, -2.507139558745000052 ) ) ;
#47042=CARTESIAN_POINT ( 'NONE',  ( -10.43912668352000139, -76.61936152454400428, -6.221750613054999768 ) ) ;
#47062=CARTESIAN_POINT ( 'NONE',  ( -6.103876716051000351, -79.88052105083718857, 9.189364690594999274 ) ) ;
#47076=CARTESIAN_POINT ( 'NONE',  ( -2.710423231297999891, -79.59273834571499151, 10.88447134676999895 ) ) ;
#47078=ORIENTED_EDGE ( 'NONE', *, *, #15329, .F. ) ;
#47092=CARTESIAN_POINT ( 'NONE',  ( 10.68110037031465254, -76.83975127526852589, -1.407209699235823397 ) ) ;
#47098=DIRECTION ( 'NONE',  ( 0.000000000000000000, -1.000000000000000000, 0.000000000000000000 ) ) ;
#47102=CARTESIAN_POINT ( 'NONE',  ( 10.75000000000000000, -79.75000000000000000, 0.000000000000000000 ) ) ;
#47110=CIRCLE ( 'NONE', #15976, 10.34999999999999964 ) ;
#47113=CARTESIAN_POINT ( 'NONE',  ( 6.562466215526181479, -79.42274286776711278, 8.517979315676269536 ) ) ;
#47127=CARTESIAN_POINT ( 'NONE',  ( 4.222689032385934738, -80.25723640890934973, -9.885936313453116853 ) ) ;
#47128=CARTESIAN_POINT ( 'NONE',  ( -6.440114635396656517, -77.17402085401280942, -8.608282088332575910 ) ) ;
#47132=CARTESIAN_POINT ( 'NONE',  ( -8.850953919802000414, -79.62531023410498676, -8.146641040006999290 ) ) ;
#47136=CARTESIAN_POINT ( 'NONE',  ( 3.910274016995999968, -78.47184600323399195, 11.27587067850999958 ) ) ;
#47139=VERTEX_POINT ( 'NONE', #17781 ) ;
#47146=B_SPLINE_CURVE_WITH_KNOTS ( 'NONE', 3,
 ( #29514, #21241, #7667, #25380, #42826, #2678, #34514, #47849, #6512, #16534, #24523, #15662, #52544, #47569, #2389, #57258, #38958, #25668, #51982, #6805 ),
 .UNSPECIFIED., .F., .F.,
 ( 4, 2, 2, 2, 2, 2, 2, 2, 2, 4 ),
 ( 0.000000000000000000, 0.1250000000000000555, 0.2500000000000001110, 0.3750000000000001665, 0.5000000000000002220, 0.5625000000000002220, 0.6250000000000002220, 0.7500000000000002220, 0.8750000000000001110, 1.000000000000000000 ),
 .UNSPECIFIED. ) ;
#47151=CARTESIAN_POINT ( 'NONE',  ( 10.31138940913660385, -79.80000000000002558, 5.792230958630865345 ) ) ;
#47156=CARTESIAN_POINT ( 'NONE',  ( 11.01994305158000031, -76.57026195917399036, -1.906499110313000234 ) ) ;
#47157=CARTESIAN_POINT ( 'NONE',  ( 9.530288639337330281, -76.31250477656314501, -5.032706227462631965 ) ) ;
#47159=CARTESIAN_POINT ( 'NONE',  ( -10.49640831179000067, -76.93768998730399744, 2.856326049988000104 ) ) ;
#47165=CARTESIAN_POINT ( 'NONE',  ( -0.5512063501708999169, -78.95522159786899863, 12.07130450291999857 ) ) ;
#47166=CARTESIAN_POINT ( 'NONE',  ( -8.425013773427030728, -78.04682285271482556, 6.676943546907208926 ) ) ;
#47173=EDGE_CURVE ( 'NONE', #34745, #7885, #48917, .T. ) ;
#47188=CARTESIAN_POINT ( 'NONE',  ( -0.8253947190445000137, -77.52082181323800114, -11.18645762290999990 ) ) ;
#47192=DIRECTION ( 'NONE',  ( -1.000000000000000000, 0.000000000000000000, 0.000000000000000000 ) ) ;
#47205=ORIENTED_EDGE ( 'NONE', *, *, #33377, .T. ) ;
#47206=CARTESIAN_POINT ( 'NONE',  ( -11.23155942826000064, -78.22748971612699620, 4.672751159098000429 ) ) ;
#47215=CARTESIAN_POINT ( 'NONE',  ( -2.772348231745000113, -78.67797663195699442, -10.55885653242000011 ) ) ;
#47218=CARTESIAN_POINT ( 'NONE',  ( 8.595272398064562225, -80.79796620898505921, -6.605316870660081108 ) ) ;
#47228=CARTESIAN_POINT ( 'NONE',  ( 1.407171709420440342, -77.63541666666667140, -10.74999999999999822 ) ) ;
#47234=CARTESIAN_POINT ( 'NONE',  ( -10.51110168222999874, -76.09063960659899806, 6.351495789100000344 ) ) ;
#47243=CARTESIAN_POINT ( 'NONE',  ( 2.713377469415999776, -77.65193793104199926, -11.74024507335000145 ) ) ;
#47248=CARTESIAN_POINT ( 'NONE',  ( -10.54394959781209806, -79.58451761008286951, 2.094245364761433414 ) ) ;
#47261=CARTESIAN_POINT ( 'NONE',  ( 9.492027143945000134, -79.07181222620799588, 6.060972302936999512 ) ) ;
#47263=CARTESIAN_POINT ( 'NONE',  ( 9.019638247444307311, -79.24418804902973079, -7.564637645086659923 ) ) ;
#47276=CARTESIAN_POINT ( 'NONE',  ( 0.000000000000000000, -87.20000000000000284, 0.000000000000000000 ) ) ;
#47280=CARTESIAN_POINT ( 'NONE',  ( -11.12828319551999812, -76.36530140318998860, -5.885103109553999623 ) ) ;
#47281=CARTESIAN_POINT ( 'NONE',  ( 4.725312280198877168, -78.76122478628501256, -9.657371511130047992 ) ) ;
#47287=CARTESIAN_POINT ( 'NONE',  ( 9.392928023032661500, -79.80834514118080847, -5.413658657368042526 ) ) ;
#47290=CARTESIAN_POINT ( 'NONE',  ( -9.735611069857000643, -79.29253396423798961, 5.570995215215999607 ) ) ;
#47298=CARTESIAN_POINT ( 'NONE',  ( 2.187346494202816682, -78.49075902077704825, -10.82308098013309205 ) ) ;
#47301=CARTESIAN_POINT ( 'NONE',  ( -12.00000000000000000, -76.89999999999999147, 0.000000000000000000 ) ) ;
#47312=CARTESIAN_POINT ( 'NONE',  ( 11.53501176087999980, -78.79435273914799609, -3.234124663588000104 ) ) ;
#47320=CARTESIAN_POINT ( 'NONE',  ( -2.271373002040000255, -77.85036594554799194, 10.79548975578000025 ) ) ;
#47322=CARTESIAN_POINT ( 'NONE',  ( 9.568449708939001042, -80.73670158748298320, -5.242933980235000568 ) ) ;
#47330=CARTESIAN_POINT ( 'NONE',  ( 11.19180402071999936, -77.52142642169400233, 0.7494220128532999015 ) ) ;
#47341=COLOUR_RGB ( '', 0.40784314, 0.44705882, 0.49803922) ;
#47347=FACE_OUTER_BOUND ( 'NONE', #38999, .T. ) ;
#47361=CARTESIAN_POINT ( 'NONE',  ( 2.778581917922999800, -77.92792964775300391, 10.55721783972000161 ) ) ;
#47368=DIRECTION ( 'NONE',  ( -1.000000000000000000, 0.000000000000000000, 0.000000000000000000 ) ) ;
#47376=CARTESIAN_POINT ( 'NONE',  ( -1.649952397703835283, -77.41404686049249051, -11.92900123064598183 ) ) ;
#47389=CARTESIAN_POINT ( 'NONE',  ( 0.000000000000000000, -80.79999999999999716, 0.000000000000000000 ) ) ;
#47396=EDGE_CURVE ( 'NONE', #12674, #31055, #18707, .T. ) ;
#47404=CARTESIAN_POINT ( 'NONE',  ( 0.000000000000000000, -75.15999999999999659, 0.000000000000000000 ) ) ;
#47409=CARTESIAN_POINT ( 'NONE',  ( 0.5383385070467999745, -76.77002127708399826, -11.01870799087000030 ) ) ;
#47415=CARTESIAN_POINT ( 'NONE',  ( 6.980956135117539318, -80.28139258642764275, -8.175132495031112612 ) ) ;
#47418=CARTESIAN_POINT ( 'NONE',  ( -0.7406579117306999471, -79.44600844901900416, 12.00660533699000077 ) ) ;
#47432=VERTEX_POINT ( 'NONE', #41974 ) ;
#47439=AXIS2_PLACEMENT_3D ( 'NONE', #36605, #5890, #23899 ) ;
#47440=CARTESIAN_POINT ( 'NONE',  ( -10.04068294437870890, -79.80000000000001137, -6.437684011260381922 ) ) ;
#47441=B_SPLINE_SURFACE_WITH_KNOTS ( 'NONE', 3, 3, ( 
 ( #57668, #39948, #21655, #48824, #8366, #17224, #53243, #16663, #21082, #16947, #52961, #12510, #39662, #12792, #26364, #431, #41420, #44980, #18117, #49414, #50002, #718, #31959, #50581, #54705, #36980, #4827, #41710, #18407, #22826, #14249, #4535, #9548, #32535, #36399, #10135, #54127, #28111, #31664, #23117, #22536, #8962, #1285, #9255, #46162, #27822, #27531, #1003, #18988, #14542, #27240, #40837, #54427, #5687, #50288, #18696, #31369, #23697, #54993, #45573, #36690, #19279, #37269, #36111, #13373, #26947, #32245 ),
 ( #5121, #40545, #41124, #140, #13668, #49710, #45278, #13962, #45868, #9842, #5401, #23409, #38440, #55580, #42885, #34000, #1870, #56169, #56457, #24579, #42303, #43176, #15717, #2731, #52036, #7148, #33713, #51750, #11593, #11300, #51168, #29281, #23987, #33423, #20730, #47330, #25150, #2157, #6270, #28700, #46452, #6859, #1571, #29569, #55284, #24286, #47625, #5980, #19864, #19564, #51460, #24867, #42003, #37858, #42595, #2442, #11014, #20444, #16011, #20158, #38147, #37565, #14832, #32829, #50874, #15128, #10420 ),
 ( #33126, #28405, #46751, #10722, #55879, #15429, #28998, #47038, #6568, #26577, #39307, #43459, #34288, #39594, #13005, #11876, #12158, #39019, #53463, #44611, #57031, #35434, #38728, #4166, #44314, #52322, #57317, #30718, #29854, #16881, #16590, #34862, #8300, #9404, #26802, #40094, #40397, #54852, #49565, #8810, #9111, #30928, #45729, #32111, #48967, #40989, #9694, #35961, #49258, #18561, #36553, #58406, #13226, #8509, #45135, #54575, #289, #50152, #4083, #58108, #17671, #22386, #4970, #35657, #53687, #13820, #31220 ),
 ( #53985, #49861, #4387, #18268, #17969, #27395, #15282, #2304, #51610, #24728, #51317, #10875, #29142, #28846, #10278, #46897, #41569, #51026, #20301, #33276, #42741, #19720, #23844, #46313, #5543, #6424, #19135, #11167, #38296, #41861, #6720, #23553, #1438, #37130, #10575, #24439, #1150, #19429, #14687, #14399, #47188, #1727, #32397, #37421, #55441, #50441, #42453, #37716, #9993, #33572, #2021, #32980, #55738, #27972, #20019, #55141, #38002, #56028, #15577, #46022, #28558, #32688, #50738, #28259, #5838, #14982, #46606 ) ),
 .UNSPECIFIED., .F., .F., .F.,
 ( 4, 4 ),
 ( 4, 1, 1, 1, 1, 1, 1, 1, 1, 1, 1, 1, 1, 1, 1, 1, 1, 1, 1, 1, 1, 1, 1, 1, 1, 1, 1, 1, 1, 1, 1, 1, 1, 1, 1, 1, 1, 1, 1, 1, 1, 1, 1, 1, 1, 1, 1, 1, 1, 1, 1, 1, 1, 1, 1, 1, 1, 1, 1, 1, 1, 1, 1, 1, 4 ),
 ( -0.5168282991433000850, 1.516828299142999992 ),
 ( -0.02000000000000000042, -0.003749999999999999861, 0.01250000000000000069, 0.02875000000000000125, 0.04499999999999999833, 0.06124999999999999889, 0.07749999999999999944, 0.09375000000000000000, 0.1100000000000000006, 0.1262500000000000011, 0.1424999999999999878, 0.1587500000000000022, 0.1749999999999999889, 0.1912500000000000033, 0.2074999999999999900, 0.2237500000000000044, 0.2399999999999999911, 0.2562499999999999778, 0.2725000000000000200, 0.2887500000000000067, 0.3049999999999999933, 0.3212499999999999800, 0.3375000000000000222, 0.3537500000000000089, 0.3699999999999999956, 0.3862499999999999822, 0.4025000000000000244, 0.4187500000000000111, 0.4349999999999999978, 0.4512499999999999845, 0.4675000000000000266, 0.4837500000000000133, 0.5000000000000000000, 0.5162499999999999867, 0.5324999999999999734, 0.5487499999999999600, 0.5649999999999999467, 0.5812500000000000444, 0.5975000000000000311, 0.6137500000000000178, 0.6300000000000000044, 0.6462499999999999911, 0.6624999999999999778, 0.6787499999999999645, 0.6949999999999999512, 0.7112500000000000488, 0.7275000000000000355, 0.7437500000000000222, 0.7600000000000000089, 0.7762499999999999956, 0.7924999999999999822, 0.8087499999999999689, 0.8249999999999999556, 0.8412500000000000533, 0.8575000000000000400, 0.8737500000000000266, 0.8900000000000000133, 0.9062500000000000000, 0.9224999999999999867, 0.9387499999999999734, 0.9549999999999999600, 0.9712499999999999467, 0.9875000000000000444, 1.003749999999999920, 1.020000000000000018 ),
 .UNSPECIFIED. ) ;
#47442=ADVANCED_FACE ( 'NONE', ( #50844 ), #50262, .F. ) ;
#47443=CARTESIAN_POINT ( 'NONE',  ( -10.09223574029775783, -80.07210543507824241, 3.703295250976208486 ) ) ;
#47446=CARTESIAN_POINT ( 'NONE',  ( 1.849737152796000039, -76.76346022239599165, 11.02961253862999946 ) ) ;
#47447=CARTESIAN_POINT ( 'NONE',  ( 10.13752626742690666, -76.38035237456122672, 3.893437952651892076 ) ) ;
#47449=B_SPLINE_CURVE_WITH_KNOTS ( 'NONE', 3,
 ( #40476, #31301, #49344, #12730, #4756, #54065, #9185, #8890, #53771, #44909, #58189, #18341, #31010, #21593, #8305, #27171, #13896, #31890 ),
 .UNSPECIFIED., .F., .F.,
 ( 4, 2, 2, 2, 2, 2, 2, 2, 4 ),
 ( 0.000000000000000000, 0.1250000000000000278, 0.2500000000000000555, 0.3750000000000001110, 0.5000000000000001110, 0.6250000000000001110, 0.7500000000000002220, 0.8750000000000001110, 1.000000000000000000 ),
 .UNSPECIFIED. ) ;
#47452=CARTESIAN_POINT ( 'NONE',  ( 5.145480625322999657, -76.72783191828600025, 9.851073647752999207 ) ) ;
#47459=CARTESIAN_POINT ( 'NONE',  ( 6.473318383219999639, -79.33935673447399495, 10.34143508852999815 ) ) ;
#47461=CARTESIAN_POINT ( 'NONE',  ( -10.74994593004994137, -78.09660187553588173, 0.4712215136974609586 ) ) ;
#47468=CARTESIAN_POINT ( 'NONE',  ( 6.606377239730315765, -80.17708333333334281, -8.596418555780452664 ) ) ;
#47469=CARTESIAN_POINT ( 'NONE',  ( -3.882040082920266588, -79.20112713863417753, 11.40455788431460249 ) ) ;
#47478=CARTESIAN_POINT ( 'NONE',  ( 5.620590082324000036, -80.41656716774588176, -9.763102121971000358 ) ) ;
#47482=CARTESIAN_POINT ( 'NONE',  ( 0.000000000000000000, -76.00000000000000000, 0.000000000000000000 ) ) ;
#47496=CARTESIAN_POINT ( 'NONE',  ( -7.347140770713999736, -77.75263047206500744, 9.839476697348001011 ) ) ;
#47499=ORIENTED_EDGE ( 'NONE', *, *, #17943, .F. ) ;
#47500=ORIENTED_EDGE ( 'NONE', *, *, #14163, .F. ) ;
#47505=CARTESIAN_POINT ( 'NONE',  ( 5.414045489727194571, -77.76670134806883539, -9.393387330184902240 ) ) ;
#47509=CARTESIAN_POINT ( 'NONE',  ( 2.120986319506000140, -78.43284954493999805, 10.70872462160000005 ) ) ;
#47518=CARTESIAN_POINT ( 'NONE',  ( -5.374516262939114775, -80.26463862341171307, 9.838658862348587775 ) ) ;
#47541=CARTESIAN_POINT ( 'NONE',  ( -0.08650930969203998733, -78.31670238307098941, 12.16449944406000050 ) ) ;
#47554=CARTESIAN_POINT ( 'NONE',  ( -12.00000000000000178, -77.91041666666669130, -1.570796326794897668 ) ) ;
#47557=CARTESIAN_POINT ( 'NONE',  ( -2.860041384466000203, -78.88115782519599861, -10.89284755413000028 ) ) ;
#47559=CARTESIAN_POINT ( 'NONE',  ( 8.681769470831671498, -79.35917672052410410, 8.041084891514902466 ) ) ;
#47566=B_SPLINE_CURVE_WITH_KNOTS ( 'NONE', 3,
 ( #5505, #55394, #37380, #14940, #45979, #42412, #33531, #23514, #28808, #28216, #32643, #55989, #23229, #24398, #32356, #54815, #1393, #1110 ),
 .UNSPECIFIED., .F., .F.,
 ( 4, 2, 2, 2, 2, 2, 2, 2, 4 ),
 ( 0.000000000000000000, 0.1250000000000000000, 0.2499999999999999722, 0.3750000000000000000, 0.5000000000000000000, 0.6250000000000000000, 0.7500000000000000000, 0.8750000000000000000, 1.000000000000000000 ),
 .UNSPECIFIED. ) ;
#47568=DIRECTION ( 'NONE',  ( 0.9999896828222031298, 0.000000000000000000, 0.004542493714850020202 ) ) ;
#47569=CARTESIAN_POINT ( 'NONE',  ( 5.413886177876668704, -78.43335082942924430, 9.393028503726839062 ) ) ;
#47572=ORIENTED_EDGE ( 'NONE', *, *, #28091, .T. ) ;
#47573=VERTEX_POINT ( 'NONE', #16560 ) ;
#47574=CARTESIAN_POINT ( 'NONE',  ( 5.543805526018000585, -76.42052255369199543, -11.17061805242999917 ) ) ;
#47575=CARTESIAN_POINT ( 'NONE',  ( 2.531064403381080297, -78.74405570548175604, -10.44842218354998842 ) ) ;
#47586=CARTESIAN_POINT ( 'NONE',  ( 8.645668071321999548, -78.63886173219398756, 7.146365085715999044 ) ) ;
#47593=CARTESIAN_POINT ( 'NONE',  ( -11.21684559259269065, -77.85035602949233180, -0.06311826741395569484 ) ) ;
#47609=CARTESIAN_POINT ( 'NONE',  ( -7.167604382870000457, -77.49214559880800834, 9.599037027053000770 ) ) ;
#47611=CARTESIAN_POINT ( 'NONE',  ( 8.547507901081861093, -78.90223080703543701, 6.557426330200511799 ) ) ;
#47616=CARTESIAN_POINT ( 'NONE',  ( -3.190971086128000067, -77.06051199849498801, -10.56027646911999973 ) ) ;
#47625=CARTESIAN_POINT ( 'NONE',  ( -9.524774638983998898, -77.22182664867399637, 5.924253427062000199 ) ) ;
#47630=CARTESIAN_POINT ( 'NONE',  ( -12.13371464510999864, -77.07215438420399778, 0.6771217750942000180 ) ) ;
#47650=ORIENTED_EDGE ( 'NONE', *, *, #30602, .F. ) ;
#47653=CARTESIAN_POINT ( 'NONE',  ( 10.47129194184999967, -77.84622061874799215, 3.086650459461000473 ) ) ;
#47659=CARTESIAN_POINT ( 'NONE',  ( 0.8479846733620011179, -76.25703125043162345, -10.79296874152367991 ) ) ;
#47661=ADVANCED_FACE ( 'NONE', ( #15688 ), #11273, .F. ) ;
#47673=EDGE_CURVE ( 'NONE', #4324, #28272, #29826, .T. ) ;
#47677=CARTESIAN_POINT ( 'NONE',  ( 4.899854808515000215, -78.36021422180199636, -10.93194800986000104 ) ) ;
#47691=CARTESIAN_POINT ( 'NONE',  ( 5.413775304621431417, -76.93349803630370332, 9.393090362380020153 ) ) ;
#47698=CARTESIAN_POINT ( 'NONE',  ( -9.833855776131001036, -77.17856642211100393, -4.999701486664000605 ) ) ;
#47707=CARTESIAN_POINT ( 'NONE',  ( 5.622902522875882880, -80.01669284979236352, -9.705904178814742878 ) ) ;
#47708=CARTESIAN_POINT ( 'NONE',  ( -2.112861425255000203, -79.17705577139200557, -11.84242215301999934 ) ) ;
#47710=CARTESIAN_POINT ( 'NONE',  ( 8.588590363140999884, -80.01743035202939325, -7.284921508032001114 ) ) ;
#47715=CYLINDRICAL_SURFACE ( 'NONE', #10338, 11.59999999999999964 ) ;
#47724=ADVANCED_FACE ( 'NONE', ( #7122 ), #43425, .T. ) ;
#47728=CARTESIAN_POINT ( 'NONE',  ( -8.123805058510761512, -80.04318495892768226, 7.052709536781835098 ) ) ;
#47731=CARTESIAN_POINT ( 'NONE',  ( 4.903943924252999409, -76.56280468648299120, -10.05113017056000047 ) ) ;
#47735=CARTESIAN_POINT ( 'NONE',  ( 8.366417051415998785, -76.01633500948599931, -7.302494661396999653 ) ) ;
#47739=DIRECTION ( 'NONE',  ( -0.9999813732757145690, 0.000000000000000000, 0.006103531896856088240 ) ) ;
#47743=CARTESIAN_POINT ( 'NONE',  ( 9.700000000000001066, -87.20000000000000284, 0.000000000000000000 ) ) ;
#47748=CARTESIAN_POINT ( 'NONE',  ( 1.407171709420409478, -80.13541666666665719, -10.75000000000000000 ) ) ;
#47757=FACE_OUTER_BOUND ( 'NONE', #53635, .T. ) ;
#47758=CARTESIAN_POINT ( 'NONE',  ( -10.94304050380999982, -80.25384972744670620, 3.215197110691000226 ) ) ;
#47762=FACE_OUTER_BOUND ( 'NONE', #6516, .T. ) ;
#47765=CARTESIAN_POINT ( 'NONE',  ( 4.314091565978001697, -79.94225553412998408, 9.846348350499049218 ) ) ;
#47770=CARTESIAN_POINT ( 'NONE',  ( 10.44328705206031316, -77.33088393209217770, -2.574374161856753052 ) ) ;
#47782=ORIENTED_EDGE ( 'NONE', *, *, #46750, .T. ) ;
#47788=EDGE_LOOP ( 'NONE', ( #25835, #19240, #45188, #13875 ) ) ;
#47796=CARTESIAN_POINT ( 'NONE',  ( 7.413727788746441227, -80.66735391346617234, 8.409593088671112326 ) ) ;
#47797=CARTESIAN_POINT ( 'NONE',  ( 3.249499231399000099, -78.79685944621013505, -11.53069031867000049 ) ) ;
#47817=CARTESIAN_POINT ( 'NONE',  ( 10.98749645531832364, -78.68354319426249788, 4.929334125397527799 ) ) ;
#47819=CARTESIAN_POINT ( 'NONE',  ( 10.48586718643000104, -77.21786888426198914, -5.936521791247999502 ) ) ;
#47828=CARTESIAN_POINT ( 'NONE',  ( 7.730712852075999564, -79.57901625786399791, 9.381427633351998807 ) ) ;
#47830=CARTESIAN_POINT ( 'NONE',  ( 2.808087910937577814, -79.75624999999999432, 11.70482407730010799 ) ) ;
#47832=DIRECTION ( 'NONE',  ( -1.000000000000000000, 0.000000000000000000, 0.000000000000000000 ) ) ;
#47836=EDGE_LOOP ( 'NONE', ( #21683, #28717, #1156, #50610 ) ) ;
#47838=CARTESIAN_POINT ( 'NONE',  ( 2.595923711085492247, -79.40708866698008705, 11.48131793224416697 ) ) ;
#47849=CARTESIAN_POINT ( 'NONE',  ( -2.813605875113437182, -78.49586331468553624, 10.46960120928732607 ) ) ;
#47854=CARTESIAN_POINT ( 'NONE',  ( 11.90218195501999965, -77.10299069267900052, 4.100124956475999838 ) ) ;
#47855=CARTESIAN_POINT ( 'NONE',  ( 5.166696889923573011, -78.76497110610900165, -9.426996544925714261 ) ) ;
#47865=CARTESIAN_POINT ( 'NONE',  ( 5.986115112277999195, -80.23188549357229249, 9.486000076385000312 ) ) ;
#47874=CARTESIAN_POINT ( 'NONE',  ( 7.199925632633625838, -77.16944745444732234, 8.601318494760706201 ) ) ;
#47878=CARTESIAN_POINT ( 'NONE',  ( -2.813789756862300262, -80.89583333333328596, 10.47020627418438465 ) ) ;
#47891=CARTESIAN_POINT ( 'NONE',  ( 1.634596122093999959, -78.86221076299099764, 11.63574645295999943 ) ) ;
#47899=CARTESIAN_POINT ( 'NONE',  ( -4.410648470793000264, -77.61849323694099212, -9.986067597275999574 ) ) ;
#47906=CARTESIAN_POINT ( 'NONE',  ( -2.904336368201000163, -79.22060522871599630, 11.92263291878999887 ) ) ;
#47916=ORIENTED_EDGE ( 'NONE', *, *, #56573, .F. ) ;
#47917=CARTESIAN_POINT ( 'NONE',  ( -2.693529710394999999, -79.60328470783500165, 10.81663063389000001 ) ) ;
#47927=PLANE ( 'NONE',  #7046 ) ;
#47938=CARTESIAN_POINT ( 'NONE',  ( -2.181032210905110791, -81.00000000000000000, -10.72093034226582553 ) ) ;
#47944=CARTESIAN_POINT ( 'NONE',  ( 8.696932689530999738, -76.29999999999999716, -6.318691462144000681 ) ) ;
#47949=EDGE_CURVE ( 'NONE', #8361, #22144, #29137, .T. ) ;
#47958=FACE_OUTER_BOUND ( 'NONE', #5298, .T. ) ;
#47960=CARTESIAN_POINT ( 'NONE',  ( -5.687706977064000746, -78.11605038298799286, 10.54353137130999940 ) ) ;
#47965=CARTESIAN_POINT ( 'NONE',  ( 10.33259770149999923, -77.60596644471499417, 4.480110411294999651 ) ) ;
#47969=CARTESIAN_POINT ( 'NONE',  ( 10.26995137457921636, -80.27463911791144824, 3.283750080291039986 ) ) ;
#47982=EDGE_CURVE ( 'NONE', #22708, #43698, #31955, .T. ) ;
#47984=CARTESIAN_POINT ( 'NONE',  ( 6.163257195008000622, -78.38114111159998743, -9.114053931137998887 ) ) ;
#47991=CARTESIAN_POINT ( 'NONE',  ( 5.974268513220012622, -80.27235878227935473, -8.936697743355807688 ) ) ;
#47994=ORIENTED_EDGE ( 'NONE', *, *, #1949, .F. ) ;
#47995=CARTESIAN_POINT ( 'NONE',  ( 3.714552462503000196, -79.34833626489600533, 11.44155784250999908 ) ) ;
#47998=CARTESIAN_POINT ( 'NONE',  ( 10.09881335831000015, -79.03692200396399414, -4.984770136353999348 ) ) ;
#48004=DIRECTION ( 'NONE',  ( -1.000000000000000000, 0.000000000000000000, 0.000000000000000000 ) ) ;
#48015=CARTESIAN_POINT ( 'NONE',  ( 4.976371158049889942, -79.80000000000001137, 10.82108306336006720 ) ) ;
#48017=CARTESIAN_POINT ( 'NONE',  ( -10.20761871445822244, -80.07464919416229066, 3.371456631957987948 ) ) ;
#48021=CARTESIAN_POINT ( 'NONE',  ( 7.778176538613999824, -76.52009807519600315, -8.035785801754000701 ) ) ;
#48024=CARTESIAN_POINT ( 'NONE',  ( 9.963260314060999434, -76.67766803430798461, 4.924740193090999085 ) ) ;
#48033=CARTESIAN_POINT ( 'NONE',  ( -2.524762559494834413, -77.99400743061801222, 10.44993185993495999 ) ) ;
#48042=DIRECTION ( 'NONE',  ( 0.000000000000000000, 1.000000000000000000, 0.000000000000000000 ) ) ;
#48058=CARTESIAN_POINT ( 'NONE',  ( 0.000000000000000000, -87.70000000000000284, 0.000000000000000000 ) ) ;
#48061=CARTESIAN_POINT ( 'NONE',  ( 8.473210114131379811, -77.29736020677133013, -6.623708463630019416 ) ) ;
#48071=CARTESIAN_POINT ( 'NONE',  ( -3.600395895414000069, -77.65777409222799577, 11.61979689923000159 ) ) ;
#48087=CARTESIAN_POINT ( 'NONE',  ( 6.233047529871999615, -78.98050366622999263, 9.960502923565000444 ) ) ;
#48091=EDGE_CURVE ( 'NONE', #57578, #5899, #16328, .T. ) ;
#48095=CARTESIAN_POINT ( 'NONE',  ( 7.144724566336000393, -76.32390714479099358, 9.988770583665001368 ) ) ;
#48100=DIRECTION ( 'NONE',  ( 0.000000000000000000, -1.000000000000000000, 0.000000000000000000 ) ) ;
#48101=CARTESIAN_POINT ( 'NONE',  ( 6.365665562422999635, -78.73050366622999263, 10.17242851768000023 ) ) ;
#48103=AXIS2_PLACEMENT_3D ( 'NONE', #45224, #18063, #57910 ) ;
#48104=CARTESIAN_POINT ( 'NONE',  ( -5.292199200464000164, -77.59767930019499715, -10.82535908394999957 ) ) ;
#48112=CARTESIAN_POINT ( 'NONE',  ( 0.2390640603075999959, -79.56455645514600405, 12.03889950388999885 ) ) ;
#48116=CARTESIAN_POINT ( 'NONE',  ( -5.449838856306469026, -76.22708333364460032, -9.457243427908759159 ) ) ;
#48120=CARTESIAN_POINT ( 'NONE',  ( -11.59999999999999964, -87.70000000000000284, 0.000000000000000000 ) ) ;
#48123=CARTESIAN_POINT ( 'NONE',  ( 7.514114347650544978, -79.22981446509285774, -9.060189168767688983 ) ) ;
#48133=EDGE_CURVE ( 'NONE', #55386, #10196, #8022, .T. ) ;
#48139=CARTESIAN_POINT ( 'NONE',  ( -12.58344645258000050, -76.32431866488499850, 0.3593549516198999982 ) ) ;
#48141=CARTESIAN_POINT ( 'NONE',  ( 0.2431151423990842164, -78.72686878867834537, -10.74764302140133765 ) ) ;
#48152=CARTESIAN_POINT ( 'NONE',  ( 8.733858618705999888, -78.59770491346299082, -7.038306768505999678 ) ) ;
#48156=EDGE_LOOP ( 'NONE', ( #31833, #12970, #40277, #3119, #19929, #16843, #48531, #53198, #11694, #50478, #3617 ) ) ;
#48162=EDGE_CURVE ( 'NONE', #41200, #20196, #4472, .T. ) ;
#48174=ORIENTED_EDGE ( 'NONE', *, *, #53542, .T. ) ;
#48178=CARTESIAN_POINT ( 'NONE',  ( 1.720939166139000109, -77.20276623428699736, -11.69973432676000158 ) ) ;
#48198=CARTESIAN_POINT ( 'NONE',  ( 9.414259929411999295, -76.63483834893800406, -8.050387765842000221 ) ) ;
#48203=CARTESIAN_POINT ( 'NONE',  ( 7.861046360898000351, -79.52157567883000411, 7.903072230637000040 ) ) ;
#48207=DIRECTION ( 'NONE',  ( -1.000000000000000000, 0.000000000000000000, -3.332495962870000189E-11 ) ) ;
#48218=ORIENTED_EDGE ( 'NONE', *, *, #34951, .F. ) ;
#48224=CARTESIAN_POINT ( 'NONE',  ( -9.611543720960897375, -81.00000000000001421, -4.953819405574181545 ) ) ;
#48225=CARTESIAN_POINT ( 'NONE',  ( -2.247674004742000076, -77.46491181672199389, 10.68285203299000052 ) ) ;
#48245=CARTESIAN_POINT ( 'NONE',  ( 6.444980599754999595, -77.87188654417400357, -10.09843005143000028 ) ) ;
#48251=CARTESIAN_POINT ( 'NONE',  ( -3.491544874602000359, -78.49078379918199744, -10.58601217070000189 ) ) ;
#48257=DIRECTION ( 'NONE',  ( -2.044813970925000100E-13, 0.000000000000000000, 1.000000000000000000 ) ) ;
#48271=CARTESIAN_POINT ( 'NONE',  ( -4.457153411444000568, -77.23303910811499406, -10.09135857296999994 ) ) ;
#48277=CARTESIAN_POINT ( 'NONE',  ( 2.326191296373886885, -80.24266891153970960, -10.49546658612705841 ) ) ;
#48279=CARTESIAN_POINT ( 'NONE',  ( -6.206331755963327090, -79.77156576277585032, 9.343610388852424009 ) ) ;
#48280=CARTESIAN_POINT ( 'NONE',  ( -11.22206352833000054, -79.52763804998100738, -4.332716936452000844 ) ) ;
#48282=CARTESIAN_POINT ( 'NONE',  ( -4.169330562119000660, -79.41823080598898343, -10.46186633551000078 ) ) ;
#48298=CARTESIAN_POINT ( 'NONE',  ( -4.834103127707872538, -80.01221937575003551, 9.601684949764214494 ) ) ;
#48301=CARTESIAN_POINT ( 'NONE',  ( 11.09875712452000052, -76.09370506138100154, 1.375294608629999971 ) ) ;
#48306=CARTESIAN_POINT ( 'NONE',  ( 1.536913952029000052, -76.52717638237299980, -11.00715755867000034 ) ) ;
#48317=CARTESIAN_POINT ( 'NONE',  ( 10.75000000000000000, -80.25000000000000000, -1.651583051307000043E-14 ) ) ;
#48332=CARTESIAN_POINT ( 'NONE',  ( 1.570796326794910547, -79.03541666666664867, -11.99999999999999822 ) ) ;
#48335=CARTESIAN_POINT ( 'NONE',  ( 4.280065084278556142, -79.94253482840156266, 9.861166758580704794 ) ) ;
#48339=LINE ( 'NONE', #30591, #33371 ) ;
#48344=CARTESIAN_POINT ( 'NONE',  ( 9.599999999999999645, -92.13603921945998820, 0.000000000000000000 ) ) ;
#48347=CARTESIAN_POINT ( 'NONE',  ( -11.03570087982000025, -77.79342066934700028, -5.118186854384000561 ) ) ;
#48374=CARTESIAN_POINT ( 'NONE',  ( -12.17466003208999936, -76.48783809801099665, 1.612538369963999907 ) ) ;
#48378=EDGE_CURVE ( 'NONE', #23335, #8076, #39856, .T. ) ;
#48385=CARTESIAN_POINT ( 'NONE',  ( 5.022587898441999599, -78.03194079526799953, -11.20577484976000093 ) ) ;
#48390=CARTESIAN_POINT ( 'NONE',  ( -8.951034867792523997, -79.55334570058815302, 5.953222655899479854 ) ) ;
#48394=CARTESIAN_POINT ( 'NONE',  ( 5.174923306164999737, -79.35148740836599757, -10.87255359444000113 ) ) ;
#48396=CARTESIAN_POINT ( 'NONE',  ( -0.001936697166661765362, -79.77500000000000568, 12.03695396042130561 ) ) ;
#48403=AXIS2_PLACEMENT_3D ( 'NONE', #20728, #52321, #3304 ) ;
#48418=EDGE_LOOP ( 'NONE', ( #55313, #42179, #24171, #8111 ) ) ;
#48420=CARTESIAN_POINT ( 'NONE',  ( 7.255050800794000665, -76.58445350691199849, 10.14301354085000106 ) ) ;
#48421=CARTESIAN_POINT ( 'NONE',  ( -10.36620373394242911, -78.62142715943907945, -2.852891701318189810 ) ) ;
#48430=CARTESIAN_POINT ( 'NONE',  ( -8.382198119002001846, -79.95952206355410397, -7.453647783897999979 ) ) ;
#48434=EDGE_CURVE ( 'NONE', #53816, #22708, #27145, .T. ) ;
#48438=AXIS2_PLACEMENT_3D ( 'NONE', #13110, #21686, #44717 ) ;
#48455=CARTESIAN_POINT ( 'NONE',  ( -4.085659785884999451, -78.40101240078699618, 11.26159174134999930 ) ) ;
#48466=CARTESIAN_POINT ( 'NONE',  ( -2.739513636030999955, -79.43367427549699755, -11.96158333944000063 ) ) ;
#48471=CARTESIAN_POINT ( 'NONE',  ( -12.18147860638999980, -75.95564905944900147, -2.246276167021000081 ) ) ;
#48475=CARTESIAN_POINT ( 'NONE',  ( 3.449307203194000415, -78.99083078338598796, 10.47874105986000082 ) ) ;
#48482=CARTESIAN_POINT ( 'NONE',  ( 2.269106295766999856E-14, -92.56607767729998670, 0.000000000000000000 ) ) ;
#48484=DIRECTION ( 'NONE',  ( -1.000000000000000000, 0.000000000000000000, 0.000000000000000000 ) ) ;
#48488=EDGE_CURVE ( 'NONE', #9151, #30430, #53834, .T. ) ;
#48498=CARTESIAN_POINT ( 'NONE',  ( -6.807885647488862269, -81.00000000000001421, -8.483415954689156990 ) ) ;
#48499=CARTESIAN_POINT ( 'NONE',  ( -5.702669450565000631, -77.49214815972399606, 9.308862826782998923 ) ) ;
#48501=CARTESIAN_POINT ( 'NONE',  ( -10.34326456654000026, -78.66670268365299989, 4.339929572939999147 ) ) ;
#48518=CARTESIAN_POINT ( 'NONE',  ( 10.79000226207000068, -79.78942873821000603, -5.440152796310999683 ) ) ;
#48521=CARTESIAN_POINT ( 'NONE',  ( -4.085659785884999451, -78.60437806061599986, 11.26159174134999930 ) ) ;
#48528=CARTESIAN_POINT ( 'NONE',  ( 11.23689443680000011, -77.57873010171299200, 0.7524413429202000403 ) ) ;
#48530=CARTESIAN_POINT ( 'NONE',  ( -10.38445589244000011, -80.29189122021149672, 4.342440965381999973 ) ) ;
#48531=ORIENTED_EDGE ( 'NONE', *, *, #18449, .F. ) ;
#48538=CARTESIAN_POINT ( 'NONE',  ( -10.40651698430760419, -77.07932101869644725, 2.787361001673857253 ) ) ;
#48548=CARTESIAN_POINT ( 'NONE',  ( -7.755223252044999960, -78.14509280558399951, 8.006941543446998821 ) ) ;
#48554=DIRECTION ( 'NONE',  ( 0.7071067811865975328, 0.7071067811864976127, -1.603641050304993672E-09 ) ) ;
#48555=CARTESIAN_POINT ( 'NONE',  ( 4.141311620441085140, -80.25655908808295180, -9.920226166596769701 ) ) ;
#48560=CARTESIAN_POINT ( 'NONE',  ( 11.66950233118999947, -79.22880174150600396, -2.920592611544999606 ) ) ;
#48563=CARTESIAN_POINT ( 'NONE',  ( 6.010232441408999371, -80.15361206703849462, 9.524218016016000377 ) ) ;
#48564=CARTESIAN_POINT ( 'NONE',  ( -6.557200067333805116, -77.52710381399123207, 8.547272894749051275 ) ) ;
#48574=CARTESIAN_POINT ( 'NONE',  ( -10.11939726227999969, -79.60401229401898604, -4.095505467953000078 ) ) ;
#48577=ORIENTED_EDGE ( 'NONE', *, *, #17980, .T. ) ;
#48578=CARTESIAN_POINT ( 'NONE',  ( 9.838393222920561954, -78.31597548449377655, -4.482763737194812137 ) ) ;
#48583=CARTESIAN_POINT ( 'NONE',  ( -8.776032052582039000, -80.05126053055296609, 6.209312603182142176 ) ) ;
#48590=CARTESIAN_POINT ( 'NONE',  ( 8.109890173097999977, -76.21951620272498928, -7.078589237139000012 ) ) ;
#48598=CARTESIAN_POINT ( 'NONE',  ( 0.8024039916437721853, -80.96950772143027564, 10.72170357542168340 ) ) ;
#48603=CARTESIAN_POINT ( 'NONE',  ( -2.813789756862274949, -80.10416666666667140, -10.47020627418438998 ) ) ;
#48609=ADVANCED_FACE ( 'NONE', ( #1485 ), #55490, .F. ) ;
#48615=CARTESIAN_POINT ( 'NONE',  ( -10.75000000000000000, -79.00000000000000000, 0.000000000000000000 ) ) ;
#48619=CARTESIAN_POINT ( 'NONE',  ( -0.7814361956828775879, -79.98113340217017253, 10.72722109628113074 ) ) ;
#48631=ORIENTED_EDGE ( 'NONE', *, *, #3886, .F. ) ;
#48633=CARTESIAN_POINT ( 'NONE',  ( -10.11841891201000010, -77.71203272307600685, 6.752786780719000070 ) ) ;
#48635=CIRCLE ( 'NONE', #3487, 10.34999999999999964 ) ;
#48643=ORIENTED_EDGE ( 'NONE', *, *, #47982, .T. ) ;
#48644=CARTESIAN_POINT ( 'NONE',  ( -10.46898571549482249, -80.62085544309125851, -2.813567758576272393 ) ) ;
#48649=CARTESIAN_POINT ( 'NONE',  ( 9.779478297622604899, -80.64050622746258057, 5.481461471981479150 ) ) ;
#48650=CARTESIAN_POINT ( 'NONE',  ( 9.450487096927000508, -77.84733340637855292, -7.362360902975001231 ) ) ;
#48667=CARTESIAN_POINT ( 'NONE',  ( 10.63100742340999894, -77.23152976611999065, 5.913054471243999188 ) ) ;
#48669=CARTESIAN_POINT ( 'NONE',  ( -6.606377239730330864, -79.07291666666665719, -8.596418555780440229 ) ) ;
#48673=CARTESIAN_POINT ( 'NONE',  ( -4.297144572240187976, -79.50789134964543337, 9.855296198807199204 ) ) ;
#48674=VECTOR ( 'NONE', #2674, 1000.000000000000000 ) ;
#48676=CARTESIAN_POINT ( 'NONE',  ( 2.445294723173424334, -78.75875305519164726, 11.79638544041784876 ) ) ;
#48677=CARTESIAN_POINT ( 'NONE',  ( 11.88364051439999969, -79.52574899616899984, 2.560115967181999963 ) ) ;
#48693=EDGE_CURVE ( 'NONE', #12876, #21964, #40435, .T. ) ;
#48700=SURFACE_STYLE_USAGE ( .BOTH. , #7955 ) ;
#48705=CARTESIAN_POINT ( 'NONE',  ( 6.700289941238000146, -77.29597596972099893, -9.806486244952001385 ) ) ;
#48706=CARTESIAN_POINT ( 'NONE',  ( -10.68949850836979820, -78.61016907666331122, -1.353545228532917699 ) ) ;
#48709=VECTOR ( 'NONE', #36263, 1000.000000000000000 ) ;
#48715=CARTESIAN_POINT ( 'NONE',  ( 10.75916580683999690, -78.02281159953585643, 3.171507801093999657 ) ) ;
#48740=CARTESIAN_POINT ( 'NONE',  ( -9.964549960864999889, -77.45148636095500194, 6.650098383618000319 ) ) ;
#48752=CARTESIAN_POINT ( 'NONE',  ( -9.675565990256998816, -79.27387249041099437, 7.547703503149000070 ) ) ;
#48756=CARTESIAN_POINT ( 'NONE',  ( 11.93738031268999933, -76.74029815165599189, -2.836636764837000335 ) ) ;
#48761=CARTESIAN_POINT ( 'NONE',  ( -7.180765598437999664, -79.07253981239199447, 8.374863569145000852 ) ) ;
#48769=VECTOR ( 'NONE', #6291, 1000.000000000000000 ) ;
#48771=CARTESIAN_POINT ( 'NONE',  ( -10.88187945745999841, -78.86493240443898856, -5.690384754473000406 ) ) ;
#48784=CARTESIAN_POINT ( 'NONE',  ( 3.947457275559000500, -78.29525648518600178, -10.30140706531999939 ) ) ;
#48787=CARTESIAN_POINT ( 'NONE',  ( 6.766402264611000028, -79.37484760169999731, -8.946167390840999545 ) ) ;
#48800=CIRCLE ( 'NONE', #17696, 9.700000000000001066 ) ;
#48803=CARTESIAN_POINT ( 'NONE',  ( -1.760068246105999989, -79.96322189244729373, 11.95491093743999933 ) ) ;
#48808=EDGE_CURVE ( 'NONE', #3715, #31099, #12914, .T. ) ;
#48815=CARTESIAN_POINT ( 'NONE',  ( -3.647741209468000179, -77.22465764268899591, 10.65494948965999988 ) ) ;
#48817=CARTESIAN_POINT ( 'NONE',  ( 7.443430083705999678, -80.64091113825868717, 8.443285209763999433 ) ) ;
#48824=CARTESIAN_POINT ( 'NONE',  ( 0.2654799511899000319, -78.32520084447600084, -11.21373274707999990 ) ) ;
#48833=CARTESIAN_POINT ( 'NONE',  ( 6.355487164442999770, -78.10387449799000592, 9.297405415548999130 ) ) ;
#48840=CARTESIAN_POINT ( 'NONE',  ( -5.888313336375618157, -80.17893371189863672, -8.993908195848307585 ) ) ;
#48846=CARTESIAN_POINT ( 'NONE',  ( 10.56386067434198317, -78.73297245124483368, -2.300023321096129614 ) ) ;
#48849=ORIENTED_EDGE ( 'NONE', *, *, #44879, .T. ) ;
#48858=CARTESIAN_POINT ( 'NONE',  ( 9.789168614380999500, -78.78692200396399414, -4.831929617604999727 ) ) ;
#48859=CARTESIAN_POINT ( 'NONE',  ( -11.99999999994999911, -76.29999999994899440, 3.078392110872999642E-09 ) ) ;
#48876=DIRECTION ( 'NONE',  ( 0.000000000000000000, 1.000000000000000000, 0.000000000000000000 ) ) ;
#48885=CARTESIAN_POINT ( 'NONE',  ( -1.002682972311154996, -80.98253985172503633, 10.70322111416496469 ) ) ;
#48886=CARTESIAN_POINT ( 'NONE',  ( 11.14639666075000157, -81.14010679683600813, -1.632917082138999776 ) ) ;
#48900=EDGE_LOOP ( 'NONE', ( #758, #30164, #3516, #2889 ) ) ;
#48904=CARTESIAN_POINT ( 'NONE',  ( -7.374560639698973574, -78.97291666666667709, -9.596002108778167283 ) ) ;
#48907=CARTESIAN_POINT ( 'NONE',  ( 1.888467876749918561, -79.96132589731932683, 10.58272476696118147 ) ) ;
#48910=CARTESIAN_POINT ( 'NONE',  ( 7.661146283331804696, -77.28829716686190920, -7.541047385534751513 ) ) ;
#48917=B_SPLINE_CURVE_WITH_KNOTS ( 'NONE', 3,
 ( #54670, #5941, #9505, #55839, #5364, #23371, #19528, #680, #55539, #23946, #32788, #10682, #28663, #50836, #15389, #10381, #46124, #50249, #41962, #1535, #49964, #37521, #41382, #15090, #18663, #28075, #37818, #28366, #1830, #55247, #965, #18948, #41089, #46412, #14211, #46712, #19826, #36941, #42264, #36651, #54952, #51129, #33085, #6232, #45533, #14504, #5648, #27492, #32208, #5079, #24248, #37230, #14793, #23074, #9800, #19238, #27783, #32495, #50542, #10095, #23657, #41670, #1250, #2401, #33959 ),
 .UNSPECIFIED., .F., .F.,
 ( 4, 1, 1, 1, 1, 1, 1, 1, 1, 1, 1, 1, 1, 1, 1, 1, 1, 1, 1, 1, 1, 1, 1, 1, 1, 1, 1, 1, 1, 1, 1, 1, 1, 1, 1, 1, 1, 1, 1, 1, 1, 1, 1, 1, 1, 1, 1, 1, 1, 1, 1, 1, 1, 1, 1, 1, 1, 1, 1, 1, 1, 1, 4 ),
 ( 0.000000000000000000, 0.01249978245764908277, 0.02874978979738820883, 0.04499979713712733143, 0.06124980447686646096, 0.07749981181660559049, 0.09374981915634472696, 0.1099998264960838495, 0.1262498338358229721, 0.1424998411755621086, 0.1587498485153012451, 0.1749998558550403538, 0.1912498631947794903, 0.2074998705345185990, 0.2237498778742577632, 0.2399998852139968719, 0.2562498925537359806, 0.2724998998934751171, 0.2887499072332142536, 0.3049999145729533345, 0.3212499219126924710, 0.3374999292524316630, 0.3537499365921707439, 0.3699999439319098804, 0.3862499512716489614, 0.4024999586113881533, 0.4187499659511272898, 0.4349999732908663708, 0.4512499806306055072, 0.4674999879703446437, 0.4837499953100837802, 0.5000000026498229166, 0.5162500099895620531, 0.5325000173293011896, 0.5487500246690403261, 0.5650000320087793515, 0.5812500393485185990, 0.5975000466882577355, 0.6137500540279968719, 0.6300000613677360084, 0.6462500687074750338, 0.6625000760472141703, 0.6787500833869533068, 0.6950000907266924433, 0.7112500980664316907, 0.7275001054061708272, 0.7437501127459098527, 0.7600001200856489891, 0.7762501274253881256, 0.7925001347651272621, 0.8087501421048663985, 0.8250001494446054240, 0.8412501567843446715, 0.8575001641240838079, 0.8737501714638229444, 0.8900001788035620809, 0.9062501861433011063, 0.9225001934830402428, 0.9387502008227793793, 0.9550002081625185157, 0.9712502155022576522, 0.9875002228419967887, 1.000000000000000000 ),
 .UNSPECIFIED. ) ;
#48923=CARTESIAN_POINT ( 'NONE',  ( 6.043450171152322525, -76.56602488911100579, -10.48647902363864048 ) ) ;
#48946=CARTESIAN_POINT ( 'NONE',  ( -3.630949683904999947, -76.04999999999999716, 11.17491406647000041 ) ) ;
#48953=CARTESIAN_POINT ( 'NONE',  ( -7.506332976489000330, -77.59125689393900416, -7.926558599818001483 ) ) ;
#48954=CARTESIAN_POINT ( 'NONE',  ( -6.947761447124999989, -77.95055284899699188, -10.12543283296999874 ) ) ;
#48963=CARTESIAN_POINT ( 'NONE',  ( 4.180271402314000184, -79.53792282429900240, 11.29236839158000016 ) ) ;
#48965=DIRECTION ( 'NONE',  ( 0.000000000000000000, 0.7071067811866525998, -0.7071067811864425456 ) ) ;
#48967=CARTESIAN_POINT ( 'NONE',  ( -11.12496554189999998, -77.34408788795398948, -1.432917402686000097 ) ) ;
#48982=CARTESIAN_POINT ( 'NONE',  ( 0.000000000000000000, -87.29999999999999716, -9.599999999999999645 ) ) ;
#48991=CARTESIAN_POINT ( 'NONE',  ( 8.143754814233000516, -77.30963688248900212, -8.408463387949000278 ) ) ;
#48992=CARTESIAN_POINT ( 'NONE',  ( -10.45280047210375862, -78.61879557912125449, -2.510124479038314149 ) ) ;
#48999=CARTESIAN_POINT ( 'NONE',  ( -3.513443458491999571, -78.34964771555745244, -10.65240647004999808 ) ) ;
#49002=CARTESIAN_POINT ( 'NONE',  ( 4.653115705712000505, -79.06072274449400084, -10.20620521156999949 ) ) ;
#49020=CARTESIAN_POINT ( 'NONE',  ( 3.949587968339014044, -78.99812697311170950, 11.21690579045210967 ) ) ;
#49028=DIRECTION ( 'NONE',  ( -1.000000000000000000, 0.000000000000000000, 0.000000000000000000 ) ) ;
#49031=CARTESIAN_POINT ( 'NONE',  ( -8.852102014390000662, -78.01808746511700576, 8.004735621704000437 ) ) ;
#49046=CARTESIAN_POINT ( 'NONE',  ( 4.569396385344999700, -76.85349636657100802, 11.38719340697999982 ) ) ;
#49050=CARTESIAN_POINT ( 'NONE',  ( 10.41480047653000085, -78.36439489434398808, -3.637813056042999982 ) ) ;
#49057=EDGE_CURVE ( 'NONE', #45906, #26455, #55819, .T. ) ;
#49058=CARTESIAN_POINT ( 'NONE',  ( -9.108185712014998714, -78.26808746511700576, 8.236305738405000909 ) ) ;
#49064=EDGE_LOOP ( 'NONE', ( #23646, #21622, #13763, #3799 ) ) ;
#49074=CARTESIAN_POINT ( 'NONE',  ( 5.745747329289000227, -78.53052096864399800, 9.633509135241000720 ) ) ;
#49077=CIRCLE ( 'NONE', #22700, 10.74999999999999467 ) ;
#49092=CARTESIAN_POINT ( 'NONE',  ( -11.42485267055999998, -79.41066419345099803, 4.602037622659000071 ) ) ;
#49095=CARTESIAN_POINT ( 'NONE',  ( -2.114515350056125342, -77.99088766215147928, 10.53989743401121970 ) ) ;
#49096=CARTESIAN_POINT ( 'NONE',  ( -9.690626710582000314, -78.18390840682999965, -7.043281791253000357 ) ) ;
#49101=DIRECTION ( 'NONE',  ( -1.000000000000000000, 0.000000000000000000, 0.000000000000000000 ) ) ;
#49104=CARTESIAN_POINT ( 'NONE',  ( 5.172078487859000262, -77.66043913071798954, 10.00417756108999967 ) ) ;
#49105=CARTESIAN_POINT ( 'NONE',  ( 3.140974612311327796, -78.15416666666665435, 11.68767212001979594 ) ) ;
#49122=CARTESIAN_POINT ( 'NONE',  ( 1.639991984446999895, -77.91322009697699968, -11.14201017990999887 ) ) ;
#49128=CARTESIAN_POINT ( 'NONE',  ( 4.127591228001228352, -80.25644506522834831, -9.925940447433527325 ) ) ;
#49130=CARTESIAN_POINT ( 'NONE',  ( 2.179326186851605396, -78.70934838570477154, 11.00327889010784332 ) ) ;
#49131=DIRECTION ( 'NONE',  ( 0.000000000000000000, 1.000000000000000000, 7.697546304067999821E-14 ) ) ;
#49133=CARTESIAN_POINT ( 'NONE',  ( -0.2704138798119000153, -79.26806712638799013, 11.14367429999999892 ) ) ;
#49135=ORIENTED_EDGE ( 'NONE', *, *, #35821, .T. ) ;
#49136=ORIENTED_EDGE ( 'NONE', *, *, #50580, .T. ) ;
#49143=CIRCLE ( 'NONE', #8597, 11.59999999999999964 ) ;
#49146=CARTESIAN_POINT ( 'NONE',  ( 2.005614507304999794, -79.78068473043899189, -10.84800649278999884 ) ) ;
#49147=CARTESIAN_POINT ( 'NONE',  ( 1.570796326794909881, -76.43541666664329171, -11.99999999999999822 ) ) ;
#49151=CARTESIAN_POINT ( 'NONE',  ( 9.298505144763540287, -78.30746914334582698, -5.515131374144830012 ) ) ;
#49171=CARTESIAN_POINT ( 'NONE',  ( 3.228614917279000185, -81.04981373882509388, -10.79283437469000084 ) ) ;
#49176=LINE ( 'NONE', #17891, #13810 ) ;
#49177=ADVANCED_FACE ( 'NONE', ( #41538 ), #22950, .F. ) ;
#49197=CARTESIAN_POINT ( 'NONE',  ( -4.804849618107155607, -77.18816215842083750, -9.616802285769223246 ) ) ;
#49208=CARTESIAN_POINT ( 'NONE',  ( 8.321246128606000880, -78.37679717510499700, -8.715080868295999039 ) ) ;
#49210=B_SPLINE_CURVE_WITH_KNOTS ( 'NONE', 3,
 ( #38718, #25719, #39010, #42584, #57018, #16580, #16299, #20149, #34277, #37850, #29560, #30135, #55870 ),
 .UNSPECIFIED., .F., .F.,
 ( 4, 2, 2, 1, 2, 2, 4 ),
 ( 0.000000000000000000, 0.2499999999999995559, 0.3749999999999995559, 0.4374999999999995004, 0.4687499999999995004, 0.4999999999999994449, 1.000000000000000000 ),
 .UNSPECIFIED. ) ;
#49215=CARTESIAN_POINT ( 'NONE',  ( 3.141622339616611193, -76.54521521273609608, -11.68862050864443880 ) ) ;
#49218=VERTEX_POINT ( 'NONE', #1915 ) ;
#49245=EDGE_CURVE ( 'NONE', #50686, #15223, #36163, .T. ) ;
#49246=CARTESIAN_POINT ( 'NONE',  ( 8.899710312955001257, -77.72743860894800605, -6.322224476856000308 ) ) ;
#49247=CARTESIAN_POINT ( 'NONE',  ( 10.03503830778000072, -78.57452710374299443, -7.077696433220999950 ) ) ;
#49254=CARTESIAN_POINT ( 'NONE',  ( 7.165667693159000429, -78.94640101988399294, 9.347813962385000508 ) ) ;
#49255=CARTESIAN_POINT ( 'NONE',  ( 11.12875569142000032, -80.39817708664989482, 0.9871941560245000025 ) ) ;
#49258=CARTESIAN_POINT ( 'NONE',  ( -3.633103876188000125, -77.23514251594700397, 10.61219425078000000 ) ) ;
#49273=EDGE_CURVE ( 'NONE', #31098, #31041, #7902, .T. ) ;
#49279=ORIENTED_EDGE ( 'NONE', *, *, #26108, .F. ) ;
#49287=CARTESIAN_POINT ( 'NONE',  ( -9.858444951501001086, -76.63967465741301055, 7.443044607738000806 ) ) ;
#49288=CARTESIAN_POINT ( 'NONE',  ( -10.04959685401797032, -78.62904166612709389, -3.823887791762236699 ) ) ;
#49295=CARTESIAN_POINT ( 'NONE',  ( 5.263131812197999970, -77.91386622752847302, -9.905430536777000583 ) ) ;
#49298=CARTESIAN_POINT ( 'NONE',  ( 1.099819419251000019, -79.76886766254099825, 11.16281809564999961 ) ) ;
#49302=ORIENTED_EDGE ( 'NONE', *, *, #45383, .T. ) ;
#49309=CARTESIAN_POINT ( 'NONE',  ( 12.24159337356999977, -76.44530732801000283, -0.9828625608234000666 ) ) ;
#49314=LINE ( 'NONE', #21566, #36537 ) ;
#49315=CARTESIAN_POINT ( 'NONE',  ( -2.710423231297999891, -79.64442155979752158, 10.88447134676999895 ) ) ;
#49323=CARTESIAN_POINT ( 'NONE',  ( 10.46934363224000109, -77.28871046841200609, 5.823135730235999397 ) ) ;
#49324=CARTESIAN_POINT ( 'NONE',  ( 0.000000000000000000, -75.15999999999999659, 0.000000000000000000 ) ) ;
#49327=CARTESIAN_POINT ( 'NONE',  ( 0.9591162783412999771, -78.20799267308299818, -11.89603288543000126 ) ) ;
#49332=B_SPLINE_CURVE_WITH_KNOTS ( 'NONE', 3,
 ( #18914, #54919, #14472, #28921, #30065, #20085, #48116, #43673, #56955, #20369 ),
 .UNSPECIFIED., .F., .F.,
 ( 4, 2, 2, 2, 4 ),
 ( 0.000000000000000000, 0.1562500009478632601, 0.3125000018957265202, 0.4687500028435898081, 0.6250000037914531514 ),
 .UNSPECIFIED. ) ;
#49333=CARTESIAN_POINT ( 'NONE',  ( 1.070392484793000198, -79.89377542924650299, 10.86414404906000009 ) ) ;
#49335=EDGE_LOOP ( 'NONE', ( #42184, #16109, #13337 ) ) ;
#49336=AXIS2_PLACEMENT_3D ( 'NONE', #47482, #56319, #33277 ) ;
#49342=CARTESIAN_POINT ( 'NONE',  ( -7.844390712406000610, -76.37070918080398485, 9.586582683531000626 ) ) ;
#49344=CARTESIAN_POINT ( 'NONE',  ( -9.006387858036243088, -76.95327272276941244, 6.000451096308640153 ) ) ;
#49346=CARTESIAN_POINT ( 'NONE',  ( 2.047466772651000078, -79.91613885926460625, -11.07437783411999987 ) ) ;
#49352=CARTESIAN_POINT ( 'NONE',  ( 8.696932689530999738, -76.29999999999999716, 6.318691462144000681 ) ) ;
#49368=CARTESIAN_POINT ( 'NONE',  ( -9.053955183288000086, -76.62058518366599458, -6.099285168125999412 ) ) ;
#49374=CARTESIAN_POINT ( 'NONE',  ( -11.19989528650999944, -78.69393902665500207, 0.6168112860373000661 ) ) ;
#49381=DIRECTION ( 'NONE',  ( 0.000000000000000000, -1.000000000000000000, 0.000000000000000000 ) ) ;
#49386=B_SPLINE_CURVE_WITH_KNOTS ( 'NONE', 3,
 ( #51908, #33867, #55753, #46325 ),
 .UNSPECIFIED., .F., .F.,
 ( 4, 4 ),
 ( 0.000000000000000000, 1.000000000000000000 ),
 .UNSPECIFIED. ) ;
#49392=ORIENTED_EDGE ( 'NONE', *, *, #39337, .T. ) ;
#49393=CARTESIAN_POINT ( 'NONE',  ( 6.535144700214000402, -79.27162967006100303, 10.44020558090000073 ) ) ;
#49394=CARTESIAN_POINT ( 'NONE',  ( -10.15588082254999946, -76.17008402689499746, 5.382090387917999763 ) ) ;
#49395=CARTESIAN_POINT ( 'NONE',  ( -7.030156735645810784, -78.03177828160880836, 8.132844556063748342 ) ) ;
#49396=CARTESIAN_POINT ( 'NONE',  ( -10.86788298907000083, -77.73623996705498485, -5.040355520269000245 ) ) ;
#49402=CARTESIAN_POINT ( 'NONE',  ( 1.677588531244923464, -80.96289356016140459, 10.61806853404734419 ) ) ;
#49405=CARTESIAN_POINT ( 'NONE',  ( -9.992683672509999226, -78.35460208417299555, 4.939724043997999914 ) ) ;
#49406=CARTESIAN_POINT ( 'NONE',  ( 12.00000000000000000, -78.04999999999999716, 0.000000000000000000 ) ) ;
#49409=CARTESIAN_POINT ( 'NONE',  ( 3.042547531669000271, -78.24783470746899638, -10.31045122763999977 ) ) ;
#49414=CARTESIAN_POINT ( 'NONE',  ( 8.282307197233999219, -77.88941935644699299, -7.564489280985000619 ) ) ;
#49423=CARTESIAN_POINT ( 'NONE',  ( 4.249074618647000534, -76.86498468449899235, -10.30533674824999935 ) ) ;
#49429=CARTESIAN_POINT ( 'NONE',  ( -2.849102345952564619, -80.20408735378460108, -10.37120360196352209 ) ) ;
#49431=CARTESIAN_POINT ( 'NONE',  ( 6.879672600168782459, -79.17236621673578156, 8.859554948090913484 ) ) ;
#49434=ADVANCED_FACE ( 'NONE', ( #16054 ), #52076, .T. ) ;
#49436=CARTESIAN_POINT ( 'NONE',  ( 7.861046360898000351, -79.70384861441699798, 7.903072230637000040 ) ) ;
#49438=CARTESIAN_POINT ( 'NONE',  ( -10.75000000000000000, -79.59999999999999432, 0.000000000000000000 ) ) ;
#49450=CARTESIAN_POINT ( 'NONE',  ( 10.46019799182000121, -79.91686644544779483, 3.505129431450999977 ) ) ;
#49459=ORIENTED_EDGE ( 'NONE', *, *, #48133, .T. ) ;
#49461=DIRECTION ( 'NONE',  ( 0.000000000000000000, 1.000000000000000000, 0.000000000000000000 ) ) ;
#49465=CARTESIAN_POINT ( 'NONE',  ( 5.380788203752000065, -76.23673944062498720, 9.804131929786001010 ) ) ;
#49468=CARTESIAN_POINT ( 'NONE',  ( -1.394094229632999893, -76.41181109130799598, 10.79476414467999845 ) ) ;
#49470=CARTESIAN_POINT ( 'NONE',  ( 11.14639666075000157, -81.07231824355980621, -1.632917082138999776 ) ) ;
#49475=CARTESIAN_POINT ( 'NONE',  ( 10.70339364929999881, -81.17020448283959411, 2.537196166659999808 ) ) ;
#49500=CARTESIAN_POINT ( 'NONE',  ( -2.343696616972932745, -77.20767214764329367, -10.49131370137163621 ) ) ;
#49510=CARTESIAN_POINT ( 'NONE',  ( 6.891697027498000061, -78.79739778831900310, -9.743716654505998775 ) ) ;
#49519=VERTEX_POINT ( 'NONE', #37402 ) ;
#49525=CARTESIAN_POINT ( 'NONE',  ( -9.939389728518001732, -76.66042233052399979, 5.126617716248000001 ) ) ;
#49529=CARTESIAN_POINT ( 'NONE',  ( 7.919842512017161162, -77.46752299044597123, 8.988445846368001924 ) ) ;
#49550=CARTESIAN_POINT ( 'NONE',  ( -5.702669450565000631, -77.94532935296300025, 9.308862826782998923 ) ) ;
#49552=CARTESIAN_POINT ( 'NONE',  ( 4.023394881099000564, -78.22184600323399195, 11.60207191892000012 ) ) ;
#49557=ORIENTED_EDGE ( 'NONE', *, *, #2244, .T. ) ;
#49562=CARTESIAN_POINT ( 'NONE',  ( 7.508137979765999503, -79.88746266619089909, 7.790962400017000355 ) ) ;
#49565=CARTESIAN_POINT ( 'NONE',  ( 6.433795189870999742, -77.50750594596499354, -9.188274595716000803 ) ) ;
#49588=ORIENTED_EDGE ( 'NONE', *, *, #33929, .T. ) ;
#49589=CARTESIAN_POINT ( 'NONE',  ( 10.13128904261999885, -76.32605116317100169, -6.858865348462000355 ) ) ;
#49591=CARTESIAN_POINT ( 'NONE',  ( -8.547755989943867760, -78.65230355551688035, -6.557738066417508449 ) ) ;
#49598=CARTESIAN_POINT ( 'NONE',  ( 9.144378690012999300, -77.45084839649746300, -6.496033325431000094 ) ) ;
#49612=CARTESIAN_POINT ( 'NONE',  ( 10.16964605767000052, -76.40432458970499852, -6.884832982024000181 ) ) ;
#49623=CARTESIAN_POINT ( 'NONE',  ( -11.06076315227999984, -77.96694335400700027, 4.601693484369000053 ) ) ;
#49628=CARTESIAN_POINT ( 'NONE',  ( 6.585359383873000461, -79.70312102823399414, -8.706802385234000852 ) ) ;
#49634=CARTESIAN_POINT ( 'NONE',  ( -8.596418555780466875, -77.44791666666667140, 6.606377239730298001 ) ) ;
#49637=CARTESIAN_POINT ( 'NONE',  ( -2.533887857834999924, -76.98217140587999552, -12.24478563693999966 ) ) ;
#49642=CARTESIAN_POINT ( 'NONE',  ( -4.126717922116999837, -79.30368493481499570, -10.35494083817999922 ) ) ;
#49643=CARTESIAN_POINT ( 'NONE',  ( 12.00000000000000000, -77.14999999999999147, 0.000000000000000000 ) ) ;
#49649=CYLINDRICAL_SURFACE ( 'NONE', #29902, 10.75000000000000000 ) ;
#49663=CARTESIAN_POINT ( 'NONE',  ( -8.075725583014000009, -76.31079378115468614, -7.736700848914001227 ) ) ;
#49666=CARTESIAN_POINT ( 'NONE',  ( -11.03167625133000129, -77.64158425314199974, -0.06207630174703999970 ) ) ;
#49670=CARTESIAN_POINT ( 'NONE',  ( -9.805641529082999241, -79.30645443996699839, -5.446788484474000214 ) ) ;
#49671=CARTESIAN_POINT ( 'NONE',  ( 3.295987162183630748, -81.00000000000000000, 10.32795288958829616 ) ) ;
#49689=CARTESIAN_POINT ( 'NONE',  ( 2.837288914631000303, -79.51673028327599013, -12.10536388325999901 ) ) ;
#49690=CARTESIAN_POINT ( 'NONE',  ( 9.595281647244998879, -75.85997436215698997, 4.747863145975999899 ) ) ;
#49691=CARTESIAN_POINT ( 'NONE',  ( -6.826764225854004664, -78.02984463538199122, 8.304009225933823402 ) ) ;
#49692=CARTESIAN_POINT ( 'NONE',  ( -8.557169117579000783, -77.76336928247899039, -8.383968101560000719 ) ) ;
#49697=CARTESIAN_POINT ( 'NONE',  ( 2.199922411859213778, -80.95883067551849877, 10.53541604723973180 ) ) ;
#49700=CARTESIAN_POINT ( 'NONE',  ( 1.623230447552999944, -78.02776596815100163, -11.02813327291000078 ) ) ;
#49702=CARTESIAN_POINT ( 'NONE',  ( 0.6325562992502999915, -80.58843146505920174, -11.00758983218999987 ) ) ;
#49710=CARTESIAN_POINT ( 'NONE',  ( -6.884807209879999057, -78.33851671174899423, -8.855368954042999619 ) ) ;
#49715=CARTESIAN_POINT ( 'NONE',  ( -5.769945183727626770, -78.58007713321237020, -9.108383413252392202 ) ) ;
#49722=CARTESIAN_POINT ( 'NONE',  ( -11.05562587724999979, -77.21905714352298844, -1.423986317748999975 ) ) ;
#49729=CARTESIAN_POINT ( 'NONE',  ( 10.74987430283537471, -79.85617428146984764, 0.8320502212467579817 ) ) ;
#49733=CARTESIAN_POINT ( 'NONE',  ( 6.365665562422999635, -79.13050366622999832, 10.17242851768000023 ) ) ;
#49734=CARTESIAN_POINT ( 'NONE',  ( 3.609690327934000020, -80.23949669345269342, 10.39335624559999971 ) ) ;
#49738=B_SPLINE_CURVE_WITH_KNOTS ( 'NONE', 3,
 ( #48317, #6990, #21434, #39442, #34991, #47468, #20573, #52168, #47748, #30570, #48603, #43301, #26149, #57732, #53603, #27313, #44749, #493 ),
 .UNSPECIFIED., .F., .F.,
 ( 4, 2, 2, 2, 2, 2, 2, 2, 4 ),
 ( 0.000000000000000000, 0.1250000000000000000, 0.2499999999999999445, 0.3750000000000000000, 0.5000000000000000000, 0.6250000000000000000, 0.7500000000000000000, 0.8750000000000000000, 1.000000000000000000 ),
 .UNSPECIFIED. ) ;
#49739=CARTESIAN_POINT ( 'NONE',  ( -10.24999999991999999, -82.10000000007899246, 6.817355505960000646E-10 ) ) ;
#49753=ORIENTED_EDGE ( 'NONE', *, *, #20905, .T. ) ;
#49765=CARTESIAN_POINT ( 'NONE',  ( -1.408793263084000102, -76.34408402689498985, 10.90858184500000050 ) ) ;
#49766=CARTESIAN_POINT ( 'NONE',  ( 2.854661674668000058E-14, -82.00000000000000000, 0.000000000000000000 ) ) ;
#49768=CARTESIAN_POINT ( 'NONE',  ( 10.70339364929999881, -81.03462737628719026, 2.537196166659999808 ) ) ;
#49770=CARTESIAN_POINT ( 'NONE',  ( 11.90625000002000000, -76.20625000001498961, 3.701036097655999965E-09 ) ) ;
#49773=CARTESIAN_POINT ( 'NONE',  ( -11.09105850093000001, -80.38766464674519341, 1.974238845993000258 ) ) ;
#49782=CARTESIAN_POINT ( 'NONE',  ( -3.637215472919097969, -79.50258317002523256, 10.11602608574209761 ) ) ;
#49785=EDGE_LOOP ( 'NONE', ( #3042, #6678, #29951, #47078 ) ) ;
#49791=DIRECTION ( 'NONE',  ( -1.776356839400000238E-14, -1.000000000000000000, -4.588921835116999839E-14 ) ) ;
#49798=CARTESIAN_POINT ( 'NONE',  ( 0.002952034968893703631, -77.22510189820128801, -10.74995197471566222 ) ) ;
#49800=AXIS2_PLACEMENT_3D ( 'NONE', #17790, #49381, #43794 ) ;
#49803=CARTESIAN_POINT ( 'NONE',  ( 3.552363299575000077, -79.85053823319960031, -11.49294985030999960 ) ) ;
#49806=CARTESIAN_POINT ( 'NONE',  ( -6.817533650000999756, -78.26827991340999802, -9.935643240620999350 ) ) ;
#49818=CARTESIAN_POINT ( 'NONE',  ( -11.76761288928574345, -79.80000000000001137, -2.220697818543512003 ) ) ;
#49825=CARTESIAN_POINT ( 'NONE',  ( 11.79843486695000188, -77.38613504417455147, -2.076781258317999868 ) ) ;
#49833=CARTESIAN_POINT ( 'NONE',  ( 5.445437576845045591, -76.26093750000428884, 10.69085136092807709 ) ) ;
#49837=DIRECTION ( 'NONE',  ( -1.000000000000000000, 0.000000000000000000, 0.000000000000000000 ) ) ;
#49848=B_SPLINE_CURVE_WITH_KNOTS ( 'NONE', 3,
 ( #36050, #3882, #35155, #45515, #31309, #9488, #22474, #31901, #26893, #4767, #49943, #17170, #54367, #40485, #30732, #22768, #40185, #49352 ),
 .UNSPECIFIED., .F., .F.,
 ( 4, 2, 2, 2, 2, 2, 2, 2, 4 ),
 ( 0.000000000000000000, 0.1250000000000000000, 0.2500000000000000000, 0.3750000000000000000, 0.5000000000000000000, 0.6250000000000000000, 0.7500000000000000000, 0.8750000000000000000, 1.000000000000000000 ),
 .UNSPECIFIED. ) ;
#49856=CARTESIAN_POINT ( 'NONE',  ( 4.976417922892999890, -78.96415677378300302, 10.83839387946000166 ) ) ;
#49857=CARTESIAN_POINT ( 'NONE',  ( -11.05289869489000054, -80.57525882426229202, -0.2569212408223999766 ) ) ;
#49861=CARTESIAN_POINT ( 'NONE',  ( 6.201912463541000342, -78.57396040930800041, -9.171216270948999494 ) ) ;
#49864=LINE ( 'NONE', #45731, #48709 ) ;
#49885=CARTESIAN_POINT ( 'NONE',  ( -12.24569868602999989, -76.68065739571800066, 1.621947466804000149 ) ) ;
#49893=CARTESIAN_POINT ( 'NONE',  ( 12.00000000000000000, -79.04999999999999716, 0.000000000000000000 ) ) ;
#49906=CARTESIAN_POINT ( 'NONE',  ( -8.598496321198998871, -77.26496209410798599, -8.768570137950998600 ) ) ;
#49916=AXIS2_PLACEMENT_3D ( 'NONE', #40913, #23193, #13740 ) ;
#49920=CARTESIAN_POINT ( 'NONE',  ( -11.81636186152999990, -78.58780308901600620, -1.676035442350999993 ) ) ;
#49924=CARTESIAN_POINT ( 'NONE',  ( -10.42930648941000094, -80.00272080125370167, 3.225667704544000092 ) ) ;
#49937=CARTESIAN_POINT ( 'NONE',  ( 1.104250457816000175, -79.64377542924600561, 11.20779173096999948 ) ) ;
#49939=CARTESIAN_POINT ( 'NONE',  ( -6.606377239730371720, -79.92708333333332860, 8.596418555780411808 ) ) ;
#49943=CARTESIAN_POINT ( 'NONE',  ( -1.125737367536218558, -76.38333333333332575, 10.75000000000001066 ) ) ;
#49948=CARTESIAN_POINT ( 'NONE',  ( 6.606377239730313988, -78.32291666666665719, 8.596418555780454440 ) ) ;
#49953=CARTESIAN_POINT ( 'NONE',  ( 10.56375213976313532, -78.83523569680077969, -1.992565471537876887 ) ) ;
#49954=CARTESIAN_POINT ( 'NONE',  ( -9.596002108778193929, -79.74791666666662593, 7.374560639698935383 ) ) ;
#49957=CARTESIAN_POINT ( 'NONE',  ( -1.432420283025999996, -76.13522018723111273, 11.09153081809999897 ) ) ;
#49959=CARTESIAN_POINT ( 'NONE',  ( -10.87089293717000160, -76.56611249766200444, 0.9996073426339999735 ) ) ;
#49964=CARTESIAN_POINT ( 'NONE',  ( 7.483664081376597998, -78.37121083338536209, 9.354932563365712994 ) ) ;
#49965=CARTESIAN_POINT ( 'NONE',  ( 10.63562707217000103, -80.10962425429239886, 3.563914325689000240 ) ) ;
#49966=CARTESIAN_POINT ( 'NONE',  ( 6.715248240283044900, -81.00000000000001421, 8.571091062759663259 ) ) ;
#49967=ORIENTED_EDGE ( 'NONE', *, *, #30439, .F. ) ;
#49984=CARTESIAN_POINT ( 'NONE',  ( -2.526159795857000123, -79.54969871684099303, -12.05506223905000063 ) ) ;
#49985=CARTESIAN_POINT ( 'NONE',  ( 8.325915139015000577, -76.51939509872099165, 7.923884736887000457 ) ) ;
#49986=CARTESIAN_POINT ( 'NONE',  ( -7.655266710338128000, -78.03807782818779515, 7.547193342383588188 ) ) ;
#49987=CARTESIAN_POINT ( 'NONE',  ( 11.79843486695000010, -77.43781749739399345, -2.076781258317999868 ) ) ;
#49992=CARTESIAN_POINT ( 'NONE',  ( 4.887195288127127668, -80.93790857794486726, 9.583764635476553551 ) ) ;
#49995=CARTESIAN_POINT ( 'NONE',  ( -3.224264963920000504, -76.99278493408199608, -10.67046002915000003 ) ) ;
#49996=CARTESIAN_POINT ( 'NONE',  ( -3.140974612311405512, -78.19583333333332575, 11.68767212001977640 ) ) ;
#49997=CARTESIAN_POINT ( 'NONE',  ( -8.204091511170000572, -80.95026737670430350, -7.537247813386999340 ) ) ;
#50002=CARTESIAN_POINT ( 'NONE',  ( 5.263131812197999970, -77.86218301344499082, -9.905430536777000583 ) ) ;
#50012=CARTESIAN_POINT ( 'NONE',  ( 11.01685767354999967, -76.94669371350400411, -1.698071721886999841 ) ) ;
#50024=DIRECTION ( 'NONE',  ( 1.000000000000000000, 0.000000000000000000, 0.000000000000000000 ) ) ;
#50025=CARTESIAN_POINT ( 'NONE',  ( 10.83083824887000013, -79.62213958541198622, -2.635819302916999618 ) ) ;
#50031=ORIENTED_EDGE ( 'NONE', *, *, #24578, .F. ) ;
#50056=CARTESIAN_POINT ( 'NONE',  ( 5.365883907697000410, -80.03381055689840196, 9.905345355165000143 ) ) ;
#50063=CARTESIAN_POINT ( 'NONE',  ( -0.3187246912203000049, -80.77893456479243639, 11.26088853021000169 ) ) ;
#50072=B_SPLINE_CURVE_WITH_KNOTS ( 'NONE', 3,
 ( #32286, #37313, #32578, #28153, #5730, #31707, #13417, #31417, #36156, #54175, #10464, #55328, #28449, #14873, #51792, #20198, #46498, #24908 ),
 .UNSPECIFIED., .F., .F.,
 ( 4, 2, 2, 2, 2, 2, 2, 2, 4 ),
 ( 0.000000000000000000, 0.1250000000000000000, 0.2500000000000000000, 0.3750000000000000000, 0.5000000000000000000, 0.6250000000000000000, 0.7500000000000000000, 0.8750000000000000000, 1.000000000000000000 ),
 .UNSPECIFIED. ) ;
#50075=CARTESIAN_POINT ( 'NONE',  ( -8.944662455087330599, -79.55325894290034228, 5.962789625861153020 ) ) ;
#50090=CARTESIAN_POINT ( 'NONE',  ( 7.705636733279908057, -77.28876659844397068, -7.495763092362167868 ) ) ;
#50099=CARTESIAN_POINT ( 'NONE',  ( 2.945718361321999712, -78.97825989114500089, 11.40680644849000025 ) ) ;
#50113=CARTESIAN_POINT ( 'NONE',  ( 7.995633008690000487, -76.57771923186500374, 7.819446035993999899 ) ) ;
#50117=CARTESIAN_POINT ( 'NONE',  ( -10.11684109197000048, -76.35912155000400503, -4.871678881582000464 ) ) ;
#50119=CARTESIAN_POINT ( 'NONE',  ( 9.869603865684988264, -77.06050208244033684, -5.330340373397550735 ) ) ;
#50149=CARTESIAN_POINT ( 'NONE',  ( -4.367055522304000625, -79.98072316220059008, 10.15682858329000027 ) ) ;
#50150=LINE ( 'NONE', #9692, #26609 ) ;
#50152=CARTESIAN_POINT ( 'NONE',  ( 4.275724345439000373, -76.99001542893100236, -10.36997068233999997 ) ) ;
#50156=CARTESIAN_POINT ( 'NONE',  ( 8.775844806878042803, -79.80000000000001137, -7.911246177938791035 ) ) ;
#50157=CARTESIAN_POINT ( 'NONE',  ( 9.075965193531663644, -80.99999999999998579, -6.216670379854907225 ) ) ;
#50176=ADVANCED_FACE ( 'NONE', ( #18518 ), #27646, .F. ) ;
#50182=CARTESIAN_POINT ( 'NONE',  ( -6.659967121051000305, -76.82441250745586103, -9.025682433062998555 ) ) ;
#50197=CARTESIAN_POINT ( 'NONE',  ( -5.394429334091999984, -79.83507596080985991, -9.834543342166998769 ) ) ;
#50203=DIRECTION ( 'NONE',  ( 1.000000000000000000, 0.000000000000000000, 0.000000000000000000 ) ) ;
#50205=CARTESIAN_POINT ( 'NONE',  ( -3.103176923767000162, -78.11313629324600072, -11.64328410086999988 ) ) ;
#50208=CARTESIAN_POINT ( 'NONE',  ( 7.679819846117000637, -79.14513978978800424, -7.919728626202000576 ) ) ;
#50218=CARTESIAN_POINT ( 'NONE',  ( 10.40130232906999908, -76.07658568656098907, -6.940236885917999032 ) ) ;
#50222=ORIENTED_EDGE ( 'NONE', *, *, #37091, .T. ) ;
#50224=CARTESIAN_POINT ( 'NONE',  ( -5.236138783747000147, -78.62277635977000045, 9.840602177168999987 ) ) ;
#50226=CARTESIAN_POINT ( 'NONE',  ( -10.41906440735603390, -79.58915406351319177, -5.613747789635666230 ) ) ;
#50241=CARTESIAN_POINT ( 'NONE',  ( 7.628372981931305752, -78.78778873427579299, -7.574329845077384604 ) ) ;
#50245=CARTESIAN_POINT ( 'NONE',  ( 4.903943924252999409, -76.41112154911152743, -10.05113017056000047 ) ) ;
#50248=CARTESIAN_POINT ( 'NONE',  ( -5.197406821774317009, -76.13935780419708976, -11.03714881444417806 ) ) ;
#50249=CARTESIAN_POINT ( 'NONE',  ( -4.085715681792862597, -78.45259877965739292, 11.26174581117867390 ) ) ;
#50251=CARTESIAN_POINT ( 'NONE',  ( 11.14115696400000033, -79.00685466694699244, -1.301050381412999890 ) ) ;
#50262=CYLINDRICAL_SURFACE ( 'NONE', #46430, 9.599999999999999645 ) ;
#50263=CARTESIAN_POINT ( 'NONE',  ( -9.393203674808288994, -80.95833333333331439, 5.413904038987134015 ) ) ;
#50272=CARTESIAN_POINT ( 'NONE',  ( 12.42775431196000113, -79.62100617581799611, -0.3754309351819000162 ) ) ;
#50273=CARTESIAN_POINT ( 'NONE',  ( 7.200008815102000526, -76.32067638237299434, -8.806490984069000660 ) ) ;
#50274=CARTESIAN_POINT ( 'NONE',  ( 9.600846333656411602, -77.88729592899156273, 4.835758510686050116 ) ) ;
#50275=CARTESIAN_POINT ( 'NONE',  ( 11.95248949435000085, -78.88927060784799039, 0.8087524912306001124 ) ) ;
#50282=CARTESIAN_POINT ( 'NONE',  ( -3.610459473067000324, -77.29238470710198783, 10.54605058607999979 ) ) ;
#50283=CARTESIAN_POINT ( 'NONE',  ( 8.135116633385999663, -76.96737925144761050, 9.200136113044999675 ) ) ;
#50284=CARTESIAN_POINT ( 'NONE',  ( -10.71095089696999914, -80.41331365663170061, -3.064757027600999884 ) ) ;
#50288=CARTESIAN_POINT ( 'NONE',  ( 11.08595418830999968, -76.93614735138400818, -1.708721840212999998 ) ) ;
#50298=EDGE_CURVE ( 'NONE', #22076, #12876, #4935, .T. ) ;
#50302=CARTESIAN_POINT ( 'NONE',  ( -4.550163292746999488, -77.36849323694099212, -10.30194052436999996 ) ) ;
#50308=CARTESIAN_POINT ( 'NONE',  ( -7.202660771834071163, -80.16699785840980041, -7.981660149312156172 ) ) ;
#50312=CIRCLE ( 'NONE', #36967, 9.700000000000001066 ) ;
#50315=CARTESIAN_POINT ( 'NONE',  ( -8.926133614190998600, -79.84003032942598566, 6.676731181684000482 ) ) ;
#50326=CARTESIAN_POINT ( 'NONE',  ( -9.393203674808267678, -78.04166666666665719, -5.413904038987171319 ) ) ;
#50344=CARTESIAN_POINT ( 'NONE',  ( -6.474781754604000739, -80.34238059820370381, -9.218806710208998112 ) ) ;
#50362=CARTESIAN_POINT ( 'NONE',  ( -6.382001649558278089, -79.52561732951967599, 8.650654035762535443 ) ) ;
#50380=CARTESIAN_POINT ( 'NONE',  ( -5.993167237703258543, -77.17810086631732247, -8.925825369205432125 ) ) ;
#50385=CARTESIAN_POINT ( 'NONE',  ( 11.43764105185000091, -79.97007275658970116, 2.691257544168000226 ) ) ;
#50388=DIRECTION ( 'NONE',  ( -1.000000000000000000, 0.000000000000000000, 0.000000000000000000 ) ) ;
#50390=CARTESIAN_POINT ( 'NONE',  ( -8.607099856842999941, -77.75282292035799969, -8.432888219828999610 ) ) ;
#50402=CARTESIAN_POINT ( 'NONE',  ( -11.78092668186225644, -79.79999999999998295, -2.153435279904234889 ) ) ;
#50404=CARTESIAN_POINT ( 'NONE',  ( -10.07624512687999996, -76.30181786998500115, -4.852130239470000106 ) ) ;
#50408=CARTESIAN_POINT ( 'NONE',  ( 11.11267589788999999, -76.58485902790600619, 1.610019623660999821 ) ) ;
#50417=CARTESIAN_POINT ( 'NONE',  ( 1.407171709420440342, -79.63541666666665719, -10.74999999999999822 ) ) ;
#50418=LINE ( 'NONE', #41254, #28289 ) ;
#50419=CARTESIAN_POINT ( 'NONE',  ( 11.05000000000000071, -76.00000000000000000, 0.000000000000000000 ) ) ;
#50438=CARTESIAN_POINT ( 'NONE',  ( 10.51638713295000116, -81.05822150553019867, 4.415123262547999694 ) ) ;
#50441=CARTESIAN_POINT ( 'NONE',  ( -10.96060824219999930, -77.38464009822899925, 2.383941600041999731 ) ) ;
#50458=CARTESIAN_POINT ( 'NONE',  ( 3.330893700617000075, -78.97344966613400175, -11.81951464247000061 ) ) ;
#50474=CARTESIAN_POINT ( 'NONE',  ( 10.48543666025110710, -79.00833333333332575, -6.043427764450776785 ) ) ;
#50478=ORIENTED_EDGE ( 'NONE', *, *, #58241, .F. ) ;
#50486=CARTESIAN_POINT ( 'NONE',  ( -10.85634995915000012, -76.17260508320899248, -5.741293403527000017 ) ) ;
#50498=CARTESIAN_POINT ( 'NONE',  ( 11.77424395174999994, -78.27591218578899657, 2.561825723684000078 ) ) ;
#50501=CARTESIAN_POINT ( 'NONE',  ( 5.768362037549999322, -78.62764927275399884, -9.403610972502001175 ) ) ;
#50505=CARTESIAN_POINT ( 'NONE',  ( 10.75000000000000000, -79.25000000000000000, 0.000000000000000000 ) ) ;
#50506=CARTESIAN_POINT ( 'NONE',  ( 2.241317775079999741, -79.89861982803429896, -11.94785552921999994 ) ) ;
#50516=CARTESIAN_POINT ( 'NONE',  ( -9.744524944696001612, -79.24921224881200033, -5.412839751281999234 ) ) ;
#50533=CARTESIAN_POINT ( 'NONE',  ( 6.286256452161005370, -78.77486376296185711, -8.720713732654903794 ) ) ;
#50540=CARTESIAN_POINT ( 'NONE',  ( -7.725782153457552148, -76.47895244894142763, 9.441631877404960349 ) ) ;
#50542=CARTESIAN_POINT ( 'NONE',  ( 10.46948686332650169, -77.34029684728238863, 5.823215396550667222 ) ) ;
#50543=CARTESIAN_POINT ( 'NONE',  ( -10.39759693597000023, -79.86449716727609882, -4.208097972746998927 ) ) ;
#50552=CARTESIAN_POINT ( 'NONE',  ( 12.00000000000000000, -77.64999999999999147, 0.000000000000000000 ) ) ;
#50562=CARTESIAN_POINT ( 'NONE',  ( 11.35264079262999992, -76.54345827915599898, 2.443064948458000263 ) ) ;
#50563=CARTESIAN_POINT ( 'NONE',  ( 4.601699413956535700, -77.93997073655324925, 9.715216775470373989 ) ) ;
#50564=CARTESIAN_POINT ( 'NONE',  ( 10.42503750987000011, -77.34289962869399915, -5.902083371034000159 ) ) ;
#50569=CARTESIAN_POINT ( 'NONE',  ( 4.107670404649118368, -80.94402357793687486, 9.934114837241841300 ) ) ;
#50572=CARTESIAN_POINT ( 'NONE',  ( -5.822924921437000023, -77.80987522413700219, 9.505164171658000427 ) ) ;
#50573=CARTESIAN_POINT ( 'NONE',  ( -4.368496844144680757, -76.05524822590969336, 10.93374668194784860 ) ) ;
#50574=CARTESIAN_POINT ( 'NONE',  ( -3.181350147293000141, -80.78918126068253969, 10.67690104642000115 ) ) ;
#50575=EDGE_LOOP ( 'NONE', ( #54080, #49302, #52425, #51189 ) ) ;
#50580=EDGE_CURVE ( 'NONE', #15223, #23344, #37845, .T. ) ;
#50581=CARTESIAN_POINT ( 'NONE',  ( -5.751434148371999733, -77.78047398443999327, -9.630115047516998317 ) ) ;
#50594=EDGE_CURVE ( 'NONE', #21904, #19797, #6445, .T. ) ;
#50599=CARTESIAN_POINT ( 'NONE',  ( 6.043427764450761686, -77.63333333333329733, 10.48543666025110888 ) ) ;
#50608=CARTESIAN_POINT ( 'NONE',  ( 8.413030999918001740, -80.15288448085529183, -7.136010437995999212 ) ) ;
#50610=ORIENTED_EDGE ( 'NONE', *, *, #40953, .T. ) ;
#50625=CARTESIAN_POINT ( 'NONE',  ( 6.536064251314178897, -80.02434017810877265, 8.743451022905414760 ) ) ;
#50634=EDGE_CURVE ( 'NONE', #41515, #22103, #41599, .T. ) ;
#50641=CARTESIAN_POINT ( 'NONE',  ( -11.26045488449999965, -80.76374820225451856, 0.3336940576009999604 ) ) ;
#50657=CARTESIAN_POINT ( 'NONE',  ( -2.439418945719407983, -79.49321589760896245, 10.46964760755776247 ) ) ;
#50667=EDGE_CURVE ( 'NONE', #25175, #7399, #49143, .T. ) ;
#50674=CARTESIAN_POINT ( 'NONE',  ( -6.167996266013765272, -77.17653180539056734, -8.804416017395640282 ) ) ;
#50676=ORIENTED_EDGE ( 'NONE', *, *, #46991, .T. ) ;
#50678=CARTESIAN_POINT ( 'NONE',  ( 11.43764105185000091, -79.90228420331349923, 2.691257544168000226 ) ) ;
#50683=CARTESIAN_POINT ( 'NONE',  ( -1.355082891136000001, -77.73935448679299043, -11.85745557885999979 ) ) ;
#50684=AXIS2_PLACEMENT_3D ( 'NONE', #47389, #33482, #6633 ) ;
#50686=VERTEX_POINT ( 'NONE', #35593 ) ;
#50696=CARTESIAN_POINT ( 'NONE',  ( 0.000000000000000000, -87.59999999999999432, -9.599999999999999645 ) ) ;
#50700=CARTESIAN_POINT ( 'NONE',  ( 10.97835188747000146, -75.93304601283999489, -2.133021021907000048 ) ) ;
#50701=B_SPLINE_CURVE_WITH_KNOTS ( 'NONE', 3,
 ( #17022, #44764, #22019, #40330, #21157, #53039, #39738, #13455, #48332, #31451, #4013, #30868, #48904, #40027, #58040, #53321, #17600, #34719 ),
 .UNSPECIFIED., .F., .F.,
 ( 4, 2, 2, 2, 2, 2, 2, 2, 4 ),
 ( 0.000000000000000000, 0.1250000000000000000, 0.2500000000000000000, 0.3750000000000000000, 0.5000000000000000000, 0.6250000000000000000, 0.7500000000000000000, 0.8750000000000000000, 1.000000000000000000 ),
 .UNSPECIFIED. ) ;
#50714=DIRECTION ( 'NONE',  ( 0.000000000000000000, -1.000000000000000000, 0.000000000000000000 ) ) ;
#50735=CARTESIAN_POINT ( 'NONE',  ( 6.471694488619999852, -80.60357658748300480, 9.391741773560999818 ) ) ;
#50738=CARTESIAN_POINT ( 'NONE',  ( -10.86658628928999981, -76.92162226719798923, -2.781249891074999869 ) ) ;
#50743=CARTESIAN_POINT ( 'NONE',  ( 11.00000000000000000, -81.00000000000000000, -2.369510767747999942E-13 ) ) ;
#50745=CARTESIAN_POINT ( 'NONE',  ( -10.75000000000000000, -78.50000000000000000, 0.000000000000000000 ) ) ;
#50746=CARTESIAN_POINT ( 'NONE',  ( 3.862060628231000159, -80.54547121896008832, 10.58270681924999934 ) ) ;
#50752=CARTESIAN_POINT ( 'NONE',  ( 8.905881360917000222, -79.06849849426399146, 8.286615985300000986 ) ) ;
#50760=EDGE_CURVE ( 'NONE', #20196, #42760, #37938, .T. ) ;
#50770=CARTESIAN_POINT ( 'NONE',  ( -10.15788331741117645, -76.62184280497177724, 3.765280591527957910 ) ) ;
#50781=CARTESIAN_POINT ( 'NONE',  ( -0.6669403506045999963, -76.18678200654200339, -12.26286337364000012 ) ) ;
#50782=DIRECTION ( 'NONE',  ( 0.000000000000000000, 1.000000000000000000, 0.000000000000000000 ) ) ;
#50793=CARTESIAN_POINT ( 'NONE',  ( 4.358044849164000922, -77.23133731782699840, -11.11047130621000001 ) ) ;
#50797=CARTESIAN_POINT ( 'NONE',  ( -8.065049863481000614, -78.96773976718499455, 7.357332172019000360 ) ) ;
#50805=CARTESIAN_POINT ( 'NONE',  ( -6.043427764450833628, -77.81666666666667709, 10.48543666025107335 ) ) ;
#50809=ORIENTED_EDGE ( 'NONE', *, *, #33229, .T. ) ;
#50812=CARTESIAN_POINT ( 'NONE',  ( -11.52726388849324657, -79.53165972776588433, 2.674423737329086670 ) ) ;
#50817=CARTESIAN_POINT ( 'NONE',  ( -0.2721136687859672665, -79.22683890273980012, 11.21372209014444898 ) ) ;
#50826=CARTESIAN_POINT ( 'NONE',  ( 5.979471860834143726, -78.77211117144966579, -8.933429240604114696 ) ) ;
#50828=ORIENTED_EDGE ( 'NONE', *, *, #14350, .F. ) ;
#50834=CARTESIAN_POINT ( 'NONE',  ( 5.936735104356777981, -76.21482328080708157, -10.65773319741336067 ) ) ;
#50836=CARTESIAN_POINT ( 'NONE',  ( -11.86126082642098112, -78.56111604135236348, -1.682403921698609306 ) ) ;
#50844=FACE_OUTER_BOUND ( 'NONE', #30379, .T. ) ;
#50845=CONICAL_SURFACE ( 'NONE', #58369, 10.90000000000000036, 0.7853981633972997312 ) ;
#50858=CARTESIAN_POINT ( 'NONE',  ( -4.650415628119000111, -76.36880274324299478, -10.64070859955000081 ) ) ;
#50859=CARTESIAN_POINT ( 'NONE',  ( 9.692338806031742138, -77.88577333623729260, 4.653132537965349869 ) ) ;
#50860=CARTESIAN_POINT ( 'NONE',  ( 3.925078296951999501, -78.41454232321599704, 11.31856107452000160 ) ) ;
#50861=DIRECTION ( 'NONE',  ( 0.000000000000000000, -1.000000000000000000, 0.000000000000000000 ) ) ;
#50862=CARTESIAN_POINT ( 'NONE',  ( 2.813943391462377264, -78.95432111614685766, 10.47071761770257758 ) ) ;
#50864=CARTESIAN_POINT ( 'NONE',  ( 9.099057355994125018, -80.89508958227955304, 5.728627856209059566 ) ) ;
#50867=CARTESIAN_POINT ( 'NONE',  ( 1.606468910658999993, -78.09549303256399355, -10.91425636589999826 ) ) ;
#50868=CARTESIAN_POINT ( 'NONE',  ( -10.51110168223000052, -76.10674174704419670, 6.351495789100000344 ) ) ;
#50869=CARTESIAN_POINT ( 'NONE',  ( -9.092652447878998956, -80.44016134263529239, -6.437458829046000197 ) ) ;
#50872=CARTESIAN_POINT ( 'NONE',  ( 6.557611461288021637, -80.42306247819995235, 8.547703452968136162 ) ) ;
#50874=CARTESIAN_POINT ( 'NONE',  ( -10.17713110909000029, -76.73157247464199315, 4.716330562529999604 ) ) ;
#50880=CARTESIAN_POINT ( 'NONE',  ( -10.75000000000000000, -78.50615977947786917, -0.8321152720825113480 ) ) ;
#50885=CARTESIAN_POINT ( 'NONE',  ( -6.686799317902000439, -76.85100271990599197, -9.062045808939998892 ) ) ;
#50888=CARTESIAN_POINT ( 'NONE',  ( -12.00000000000000000, -77.79999999999999716, 0.000000000000000000 ) ) ;
#50897=CARTESIAN_POINT ( 'NONE',  ( 10.97276992925000094, -79.71710299282599976, 1.140199307644999882 ) ) ;
#50902=ORIENTED_EDGE ( 'NONE', *, *, #17045, .T. ) ;
#50910=CARTESIAN_POINT ( 'NONE',  ( 1.407171709420440342, -78.13541666666665719, -10.74999999999999822 ) ) ;
#50913=ORIENTED_EDGE ( 'NONE', *, *, #44777, .T. ) ;
#50921=CARTESIAN_POINT ( 'NONE',  ( -11.68767212001980127, -76.87916666666666288, 3.140974612311317138 ) ) ;
#50930=CARTESIAN_POINT ( 'NONE',  ( -9.662176860537863732, -76.63657409603162307, -4.763807680900224106 ) ) ;
#50935=CARTESIAN_POINT ( 'NONE',  ( 12.00000000000000000, -78.16041666666669130, 1.570796326794922093 ) ) ;
#50946=CARTESIAN_POINT ( 'NONE',  ( 10.74992915973507479, -79.35045861777548737, 0.04600403722853010913 ) ) ;
#50954=DIRECTION ( 'NONE',  ( 0.000000000000000000, 1.000000000000000000, 0.000000000000000000 ) ) ;
#50959=CARTESIAN_POINT ( 'NONE',  ( -3.630949683904999947, -76.04999999999999716, 11.17491406647000041 ) ) ;
#50963=CARTESIAN_POINT ( 'NONE',  ( 4.847151869481000297, -79.04368020031598974, 11.00961342987999991 ) ) ;
#50967=CARTESIAN_POINT ( 'NONE',  ( -3.532272164985999829, -77.52231996340199771, 11.39993665757999963 ) ) ;
#50969=B_SPLINE_SURFACE_WITH_KNOTS ( 'NONE', 3, 3, ( 
 ( #43509, #21064, #57079, #16643, #58239, #23392, #40527, #18972, #10116, #32518, #27514, #45261, #27222, #45852, #23100, #36094, #41110, #9236, #49690 ),
 ( #41404, #412, #53819, #701, #40820, #13945, #18098, #32231, #50273, #40227, #13652, #4809, #35788, #18683, #22809, #9821, #54111, #13355, #36963 ),
 ( #31647, #31353, #36675, #26930, #121, #49985, #31941, #17802, #18390, #36381, #54407, #9529, #14233, #49394, #45555, #5101, #54691, #44961, #28096 ),
 ( #46145, #27805, #987, #54976, #14525, #5670, #50562, #8943, #4516, #22517, #50858, #55860, #28682, #51150, #24268, #41693, #10705, #38128, #46734 ) ),
 .UNSPECIFIED., .F., .F., .F.,
 ( 4, 4 ),
 ( 4, 1, 1, 1, 1, 1, 1, 1, 1, 1, 1, 1, 1, 1, 1, 1, 4 ),
 ( -0.1772706441294000235, 1.177270644128999955 ),
 ( -0.008015739112864999488, 0.01803541300395000019, 0.04408656512076000039, 0.07013771723757000753, 0.09618886935437999386, 0.1222400214711999999, 0.1482911735880000081, 0.1743423257047999886, 0.2003934778215999968, 0.2264446299384000050, 0.2524957820552999888, 0.2785469341721000247, 0.3045980862889000051, 0.3306492384056999856, 0.3567003905224999660, 0.3827515426393000020, 0.4088026947561000379 ),
 .UNSPECIFIED. ) ;
#50971=CIRCLE ( 'NONE', #33952, 10.34999999999999964 ) ;
#50972=CARTESIAN_POINT ( 'NONE',  ( -10.75000000000000000, -79.00000000000000000, 0.000000000000000000 ) ) ;
#50982=DIRECTION ( 'NONE',  ( 0.000000000000000000, 1.000000000000000000, 0.000000000000000000 ) ) ;
#50984=CARTESIAN_POINT ( 'NONE',  ( -0.6606141896019371851, -79.80000000000001137, -11.78048067788835773 ) ) ;
#50985=CARTESIAN_POINT ( 'NONE',  ( -10.63937949802054383, -80.08894649173862490, 1.537974160709378202 ) ) ;
#50988=CARTESIAN_POINT ( 'NONE',  ( 10.97835188747000146, -76.00083456611598365, -2.133021021907000048 ) ) ;
#50989=CARTESIAN_POINT ( 'NONE',  ( -5.237477409016258356, -76.51604757055756068, 9.510330503777982614 ) ) ;
#51007=CARTESIAN_POINT ( 'NONE',  ( -7.374560639699019760, -79.32708333333330586, 9.596002108778129980 ) ) ;
#51014=DIRECTION ( 'NONE',  ( -1.776356839400000238E-14, -1.000000000000000000, -1.184237892933000067E-14 ) ) ;
#51015=VECTOR ( 'NONE', #32071, 1000.000000000000000 ) ;
#51016=CARTESIAN_POINT ( 'NONE',  ( 12.27743704900000132, -77.62500106391100019, 0.2455986337158999888 ) ) ;
#51023=CARTESIAN_POINT ( 'NONE',  ( -1.111829811609999830, -80.32601340704829340, -11.23414193798999960 ) ) ;
#51026=CARTESIAN_POINT ( 'NONE',  ( 11.19952915612999966, -78.14725770227899204, -0.6234238306063999424 ) ) ;
#51031=CARTESIAN_POINT ( 'NONE',  ( 9.966176356049450291, -81.00000000000000000, -4.720956196838709928 ) ) ;
#51035=CARTESIAN_POINT ( 'NONE',  ( 5.620590082324000036, -80.36488510293838772, -9.763102121971000358 ) ) ;
#51044=CARTESIAN_POINT ( 'NONE',  ( -7.733454931756999606, -78.68868807833099766, 9.390218602554998739 ) ) ;
#51047=VERTEX_POINT ( 'NONE', #57330 ) ;
#51048=ORIENTED_EDGE ( 'NONE', *, *, #38593, .T. ) ;
#51057=CARTESIAN_POINT ( 'NONE',  ( 2.787247272279751886, -80.74587480725163857, -10.40638828497226953 ) ) ;
#51074=CARTESIAN_POINT ( 'NONE',  ( 6.725657209017000149, -77.23867228970199506, -9.843613558058999402 ) ) ;
#51078=CARTESIAN_POINT ( 'NONE',  ( -5.268979267983999293, -78.66391321173168194, 9.902321347348999936 ) ) ;
#51085=CARTESIAN_POINT ( 'NONE',  ( -6.817533650000999756, -78.08600697782200939, -9.935643240620999350 ) ) ;
#51103=CARTESIAN_POINT ( 'NONE',  ( 8.696932689530999738, -76.29999999999999716, 6.318691462144000681 ) ) ;
#51106=CARTESIAN_POINT ( 'NONE',  ( -10.99991520232270936, -76.33543575793046898, 2.019904293929638772 ) ) ;
#51107=CARTESIAN_POINT ( 'NONE',  ( 10.47020627418438643, -79.77083333333332860, 2.813789756862283387 ) ) ;
#51111=CARTESIAN_POINT ( 'NONE',  ( -11.06509191825306004, -79.36302061774877359, -1.839932010799510964 ) ) ;
#51115=CARTESIAN_POINT ( 'NONE',  ( 8.696932689530999738, -76.29999999999999716, 6.318691462144000681 ) ) ;
#51122=CARTESIAN_POINT ( 'NONE',  ( 7.815245125686015371, -78.78981169969108578, -7.382265784365210415 ) ) ;
#51128=CARTESIAN_POINT ( 'NONE',  ( -1.127572418632452944, -76.93174530860108007, 12.14745662550945760 ) ) ;
#51129=CARTESIAN_POINT ( 'NONE',  ( 11.97758669317381930, -77.80149520948634745, 0.2396004080751424348 ) ) ;
#51130=CARTESIAN_POINT ( 'NONE',  ( 5.865103843792000227, -78.50268001718499988, -9.561319920857000554 ) ) ;
#51137=CARTESIAN_POINT ( 'NONE',  ( 1.508441505249127790, -77.71417431448334412, 11.11513442064821966 ) ) ;
#51150=CARTESIAN_POINT ( 'NONE',  ( -10.26075081888999918, -76.23781109130798939, 5.437666049857999617 ) ) ;
#51151=CARTESIAN_POINT ( 'NONE',  ( 9.337418898828111935, -77.89153506836979091, 5.340059034472213639 ) ) ;
#51152=CARTESIAN_POINT ( 'NONE',  ( -11.48784787867999846, -78.08899053812999114, -3.397854551190000016 ) ) ;
#51156=CARTESIAN_POINT ( 'NONE',  ( 10.28406176041941755, -80.87383273565515651, 3.134224279283850390 ) ) ;
#51160=CARTESIAN_POINT ( 'NONE',  ( 5.066356038949999530, -77.79589325954400181, 9.799682181994000985 ) ) ;
#51161=CARTESIAN_POINT ( 'NONE',  ( 12.07535958108000074, -76.88541377483805661, -2.237927141218000404 ) ) ;
#51162=CARTESIAN_POINT ( 'NONE',  ( -10.48543666025109111, -78.34166666666665435, -6.043427764450793660 ) ) ;
#51168=CARTESIAN_POINT ( 'NONE',  ( -2.309466437479000156, -77.65760813670300422, 10.97654204954999990 ) ) ;
#51172=CARTESIAN_POINT ( 'NONE',  ( 7.929877441717000153, -77.26081807572799676, -8.610461240849000220 ) ) ;
#51178=CARTESIAN_POINT ( 'NONE',  ( -7.012165219465999577, -77.20507517892998806, 8.812689912465000219 ) ) ;
#51180=DIRECTION ( 'NONE',  ( 0.000000000000000000, 1.000000000000000000, 0.000000000000000000 ) ) ;
#51189=ORIENTED_EDGE ( 'NONE', *, *, #44879, .F. ) ;
#51192=CARTESIAN_POINT ( 'NONE',  ( 2.368087569675000115, -80.31630253886619641, 10.55620284977000090 ) ) ;
#51194=VERTEX_POINT ( 'NONE', #45740 ) ;
#51205=CARTESIAN_POINT ( 'NONE',  ( 11.68767212001979594, -76.52916666666243373, -3.140974612311341563 ) ) ;
#51217=CARTESIAN_POINT ( 'NONE',  ( -6.043427764450833628, -76.81666666666666288, 10.48543666025107335 ) ) ;
#51229=CARTESIAN_POINT ( 'NONE',  ( -12.00000000000000000, -78.39999999999999147, 0.000000000000000000 ) ) ;
#51231=CARTESIAN_POINT ( 'NONE',  ( -6.912545260079999920, -78.39582039176799810, -8.891046157644998615 ) ) ;
#51240=CARTESIAN_POINT ( 'NONE',  ( 9.448045098518800700, -79.38977526190863898, 5.154015187206609561 ) ) ;
#51255=CARTESIAN_POINT ( 'NONE',  ( 6.263868601946986914, -80.27490189587713587, -8.736624837916803443 ) ) ;
#51260=CARTESIAN_POINT ( 'NONE',  ( 3.714552462503000196, -79.48391337144799706, 11.44155784250999908 ) ) ;
#51261=DIRECTION ( 'NONE',  ( 0.000000000000000000, 1.000000000000000000, 0.000000000000000000 ) ) ;
#51265=CARTESIAN_POINT ( 'NONE',  ( -8.524893907337000698, -77.68509585594499356, -8.352346156331998728 ) ) ;
#51280=CARTESIAN_POINT ( 'NONE',  ( -0.5337471080167767168, -79.79999999999999716, -11.78542848578489455 ) ) ;
#51284=CARTESIAN_POINT ( 'NONE',  ( 10.02574878253000001, -76.55263728987598881, 4.955627619753999902 ) ) ;
#51294=CARTESIAN_POINT ( 'NONE',  ( -11.31676683693000030, -79.47839125786400416, 4.558499636902999974 ) ) ;
#51296=CARTESIAN_POINT ( 'NONE',  ( -10.75000000000000000, -78.10000000000000853, 0.000000000000000000 ) ) ;
#51313=CARTESIAN_POINT ( 'NONE',  ( 7.941842383120999216, -80.39595877905549060, -8.023044940210999343 ) ) ;
#51317=CARTESIAN_POINT ( 'NONE',  ( -7.803863155890000236, -78.33791210329199828, 8.057160196619001624 ) ) ;
#51322=AXIS2_PLACEMENT_3D ( 'NONE', #17856, #57701, #31406 ) ;
#51332=CARTESIAN_POINT ( 'NONE',  ( -1.863462560416999869, -78.14610176985598855, 12.02123279331999939 ) ) ;
#51334=CARTESIAN_POINT ( 'NONE',  ( 7.083968241731952276, -78.68188980497933471, -8.167169251009076092 ) ) ;
#51342=CARTESIAN_POINT ( 'NONE',  ( -1.596083865962000026, -78.46008588794200023, 10.79943897993000057 ) ) ;
#51346=DIRECTION ( 'NONE',  ( 0.000000000000000000, 1.000000000000000000, 0.000000000000000000 ) ) ;
#51356=CARTESIAN_POINT ( 'NONE',  ( 5.413904038987179312, -77.66666666666664298, -9.393203674808262349 ) ) ;
#51361=CARTESIAN_POINT ( 'NONE',  ( 7.144724566336000393, -76.45948425134299953, 9.988770583665001368 ) ) ;
#51371=CARTESIAN_POINT ( 'NONE',  ( 0.000000000000000000, -80.79999999999999716, 0.000000000000000000 ) ) ;
#51373=CARTESIAN_POINT ( 'NONE',  ( 4.975516581814000361, -78.09966785968099146, -11.10075516933000017 ) ) ;
#51377=CARTESIAN_POINT ( 'NONE',  ( -7.105843098096999988, -79.45799394121699777, 8.287482117959999783 ) ) ;
#51378=CARTESIAN_POINT ( 'NONE',  ( -10.46802440259882694, -79.58158398553671020, 2.476077618161485638 ) ) ;
#51386=CYLINDRICAL_SURFACE ( 'NONE', #6277, 10.75000000000000000 ) ;
#51391=CARTESIAN_POINT ( 'NONE',  ( 6.793663275700000170, -79.45312102823399414, -8.982210410292001512 ) ) ;
#51393=CARTESIAN_POINT ( 'NONE',  ( -11.62703158103455436, -79.06212265249649818, -1.840488976840387592 ) ) ;
#51396=B_SPLINE_CURVE_WITH_KNOTS ( 'NONE', 3,
 ( #11073, #29053, #24921, #2213, #38203, #28755, #24347, #42938, #2492, #42358, #20498, #1928, #19921, #56223, #41767, #19335, #28168, #37911 ),
 .UNSPECIFIED., .F., .F.,
 ( 4, 2, 2, 2, 2, 2, 2, 2, 4 ),
 ( 0.000000000000000000, 0.1250000000000000278, 0.2500000000000000555, 0.3750000000000000000, 0.5000000000000000000, 0.6250000000000000000, 0.7500000000000000000, 0.8750000000000001110, 1.000000000000000000 ),
 .UNSPECIFIED. ) ;
#51409=ORIENTED_EDGE ( 'NONE', *, *, #7186, .F. ) ;
#51412=CARTESIAN_POINT ( 'NONE',  ( 8.509671453119294071, -78.79784401220496193, -6.569625457439239646 ) ) ;
#51418=CARTESIAN_POINT ( 'NONE',  ( 10.75022122707607508, -79.83959204947723265, -1.407073340423293351 ) ) ;
#51421=CARTESIAN_POINT ( 'NONE',  ( 10.93160348586000019, -79.10187956322499758, 2.513594203403000105 ) ) ;
#51428=CARTESIAN_POINT ( 'NONE',  ( 9.144505818845814815, -77.55075625647234006, -6.496123635900521442 ) ) ;
#51429=UNCERTAINTY_MEASURE_WITH_UNIT (LENGTH_MEASURE( 1.000000000000000082E-05 ), #40420, 'distance_accuracy_value', 'NONE');
#51437=DIRECTION ( 'NONE',  ( 0.000000000000000000, -1.000000000000000000, 0.000000000000000000 ) ) ;
#51444=CARTESIAN_POINT ( 'NONE',  ( 9.576252206595992078, -77.88770107411112065, 4.884226988090900612 ) ) ;
#51445=CARTESIAN_POINT ( 'NONE',  ( 11.36821324764999908, -77.85835662174498850, -3.778861202892000115 ) ) ;
#51452=CARTESIAN_POINT ( 'NONE',  ( 4.205198518925999274, -77.11498468449899235, -10.19892346455999999 ) ) ;
#51453=CARTESIAN_POINT ( 'NONE',  ( -12.27595451888000078, -76.14772448534918681, 0.3505736730271999391 ) ) ;
#51454=CARTESIAN_POINT ( 'NONE',  ( -1.570796326794885012, -78.41458333333332575, -12.00000000000000178 ) ) ;
#51460=CARTESIAN_POINT ( 'NONE',  ( 3.895497176768000003, -77.11288127666699665, 10.51870773133999926 ) ) ;
#51464=CARTESIAN_POINT ( 'NONE',  ( -2.552548608664000351, -76.46843057132498700, 11.88149999858000072 ) ) ;
#51483=CARTESIAN_POINT ( 'NONE',  ( 5.828547835401000299, -78.55992220834100692, -9.501726143737998953 ) ) ;
#51498=CARTESIAN_POINT ( 'NONE',  ( -10.39759693597000023, -79.72892006072399340, -4.208097972746998927 ) ) ;
#51503=CARTESIAN_POINT ( 'NONE',  ( 10.81758370282001103, -76.04999999999998295, -2.303648478522546394 ) ) ;
#51521=EDGE_CURVE ( 'NONE', #34745, #28917, #49386, .T. ) ;
#51522=FACE_OUTER_BOUND ( 'NONE', #44959, .T. ) ;
#51524=VECTOR ( 'NONE', #8562, 1000.000000000000000 ) ;
#51534=CARTESIAN_POINT ( 'NONE',  ( 3.514783469115777770, -79.44852014850161481, 10.18303985929887823 ) ) ;
#51545=CARTESIAN_POINT ( 'NONE',  ( 7.605146568930318374, -80.28753541715676079, -7.597634579134508570 ) ) ;
#51549=ORIENTED_EDGE ( 'NONE', *, *, #47673, .T. ) ;
#51550=CARTESIAN_POINT ( 'NONE',  ( 10.43959491470999978, -79.77472838834199820, -5.976816984917999953 ) ) ;
#51554=CARTESIAN_POINT ( 'NONE',  ( -7.587128856971000701, -78.55323394950600857, 9.212544607993001122 ) ) ;
#51558=CARTESIAN_POINT ( 'NONE',  ( 6.606377239730313988, -78.82291666666665719, 8.596418555780454440 ) ) ;
#51563=ORIENTED_EDGE ( 'NONE', *, *, #12281, .F. ) ;
#51571=CARTESIAN_POINT ( 'NONE',  ( 11.76049068545964005, -79.80000000000002558, 0.9294003827681622809 ) ) ;
#51575=CARTESIAN_POINT ( 'NONE',  ( 9.776276929627000456, -75.97575262412699715, -5.431214116490000521 ) ) ;
#51577=EDGE_CURVE ( 'NONE', #42525, #15494, #30321, .T. ) ;
#51580=CARTESIAN_POINT ( 'NONE',  ( 4.873378631631000601, -76.55225832436200051, -9.988483505024001730 ) ) ;
#51587=CARTESIAN_POINT ( 'NONE',  ( -1.777040666284000148, -79.89549482803428759, 12.07019270111999987 ) ) ;
#51588=CARTESIAN_POINT ( 'NONE',  ( -9.932012650257558306, -78.06882224905531587, 4.112984229135753012 ) ) ;
#51603=VERTEX_POINT ( 'NONE', #35905 ) ;
#51604=AXIS2_PLACEMENT_3D ( 'NONE', #20993, #22665, #4059 ) ;
#51606=CARTESIAN_POINT ( 'NONE',  ( 0.3809989338272000703, -80.14893166943579672, 11.39926455542999939 ) ) ;
#51610=CARTESIAN_POINT ( 'NONE',  ( -11.14038684213999986, -78.39238478929600262, 1.307628137226999998 ) ) ;
#51615=LINE ( 'NONE', #56323, #18043 ) ;
#51627=CARTESIAN_POINT ( 'NONE',  ( -12.04425331849999914, -78.77007602460300006, -1.708359618215999909 ) ) ;
#51629=CARTESIAN_POINT ( 'NONE',  ( -0.7035581186724901848, -77.48024153129969704, 10.74957510668601834 ) ) ;
#51638=CARTESIAN_POINT ( 'NONE',  ( -0.4035379437255999791, -79.19546714899098561, -10.90928609572000063 ) ) ;
#51647=ADVANCED_FACE ( 'NONE', ( #45963 ), #18500, .T. ) ;
#51655=CARTESIAN_POINT ( 'NONE',  ( 10.75000000000000355, -77.73958333333331439, -1.407171709420407035 ) ) ;
#51660=CARTESIAN_POINT ( 'NONE',  ( 8.135116633385999663, -76.88348855772599677, 9.200136113044999675 ) ) ;
#51663=CARTESIAN_POINT ( 'NONE',  ( -4.152600241220000044, -79.34482178677752984, -10.41988588363999924 ) ) ;
#51665=ORIENTED_EDGE ( 'NONE', *, *, #18523, .T. ) ;
#51671=CARTESIAN_POINT ( 'NONE',  ( 11.88272347344000046, -77.27212751510998601, 1.999161996513999950 ) ) ;
#51675=CARTESIAN_POINT ( 'NONE',  ( -1.433413778493000112, -78.64090365116300063, -10.60928646434000200 ) ) ;
#51676=CARTESIAN_POINT ( 'NONE',  ( -10.54819193961059121, -79.58468236046442712, 2.072783446717219924 ) ) ;
#51687=CARTESIAN_POINT ( 'NONE',  ( -1.646570173782999857, -78.66326708118100441, 11.14103995232000166 ) ) ;
#51688=CARTESIAN_POINT ( 'NONE',  ( 11.02013089939147683, -76.58625517782145664, -1.906531608818739176 ) ) ;
#51690=CARTESIAN_POINT ( 'NONE',  ( 5.137083998358000336, -77.31100733245999379, -10.56753840748999984 ) ) ;
#51703=CARTESIAN_POINT ( 'NONE',  ( -11.98432456299000037, -77.28116005809600608, -3.448566798086999619 ) ) ;
#51704=CARTESIAN_POINT ( 'NONE',  ( 2.102229583188283346, -78.74079288752511729, -10.54235425007153992 ) ) ;
#51712=CARTESIAN_POINT ( 'NONE',  ( 11.15679540746000065, -79.59213373725799556, 1.159321710118000004 ) ) ;
#51716=ADVANCED_FACE ( 'NONE', ( #36781 ), #13468, .F. ) ;
#51719=CARTESIAN_POINT ( 'NONE',  ( 6.330072429688197388, -78.17719214551432572, 9.260226347063357011 ) ) ;
#51727=CARTESIAN_POINT ( 'NONE',  ( -11.15966350340000091, -79.61955349143056537, 4.490997254915999548 ) ) ;
#51732=CARTESIAN_POINT ( 'NONE',  ( 1.570796326794910547, -79.53541666666666288, -11.99999999999999822 ) ) ;
#51734=CARTESIAN_POINT ( 'NONE',  ( -1.407167113863494023, -79.21473436249412714, -10.75055113178693844 ) ) ;
#51736=CARTESIAN_POINT ( 'NONE',  ( 6.444980599754999595, -77.80409799089798639, -10.09843005143000028 ) ) ;
#51739=CARTESIAN_POINT ( 'NONE',  ( -11.02533051454918400, -76.36625311331162891, 4.903865969626981069 ) ) ;
#51740=CARTESIAN_POINT ( 'NONE',  ( 9.430214174385252335, -80.89008252689569645, 5.160773662914198034 ) ) ;
#51743=CARTESIAN_POINT ( 'NONE',  ( -10.95663201459999847, -78.44956549158798964, 1.286059498161999937 ) ) ;
#51744=CARTESIAN_POINT ( 'NONE',  ( 4.196317941609000179, -80.68300621547570017, -10.07146971829999949 ) ) ;
#51750=CARTESIAN_POINT ( 'NONE',  ( -10.58728162385000005, -77.73931716570899653, 3.705074683290000337 ) ) ;
#51762=CARTESIAN_POINT ( 'NONE',  ( -12.00000000000000178, -76.81041666666666856, -1.570796326794897890 ) ) ;
#51763=CARTESIAN_POINT ( 'NONE',  ( 6.043427764450807871, -79.46666666666666856, -10.48543666025108934 ) ) ;
#51781=CARTESIAN_POINT ( 'NONE',  ( 10.01578477942999967, -77.35596644471499417, 4.342743515613999961 ) ) ;
#51790=VERTEX_POINT ( 'NONE', #10517 ) ;
#51792=CARTESIAN_POINT ( 'NONE',  ( -11.36512682855694933, -76.92683455540999660, -3.982123233434259557 ) ) ;
#51803=CARTESIAN_POINT ( 'NONE',  ( -1.407069491366080172, -76.71471916496845722, -10.74971761791662672 ) ) ;
#51806=CARTESIAN_POINT ( 'NONE',  ( 0.000000000000000000, -87.29999999999999716, 0.000000000000000000 ) ) ;
#51820=CARTESIAN_POINT ( 'NONE',  ( -10.68082442906623797, -77.08973694601026239, 1.407256659424358070 ) ) ;
#51822=CARTESIAN_POINT ( 'NONE',  ( 2.157438503070702840, -79.45895713229609214, 10.55436150663177663 ) ) ;
#51826=CARTESIAN_POINT ( 'NONE',  ( 2.264809212410999647E-14, -92.79999999999999716, 0.000000000000000000 ) ) ;
#51830=CARTESIAN_POINT ( 'NONE',  ( 8.230685248251999653, -77.89996571856799790, -7.517341346183999740 ) ) ;
#51835=CARTESIAN_POINT ( 'NONE',  ( 7.429570834404548130, -80.28571891368410718, -7.771422698336870383 ) ) ;
#51839=CARTESIAN_POINT ( 'NONE',  ( 8.348735229153000148, -78.94600801619300512, 8.268078378528999295 ) ) ;
#51857=CARTESIAN_POINT ( 'NONE',  ( -7.533402290670649926, -79.79999999999999716, -9.189679446819413400 ) ) ;
#51858=CARTESIAN_POINT ( 'NONE',  ( -8.652941401739491667, -80.04965019796203762, 6.378618437432542976 ) ) ;
#51862=CARTESIAN_POINT ( 'NONE',  ( -1.660522255173999984, -76.78854216438499236, 11.05968181062000077 ) ) ;
#51865=CARTESIAN_POINT ( 'NONE',  ( 7.729696734268999947, -76.57734026635199598, -7.985700370870999265 ) ) ;
#51872=CARTESIAN_POINT ( 'NONE',  ( -2.502260836693999568, -79.61742578125399916, -11.94101425180999954 ) ) ;
#51873=CARTESIAN_POINT ( 'NONE',  ( -9.295691395107468225, -78.05822132751052322, 5.400626663501747693 ) ) ;
#51897=CARTESIAN_POINT ( 'NONE',  ( 0.000000000000000000, -75.15999999999999659, 0.000000000000000000 ) ) ;
#51908=CARTESIAN_POINT ( 'NONE',  ( 6.233047529871999615, -78.88050366622999832, 9.960502923565000444 ) ) ;
#51910=CARTESIAN_POINT ( 'NONE',  ( 11.71313121114000033, -78.98711054799299802, -3.284064838691000077 ) ) ;
#51921=CARTESIAN_POINT ( 'NONE',  ( 6.695505957611000092, -78.89586737597099386, 8.622387486181999350 ) ) ;
#51924=CARTESIAN_POINT ( 'NONE',  ( -8.595201249227393703, -80.65211028413133931, -6.605388001086274663 ) ) ;
#51941=CARTESIAN_POINT ( 'NONE',  ( -7.650089724727000551, -76.56980357461999631, -9.607224057717001386 ) ) ;
#51944=DIRECTION ( 'NONE',  ( 0.000000000000000000, -1.000000000000000000, 0.000000000000000000 ) ) ;
#51951=CARTESIAN_POINT ( 'NONE',  ( -11.92228046151999976, -78.42521964476598839, 2.416973144693999931 ) ) ;
#51955=CARTESIAN_POINT ( 'NONE',  ( -10.90022919700999893, -79.02221245318798992, 0.6003077901278000006 ) ) ;
#51956=CARTESIAN_POINT ( 'NONE',  ( -9.946797292890842357, -79.56914397919975102, 4.077092203015069138 ) ) ;
#51959=LINE ( 'NONE', #29494, #11665 ) ;
#51968=CARTESIAN_POINT ( 'NONE',  ( 11.18604332926000033, -79.01733954020500050, -1.306292155029999957 ) ) ;
#51969=CARTESIAN_POINT ( 'NONE',  ( -1.432444700303164398, -76.23510798997345717, 11.09171988620980187 ) ) ;
#51974=B_SPLINE_CURVE_WITH_KNOTS ( 'NONE', 3,
 ( #54379, #17180, #22187, #8322, #9498, #3890, #21892, #21610, #49953, #58210, #44059, #17771, #39617, #57623, #35760, #35166, #53790, #37222, #36643, #23066, #15382, #41080, #10088, #1820, #46703, #27483, #5933, #23364, #54662, #36933, #33376, #28067, #5356, #46114, #37810, #42257, #10675, #55831, #19521, #6224, #32489, #15080, #55532, #10371, #51412, #5639, #19817, #32201, #14203, #45525, #51122, #27777, #5070, #50241, #9791, #41956, #671, #18656, #41375, #957, #33077, #28654, #1526, #28359, #24239, #45820, #46406, #18941, #23938, #23649, #54945, #37514, #14496, #50533, #41662, #1241, #19231, #55238, #14784, #32781, #50826, #24818, #16254, #6518, #51988, #43701, #30088, #10965, #47855, #6810, #20110, #20390, #57264, #11542, #47281, #29519, #21246, #25674, #52551, #39248, #2962, #56977, #15667, #16539, #38965, #52269, #16830, #47575, #3257, #33664, #38101, #28948, #34519, #11252, #34812, #51704, #29232, #25385, #46990, #24528, #42833, #2394, #12106, #48141, #15957, #11823, #7672, #38676, #56408, #42543, #20960, #56121, #2111, #38388, #7384, #43400, #33948, #7101, #25100, #43124, #2683, #20677, #56696, #34232, #29799, #39542, #49591, #4711, #17995, #39827, #27122, #30382, #13553, #22710, #12392, #9137, #35689, #54012, #49288, #45162, #48421, #44266, #22112, #57548, #40723, #48992, #58134, #21823, #315, #4111, #3821, #48706, #26829, #40121 ),
 .UNSPECIFIED., .F., .F.,
 ( 4, 2, 2, 2, 1, 1, 1, 2, 2, 2, 2, 1, 1, 1, 1, 1, 2, 2, 2, 2, 2, 1, 1, 1, 1, 2, 2, 2, 1, 2, 2, 1, 1, 1, 1, 1, 1, 2, 2, 2, 2, 2, 1, 1, 1, 2, 2, 2, 2, 1, 1, 1, 2, 2, 2, 2, 1, 1, 1, 2, 2, 2, 1, 1, 1, 1, 1, 2, 2, 2, 2, 2, 1, 1, 1, 1, 2, 2, 2, 2, 1, 1, 2, 2, 2, 2, 2, 2, 2, 1, 1, 1, 2, 2, 2, 1, 1, 2, 2, 1, 1, 2, 2, 2, 2, 1, 2, 2, 1, 2, 4 ),
 ( 0.000000000000000000, 0.03125000000001028344, 0.04687500000001543904, 0.05468750000001802031, 0.05859375000001933176, 0.06054687500001998401, 0.06152343750002028933, 0.06201171875002044198, 0.06250000000002059464, 0.09375000000002767231, 0.1093750000000312250, 0.1171875000000330153, 0.1210937500000338479, 0.1230468750000342781, 0.1240234375000345557, 0.1245117187500346806, 0.1247558593750347222, 0.1250000000000347500, 0.1562500000000413836, 0.1718750000000447142, 0.1796875000000463518, 0.1835937500000472122, 0.1855468750000476008, 0.1865234375000477673, 0.1870117187500478784, 0.1872558593750479339, 0.1875000000000479894, 0.2031250000000475731, 0.2109375000000473233, 0.2148437500000472122, 0.2187500000000471012, 0.2343750000000465461, 0.2421875000000462408, 0.2460937500000460743, 0.2480468750000459355, 0.2490234375000458522, 0.2495117187500458522, 0.2497558593750458522, 0.2500000000000458522, 0.2656250000000456857, 0.2734375000000455191, 0.2773437500000454081, 0.2792968750000453526, 0.2802734375000452416, 0.2807617187500451861, 0.2810058593750451861, 0.2812500000000451306, 0.2968750000000437428, 0.3046875000000430767, 0.3085937500000427991, 0.3105468750000426326, 0.3115234375000425771, 0.3120117187500426326, 0.3125000000000426326, 0.3281250000000437983, 0.3359375000000443534, 0.3398437500000446865, 0.3417968750000447975, 0.3427734375000449085, 0.3432617187500449640, 0.3437500000000450195, 0.3593750000000483502, 0.3671875000000500711, 0.3710937500000509592, 0.3730468750000513478, 0.3740234375000516254, 0.3745117187500517364, 0.3747558593750517919, 0.3750000000000517919, 0.4062500000000540679, 0.4218750000000552336, 0.4296875000000557887, 0.4335937500000561218, 0.4355468750000562883, 0.4365234375000562883, 0.4370117187500562328, 0.4372558593750562328, 0.4375000000000562328, 0.4687500000000556777, 0.4843750000000553446, 0.4921875000000552336, 0.4960937500000551226, 0.4980468750000550671, 0.5000000000000550671, 0.5625000000000539568, 0.6250000000000528466, 0.6406250000000527356, 0.6425781250000527356, 0.6435546875000526246, 0.6445312500000526246, 0.6484375000000526246, 0.6562500000000525135, 0.6875000000000519584, 0.7500000000000506262, 0.8125000000000492939, 0.8437500000000486278, 0.8476562500000485167, 0.8496093750000485167, 0.8500976562500485167, 0.8505859375000484057, 0.8515625000000484057, 0.8593750000000480727, 0.8750000000000474065, 0.9062500000000462963, 0.9218750000000457412, 0.9238281250000458522, 0.9248046875000452971, 0.9257812500000447420, 0.9296875000000424105, 0.9375000000000376366, 1.000000000000000000 ),
 .UNSPECIFIED. ) ;
#51981=CARTESIAN_POINT ( 'NONE',  ( 10.89560438185736579, -76.15405317179865108, -1.138875632008489180 ) ) ;
#51982=CARTESIAN_POINT ( 'NONE',  ( 10.75008527255733881, -78.36041959662934175, 1.407065630674559698 ) ) ;
#51984=EDGE_LOOP ( 'NONE', ( #307, #54148, #47572, #31401 ) ) ;
#51986=EDGE_LOOP ( 'NONE', ( #39813, #40865, #9052, #54675 ) ) ;
#51987=CARTESIAN_POINT ( 'NONE',  ( 4.364318959196999970, -76.91231541335099564, -11.68200350210999972 ) ) ;
#51988=CARTESIAN_POINT ( 'NONE',  ( 5.563604409980168697, -78.76841996384091260, -9.198609774334910227 ) ) ;
#51989=EDGE_LOOP ( 'NONE', ( #13617, #46555 ) ) ;
#51997=CARTESIAN_POINT ( 'NONE',  ( -2.848564863371000122, -78.93846150521399352, -10.84913769893999991 ) ) ;
#51998=ORIENTED_EDGE ( 'NONE', *, *, #44777, .F. ) ;
#52005=CARTESIAN_POINT ( 'NONE',  ( -5.751514107123901987, -77.93206505849833832, -9.630248929252696044 ) ) ;
#52009=CARTESIAN_POINT ( 'NONE',  ( -1.407171709420465211, -80.88541666666667140, 10.74999999999999467 ) ) ;
#52019=FACE_OUTER_BOUND ( 'NONE', #5337, .T. ) ;
#52020=CARTESIAN_POINT ( 'NONE',  ( -10.26943924278000075, -78.45527103163399829, 6.168847710360999770 ) ) ;
#52024=CARTESIAN_POINT ( 'NONE',  ( 8.098718378555803454, -78.90743983794655492, 7.103735875983660186 ) ) ;
#52029=CARTESIAN_POINT ( 'NONE',  ( -4.457153411444000568, -77.55076617252800020, -10.09135857296999994 ) ) ;
#52030=CARTESIAN_POINT ( 'NONE',  ( -10.88526732619999926, -81.03202613352289063, -0.7446763694950000456 ) ) ;
#52036=CARTESIAN_POINT ( 'NONE',  ( -8.649885944100999424, -77.82102619471399407, -7.141259254888000285 ) ) ;
#52049=CARTESIAN_POINT ( 'NONE',  ( 9.596002108778172612, -76.99791666666666856, -7.374560639698962028 ) ) ;
#52065=ORIENTED_EDGE ( 'NONE', *, *, #36471, .T. ) ;
#52067=CARTESIAN_POINT ( 'NONE',  ( 4.161322419204999790, -76.72953055567299430, -10.09251018087000062 ) ) ;
#52076=CYLINDRICAL_SURFACE ( 'NONE', #7843, 12.00000000000000000 ) ;
#52104=CARTESIAN_POINT ( 'NONE',  ( -1.407080327196711611, -76.98557767287246634, 10.75010754519202294 ) ) ;
#52106=CARTESIAN_POINT ( 'NONE',  ( -11.70000000000000107, -79.79999999999999716, 0.000000000000000000 ) ) ;
#52112=CARTESIAN_POINT ( 'NONE',  ( -10.47919054151000040, -77.73654766055700804, -3.800153439748000128 ) ) ;
#52123=CARTESIAN_POINT ( 'NONE',  ( -12.02912753549999891, -79.49775441913300256, 0.08506824670321999626 ) ) ;
#52125=CARTESIAN_POINT ( 'NONE',  ( 3.385018580295000135, -79.47270349199298778, -10.74130410002999980 ) ) ;
#52131=EDGE_LOOP ( 'NONE', ( #50828, #4107 ) ) ;
#52132=CARTESIAN_POINT ( 'NONE',  ( 0.000000000000000000, -75.15999999999999659, 0.000000000000000000 ) ) ;
#52144=CARTESIAN_POINT ( 'NONE',  ( -6.907231294620150841, -80.03091450954583763, 8.236999994290794547 ) ) ;
#52148=CARTESIAN_POINT ( 'NONE',  ( 8.154961773732001262, -76.14386894535999772, 7.653135223926000208 ) ) ;
#52152=CARTESIAN_POINT ( 'NONE',  ( -1.633132813051000110, -76.84572286667699359, 10.87725817015999930 ) ) ;
#52160=CARTESIAN_POINT ( 'NONE',  ( -10.19309198600624811, -78.07437978168276516, 3.419625436452577549 ) ) ;
#52165=CARTESIAN_POINT ( 'NONE',  ( 6.233047529871999615, -78.88050366622999832, 9.960502923565000444 ) ) ;
#52166=ADVANCED_FACE ( 'NONE', ( #34380 ), #35814, .F. ) ;
#52168=CARTESIAN_POINT ( 'NONE',  ( 2.813789756862240754, -80.14583333333330017, -10.47020627418439886 ) ) ;
#52184=CARTESIAN_POINT ( 'NONE',  ( -1.620259408620695396, -79.98748962049585032, 10.62691779879149401 ) ) ;
#52195=CARTESIAN_POINT ( 'NONE',  ( 11.60231809276000092, -78.91938348357999189, -3.252995651540999678 ) ) ;
#52212=CARTESIAN_POINT ( 'NONE',  ( 6.586108526242999694, -80.17391735373439587, 8.810401493720998900 ) ) ;
#52231=CARTESIAN_POINT ( 'NONE',  ( 10.33787006668000075, -78.23531443679999597, 6.411783922571999916 ) ) ;
#52240=CARTESIAN_POINT ( 'NONE',  ( 1.151100648512999980, -79.05851746904299659, 11.98613337465000050 ) ) ;
#52245=FACE_OUTER_BOUND ( 'NONE', #51984, .T. ) ;
#52247=CARTESIAN_POINT ( 'NONE',  ( 3.140974612311376646, -78.04583333333330586, -11.68767212001978706 ) ) ;
#52250=CARTESIAN_POINT ( 'NONE',  ( -1.660550560716740121, -76.73674682975610040, 11.05987033582087165 ) ) ;
#52251=CARTESIAN_POINT ( 'NONE',  ( -4.656159886366224576, -78.95671637029290935, 10.88172775970164707 ) ) ;
#52261=CARTESIAN_POINT ( 'NONE',  ( 8.899186938124000079, -76.04999999999999716, -6.465637775218000094 ) ) ;
#52266=ORIENTED_EDGE ( 'NONE', *, *, #11850, .F. ) ;
#52267=CARTESIAN_POINT ( 'NONE',  ( 11.79063559949999984, -77.03526362826599438, 4.061698893270999200 ) ) ;
#52268=APPLICATION_CONTEXT ( 'automotive_design' ) ;
#52269=CARTESIAN_POINT ( 'NONE',  ( 3.187863135131073111, -78.74905765371072164, -10.27228247429871999 ) ) ;
#52270=ORIENTED_EDGE ( 'NONE', *, *, #56196, .F. ) ;
#52278=CARTESIAN_POINT ( 'NONE',  ( -7.301194973305000779, -79.26529762123598744, 8.515319286630999684 ) ) ;
#52286=CARTESIAN_POINT ( 'NONE',  ( -10.05549647464921570, -78.31337386052332761, 4.970774552467315921 ) ) ;
#52299=DIRECTION ( 'NONE',  ( 1.000000000000000000, 0.000000000000000000, 0.000000000000000000 ) ) ;
#52300=VERTEX_POINT ( 'NONE', #27608 ) ;
#52306=CARTESIAN_POINT ( 'NONE',  ( -10.86788298907000083, -77.60066286050300732, -5.040355520269000245 ) ) ;
#52313=CARTESIAN_POINT ( 'NONE',  ( 0.2583767295275999909, -78.65347427100999766, -10.91369642039000176 ) ) ;
#52319=CARTESIAN_POINT ( 'NONE',  ( -12.22925423141000145, -79.83317873820959676, -1.014767581180999967 ) ) ;
#52321=DIRECTION ( 'NONE',  ( 0.000000000000000000, -1.000000000000000000, 0.000000000000000000 ) ) ;
#52322=CARTESIAN_POINT ( 'NONE',  ( -10.54491486739000017, -77.86157840498900384, -3.823987582478999947 ) ) ;
#52326=CARTESIAN_POINT ( 'NONE',  ( 0.4138966918734000022, -76.20430140319000145, -12.14554839628999972 ) ) ;
#52330=CARTESIAN_POINT ( 'NONE',  ( -10.33279081301000168, -79.73946642284398933, -4.181869747484999955 ) ) ;
#52353=CARTESIAN_POINT ( 'NONE',  ( 10.50536548972000084, -77.30149375871098982, -2.968612793496999913 ) ) ;
#52375=CARTESIAN_POINT ( 'NONE',  ( -7.615853692923001184, -78.63150737603899643, 9.247423260715999405 ) ) ;
#52381=CARTESIAN_POINT ( 'NONE',  ( 10.80251317621999974, -78.09622061874799215, 3.184285419974999698 ) ) ;
#52393=CARTESIAN_POINT ( 'NONE',  ( 8.596118241356434098, -76.90225025436217265, 6.606116134054767386 ) ) ;
#52400=CARTESIAN_POINT ( 'NONE',  ( 5.119217263405000828, -77.54589325954400181, 9.901929871541000239 ) ) ;
#52406=CARTESIAN_POINT ( 'NONE',  ( 7.043910409642034409, -80.28198538032874865, -8.120786863705317771 ) ) ;
#52407=CARTESIAN_POINT ( 'NONE',  ( 10.65248731882857491, -79.86234087736364984, 1.664133241301937405 ) ) ;
#52409=CARTESIAN_POINT ( 'NONE',  ( 10.43959491470999978, -79.70693983506599523, -5.976816984917999953 ) ) ;
#52414=ORIENTED_EDGE ( 'NONE', *, *, #25946, .F. ) ;
#52425=ORIENTED_EDGE ( 'NONE', *, *, #27902, .T. ) ;
#52432=CARTESIAN_POINT ( 'NONE',  ( 7.995633008690000487, -76.71329633841800444, 7.819446035993999899 ) ) ;
#52435=CARTESIAN_POINT ( 'NONE',  ( 1.819226710355999810, -76.82064092468800709, 10.84768487502000056 ) ) ;
#52441=CARTESIAN_POINT ( 'NONE',  ( -4.129275505618361208, -78.00639181381374954, 9.925283770886389689 ) ) ;
#52443=CARTESIAN_POINT ( 'NONE',  ( -2.624566716334498562, -80.99486133380281672, 10.45026324297856313 ) ) ;
#52451=CARTESIAN_POINT ( 'NONE',  ( 5.246383657897999875, -77.06100733245999379, -10.79237965019999912 ) ) ;
#52458=CARTESIAN_POINT ( 'NONE',  ( -10.87500000000999911, -76.17499999999400018, 1.221063213659000093E-09 ) ) ;
#52465=CARTESIAN_POINT ( 'NONE',  ( 4.210840025191989078, -79.94311247203964399, 9.890888605214144036 ) ) ;
#52473=ORIENTED_EDGE ( 'NONE', *, *, #54435, .T. ) ;
#52495=CARTESIAN_POINT ( 'NONE',  ( -11.18477258988041179, -80.85528771549159899, -0.7651659436797575431 ) ) ;
#52499=AXIS2_PLACEMENT_3D ( 'NONE', #44741, #53302, #12845 ) ;
#52504=CARTESIAN_POINT ( 'NONE',  ( -3.164411967817999827, -77.10257917258499560, -11.86639179494000018 ) ) ;
#52515=CARTESIAN_POINT ( 'NONE',  ( 11.86727826211999925, -77.24499819968599468, -2.088899193827999934 ) ) ;
#52522=CARTESIAN_POINT ( 'NONE',  ( 5.462882135474435685, -78.73756601347038497, 10.73736906863111251 ) ) ;
#52523=CARTESIAN_POINT ( 'NONE',  ( -3.728673265761000000, -79.59119008599400047, 11.44942132006000080 ) ) ;
#52525=CARTESIAN_POINT ( 'NONE',  ( -3.708203932498999933, -79.79999999999999716, 11.41267819554000162 ) ) ;
#52527=CARTESIAN_POINT ( 'NONE',  ( 0.000000000000000000, -90.29999999999999716, 0.000000000000000000 ) ) ;
#52533=CARTESIAN_POINT ( 'NONE',  ( 4.510348846891466756, -79.20585849186471705, -10.94228070689720234 ) ) ;
#52540=LINE ( 'NONE', #20381, #5868 ) ;
#52543=VECTOR ( 'NONE', #37328, 1000.000000000000114 ) ;
#52544=CARTESIAN_POINT ( 'NONE',  ( 3.463640375329640531, -78.44897895074308281, 10.20056074439654914 ) ) ;
#52550=CARTESIAN_POINT ( 'NONE',  ( -7.841711555745998652, -76.89807700115400735, -9.847868799306999321 ) ) ;
#52551=CARTESIAN_POINT ( 'NONE',  ( 4.176452633942115966, -78.75676650919550070, -9.905560661817728985 ) ) ;
#52561=CARTESIAN_POINT ( 'NONE',  ( 8.596622369410699349, -79.79792950508202409, -6.606549433422280515 ) ) ;
#52564=CARTESIAN_POINT ( 'NONE',  ( 5.745747329289000227, -78.73388662847199271, 9.633509135241000720 ) ) ;
#52568=CARTESIAN_POINT ( 'NONE',  ( 0.000000000000000000, -80.89999999999999147, 0.000000000000000000 ) ) ;
#52583=CARTESIAN_POINT ( 'NONE',  ( -12.00000000000000000, -78.79999999999999716, 0.000000000000000000 ) ) ;
#52590=CARTESIAN_POINT ( 'NONE',  ( 10.75000000000000000, -79.35000000000000853, 0.000000000000000000 ) ) ;
#52591=CARTESIAN_POINT ( 'NONE',  ( 6.444980599754999595, -77.73630943762100287, -10.09843005143000028 ) ) ;
#52604=CARTESIAN_POINT ( 'NONE',  ( 11.01099501428000060, -79.54020879888699369, -5.416862536834000430 ) ) ;
#52611=CARTESIAN_POINT ( 'NONE',  ( -12.36772659745999903, -76.93670025537799972, 0.6901808088037000299 ) ) ;
#52615=CARTESIAN_POINT ( 'NONE',  ( 2.277702604431000033, -78.28268586533900475, -10.79414087890000040 ) ) ;
#52634=FACE_OUTER_BOUND ( 'NONE', #34394, .T. ) ;
#52655=CARTESIAN_POINT ( 'NONE',  ( -1.835125225091999823, -78.08892106756400153, 11.83842809849000055 ) ) ;
#52664=CARTESIAN_POINT ( 'NONE',  ( 9.107239040596999402, -78.12345696174899956, 6.625115969983998987 ) ) ;
#52668=CARTESIAN_POINT ( 'NONE',  ( 7.711243899566646576, -80.31159779477867744, 7.536022382359885086 ) ) ;
#52682=CARTESIAN_POINT ( 'NONE',  ( -10.98551332331999930, -76.63383956207499637, 1.010146990136999934 ) ) ;
#52688=CARTESIAN_POINT ( 'NONE',  ( -2.021764786808774250, -80.21014581661567888, -10.55807976612607391 ) ) ;
#52690=CARTESIAN_POINT ( 'NONE',  ( -8.382314651691611829, -79.90774747778513643, -7.453751407507572146 ) ) ;
#52692=CARTESIAN_POINT ( 'NONE',  ( -11.15966350340000091, -79.53565934156199546, 4.490997254915999548 ) ) ;
#52695=CARTESIAN_POINT ( 'NONE',  ( -9.103325846391999931, -78.87350394595299008, -6.630491919364000175 ) ) ;
#52699=CARTESIAN_POINT ( 'NONE',  ( -10.31421052434999908, -76.82175206120300004, 3.823226550887000030 ) ) ;
#52715=CARTESIAN_POINT ( 'NONE',  ( 3.670166320769038037, -79.79999999999999716, 11.34743833829017490 ) ) ;
#52716=CARTESIAN_POINT ( 'NONE',  ( -10.21315268674774757, -80.07477733434343747, 3.354632155474256194 ) ) ;
#52720=CARTESIAN_POINT ( 'NONE',  ( 4.903943924252999409, -76.49501613320700244, -10.05113017056000047 ) ) ;
#52723=CARTESIAN_POINT ( 'NONE',  ( 7.649879603444000864, -76.64506733076500211, -7.903239737143000987 ) ) ;
#52730=AXIS2_PLACEMENT_3D ( 'NONE', #39693, #12822, #17255 ) ;
#52732=CARTESIAN_POINT ( 'NONE',  ( 1.271183301036420188, -80.96600668877975693, 10.67466081527704880 ) ) ;
#52740=FACE_OUTER_BOUND ( 'NONE', #10030, .T. ) ;
#52747=CARTESIAN_POINT ( 'NONE',  ( 8.023850137665998972, -80.46368584346849673, -8.105891195326000442 ) ) ;
#52752=CARTESIAN_POINT ( 'NONE',  ( 2.721914423158461549, -79.95511695915216421, 10.40824526415593176 ) ) ;
#52775=CARTESIAN_POINT ( 'NONE',  ( -10.75045394575212399, -80.61043716274458859, -1.406899836902645973 ) ) ;
#52781=CARTESIAN_POINT ( 'NONE',  ( 1.949527607922329819, -80.21094325140447268, 11.04011390166788686 ) ) ;
#52790=CARTESIAN_POINT ( 'NONE',  ( -6.620362748380999918, -76.07801071496099610, -10.34376132320999986 ) ) ;
#52800=CONICAL_SURFACE ( 'NONE', #57510, 9.649999999909001147, 0.7853981633972997312 ) ;
#52801=CARTESIAN_POINT ( 'NONE',  ( 5.675825126306000001, -78.71017368086199895, 10.88946240266999865 ) ) ;
#52806=CARTESIAN_POINT ( 'NONE',  ( -7.294926994005753507, -79.53446014010890508, 7.905947034046361566 ) ) ;
#52809=CARTESIAN_POINT ( 'NONE',  ( -7.608356748847192819, -78.82937652759582647, 9.340614718762003221 ) ) ;
#52810=CARTESIAN_POINT ( 'NONE',  ( -9.494208634449000428, -79.13841836158600529, 7.406230482228999712 ) ) ;
#52813=DIRECTION ( 'NONE',  ( -0.7071067811864976127, 0.7071067811865975328, 1.603636560452993712E-09 ) ) ;
#52836=CARTESIAN_POINT ( 'NONE',  ( 4.405607986419999733, -76.98004247776398756, -11.79252213402000038 ) ) ;
#52837=EDGE_CURVE ( 'NONE', #23718, #9803, #45215, .T. ) ;
#52847=CARTESIAN_POINT ( 'NONE',  ( -9.998780405325002008, -77.28743033848687105, -5.083552005986999411 ) ) ;
#52850=CARTESIAN_POINT ( 'NONE',  ( -9.066796825632000179, -78.95177737248700112, -6.603885667862000375 ) ) ;
#52858=CARTESIAN_POINT ( 'NONE',  ( 12.00000000000000533, -77.14258394437167965, -1.118314842272784881 ) ) ;
#52875=CARTESIAN_POINT ( 'NONE',  ( 10.40649676915236554, -79.32929474332972575, -2.787393060167447700 ) ) ;
#52876=CARTESIAN_POINT ( 'NONE',  ( 11.79843486695000010, -77.30224039084099275, -2.076781258317999868 ) ) ;
#52895=CARTESIAN_POINT ( 'NONE',  ( 3.214918584686000003, -76.29524370419399304, 11.96249688184999904 ) ) ;
#52900=CARTESIAN_POINT ( 'NONE',  ( 9.298000630789001519, -78.93635809738199782, 5.937079976835999418 ) ) ;
#52907=CARTESIAN_POINT ( 'NONE',  ( -4.862705500402999981, -78.91919103528699964, -11.27607530993000040 ) ) ;
#52909=FACE_OUTER_BOUND ( 'NONE', #18625, .T. ) ;
#52914=ORIENTED_EDGE ( 'NONE', *, *, #15687, .T. ) ;
#52920=CARTESIAN_POINT ( 'NONE',  ( 2.565355593234150522, -81.00000000000000000, -10.72147822234086334 ) ) ;
#52921=CARTESIAN_POINT ( 'NONE',  ( -2.127308605635999772, -77.68280256073698808, -10.70747048031000048 ) ) ;
#52923=CARTESIAN_POINT ( 'NONE',  ( 11.21665020278000036, -78.44881193963800570, 0.06973997782872000395 ) ) ;
#52931=AXIS2_PLACEMENT_3D ( 'NONE', #48058, #25588, #43610 ) ;
#52942=CARTESIAN_POINT ( 'NONE',  ( -9.647309323447000651, -79.06128768769399073, -7.468504085378000035 ) ) ;
#52944=CARTESIAN_POINT ( 'NONE',  ( -11.86109855473999986, -78.71289532231099884, -1.682380905046999997 ) ) ;
#52951=CARTESIAN_POINT ( 'NONE',  ( 2.988858019399999844, -77.46978472970600649, -10.85820852157999994 ) ) ;
#52953=CARTESIAN_POINT ( 'NONE',  ( 7.524256684237999870, -80.50667270824050092, -8.371336685020999369 ) ) ;
#52955=DIRECTION ( 'NONE',  ( -1.000000000000000000, 0.000000000000000000, 0.000000000000000000 ) ) ;
#52956=ADVANCED_FACE ( 'NONE', ( #40993 ), #23848, .F. ) ;
#52961=CARTESIAN_POINT ( 'NONE',  ( -7.803863155890000236, -78.13454644346299460, 8.057160196619001624 ) ) ;
#52967=FACE_OUTER_BOUND ( 'NONE', #30594, .T. ) ;
#52977=CARTESIAN_POINT ( 'NONE',  ( 2.716004179693354281, -80.24554370127630420, -10.40178661565319729 ) ) ;
#52981=CARTESIAN_POINT ( 'NONE',  ( -6.309004353333000026, -79.14717214054400074, -10.24224633278999796 ) ) ;
#52983=CARTESIAN_POINT ( 'NONE',  ( -11.10951737771999959, -79.33652177698400010, -1.847319190731999905 ) ) ;
#52993=CARTESIAN_POINT ( 'NONE',  ( -8.741790450690999137, -79.52230326501299373, 6.538842841549999285 ) ) ;
#52997=CARTESIAN_POINT ( 'NONE',  ( 10.56370432582567176, -78.33298816678997412, -2.300065389339300825 ) ) ;
#53002=CARTESIAN_POINT ( 'NONE',  ( -6.975812051429156391, -80.03155649378894054, 8.179013189515927706 ) ) ;
#53008=CARTESIAN_POINT ( 'NONE',  ( 8.195399132537000142, -76.15178913831199736, -7.153224378557999863 ) ) ;
#53023=CARTESIAN_POINT ( 'NONE',  ( -12.00000000000000000, -79.29999999999999716, 0.000000000000000000 ) ) ;
#53025=EDGE_CURVE ( 'NONE', #27418, #10196, #51615, .T. ) ;
#53034=DIRECTION ( 'NONE',  ( 0.000000000000000000, 0.000000000000000000, -1.000000000000000000 ) ) ;
#53037=B_SPLINE_CURVE_WITH_KNOTS ( 'NONE', 3,
 ( #49770, #14019, #23177, #41185, #775, #18752, #9897, #1059, #55638, #56800 ),
 .UNSPECIFIED., .F., .F.,
 ( 4, 2, 2, 2, 4 ),
 ( 0.000000000000000000, 0.1250000012806290195, 0.2500000025612580390, 0.3750000038418869752, 0.5000000051225159670 ),
 .UNSPECIFIED. ) ;
#53039=CARTESIAN_POINT ( 'NONE',  ( 7.374560639698994002, -79.07708333333330586, -9.596002108778151296 ) ) ;
#53042=CARTESIAN_POINT ( 'NONE',  ( -1.607226962776981516, -79.98739046983742185, 10.62889775543116677 ) ) ;
#53050=CARTESIAN_POINT ( 'NONE',  ( 11.98062200086999951, -77.49499819968599468, -2.108850158091000182 ) ) ;
#53057=B_SPLINE_SURFACE_WITH_KNOTS ( 'NONE', 3, 3, ( 
 ( #50385, #22328, #54800, #40344, #53934, #49803, #9349, #45374, #13467, #4920, #22920, #14056, #9932, #31463, #27039, #27911, #55087, #42097, #6659, #19082, #33799, #24080, #1374, #6073, #46253, #11393, #56258, #15224, #33214, #10221, #14633, #19657, #50963, #14923, #46548 ),
 ( #50678, #32919, #10514, #45961, #1667, #19370, #37658, #19959, #5490, #55673, #28198, #23787, #23495, #5781, #28498, #51260, #41509, #10812, #37362, #28792, #37947, #1095, #46839, #41801, #55377, #37068, #20244, #24382, #24671, #15809, #6366, #55968, #42394, #1964, #51839 ),
 ( #15519, #32625, #33515, #51550, #11107, #38237, #42681, #29088, #47132, #2247, #16966, #52692, #29371, #57410, #47418, #56545, #34949, #11966, #25242, #39680, #21388, #8105, #34377, #47708, #52981, #12531, #38819, #29941, #42972, #6949, #2529, #24953, #25818, #12246, #20532 ),
 ( #21676, #16682, #38530, #52409, #57116, #7237, #16106, #30237, #26101, #48280, #52123, #30528, #3392, #34086, #7819, #47995, #3112, #43262, #39401, #48560, #11681, #2817, #56837, #29656, #43845, #7530, #44125, #20812, #16391, #3674, #17247, #25529, #57689, #43547, #21103 ) ),
 .UNSPECIFIED., .F., .F., .F.,
 ( 4, 4 ),
 ( 4, 1, 1, 1, 1, 1, 1, 1, 1, 1, 1, 1, 1, 1, 1, 1, 1, 1, 1, 1, 1, 1, 1, 1, 1, 1, 1, 1, 1, 1, 1, 1, 4 ),
 ( -0.5168282991433000850, 1.516828299142999992 ),
 ( 0.4382220305164999941, 0.4561218187598000129, 0.4740216070032000073, 0.4919213952464999706, 0.5098211834899000205, 0.5277209717331999839, 0.5456207599765999783, 0.5635205482198999416, 0.5814203364632999360, 0.5993201247066000104, 0.6172199129500000048, 0.6351197011933000791, 0.6530194894366999625, 0.6709192776799999258, 0.6888190659233000002, 0.7067188541666999946, 0.7246186424100000689, 0.7425184306533999523, 0.7604182188967000267, 0.7783180071401000211, 0.7962177953833999844, 0.8141175836267999788, 0.8320173718700999421, 0.8499171601134999365, 0.8678169483568000109, 0.8857167366002000053, 0.9036165248435000796, 0.9215163130869000740, 0.9394161013301999263, 0.9573158895735999208, 0.9752156778168999951, 0.9931154660602999895, 1.011015254303999855 ),
 .UNSPECIFIED. ) ;
#53067=FACE_OUTER_BOUND ( 'NONE', #51986, .T. ) ;
#53081=CARTESIAN_POINT ( 'NONE',  ( -9.596002108778161954, -77.85208333333332575, -7.374560639698982456 ) ) ;
#53088=CARTESIAN_POINT ( 'NONE',  ( 4.442094508599000235, -77.09588318900199511, -11.32474889210000057 ) ) ;
#53090=CARTESIAN_POINT ( 'NONE',  ( 1.407171709420440342, -79.13541666666665719, -10.74999999999999822 ) ) ;
#53094=CARTESIAN_POINT ( 'NONE',  ( -6.163538728152516022, -79.52360460267682640, 8.807809540774020007 ) ) ;
#53099=CARTESIAN_POINT ( 'NONE',  ( -8.792674058200999454, -79.75099187107899468, -8.226855735085999655 ) ) ;
#53102=CARTESIAN_POINT ( 'NONE',  ( 3.721465242739084189, -79.74999999999997158, 11.44722502806610365 ) ) ;
#53113=CIRCLE ( 'NONE', #19112, 14.00000000000000000 ) ;
#53120=EDGE_LOOP ( 'NONE', ( #34314, #26436, #24741, #43775 ) ) ;
#53123=SURFACE_STYLE_FILL_AREA ( #4405 ) ;
#53127=CARTESIAN_POINT ( 'NONE',  ( 2.563364080296999692, -77.04950204046299689, 12.08374998559000169 ) ) ;
#53136=CARTESIAN_POINT ( 'NONE',  ( 9.070694317316998934, -78.05004794253746070, 6.598531290616000078 ) ) ;
#53138=CARTESIAN_POINT ( 'NONE',  ( 9.453938376997999882, -79.19690445950300273, 6.036651369377000087 ) ) ;
#53145=CARTESIAN_POINT ( 'NONE',  ( 12.00000000000000000, -77.14999999999999147, 0.000000000000000000 ) ) ;
#53162=CARTESIAN_POINT ( 'NONE',  ( 10.46934363224000109, -77.35649902168898961, 5.823135730235999397 ) ) ;
#53165=CARTESIAN_POINT ( 'NONE',  ( 9.599999999999999645, -87.29999999999999716, 0.000000000000000000 ) ) ;
#53172=CARTESIAN_POINT ( 'NONE',  ( 11.99606675118999810, -79.59347606058199176, 2.584336171721000497 ) ) ;
#53179=CARTESIAN_POINT ( 'NONE',  ( 4.655405164384999850, -76.66483267504600008, -11.35230195258999863 ) ) ;
#53184=CARTESIAN_POINT ( 'NONE',  ( 11.03163745116999905, -78.39163123734599026, 0.06858965353743999571 ) ) ;
#53193=CARTESIAN_POINT ( 'NONE',  ( -4.187998665200000303, -78.72928582732099301, 11.54367560014000205 ) ) ;
#53197=CARTESIAN_POINT ( 'NONE',  ( -9.393203674808288994, -78.45833333333331439, 5.413904038987134015 ) ) ;
#53198=ORIENTED_EDGE ( 'NONE', *, *, #1839, .T. ) ;
#53204=CARTESIAN_POINT ( 'NONE',  ( -10.68161435044807561, -81.00000000000001421, -1.590318374505752974 ) ) ;
#53209=CARTESIAN_POINT ( 'NONE',  ( -8.982117338527000783, -79.71499958499398986, 6.718606902359000266 ) ) ;
#53211=ORIENTED_EDGE ( 'NONE', *, *, #55070, .F. ) ;
#53212=ORIENTED_EDGE ( 'NONE', *, *, #28903, .F. ) ;
#53226=FACE_OUTER_BOUND ( 'NONE', #23798, .T. ) ;
#53228=CARTESIAN_POINT ( 'NONE',  ( -8.148905501844000199, -78.76715395315800095, -8.781309899900000104 ) ) ;
#53231=DIRECTION ( 'NONE',  ( 0.000000000000000000, 1.000000000000000000, 0.000000000000000000 ) ) ;
#53235=CARTESIAN_POINT ( 'NONE',  ( 1.514497777301999859, -77.68767547371999171, 11.15976079676000055 ) ) ;
#53237=CARTESIAN_POINT ( 'NONE',  ( -1.715212302772999742, -80.93623568429859461, -11.12438410773000186 ) ) ;
#53243=CARTESIAN_POINT ( 'NONE',  ( -9.457500717944000712, -78.24349181547098908, -6.031068363571000290 ) ) ;
#53249=CARTESIAN_POINT ( 'NONE',  ( 0.000000000000000000, -87.59999999999999432, 0.000000000000000000 ) ) ;
#53252=CARTESIAN_POINT ( 'NONE',  ( -3.527598694514999966, -78.37623792800799549, -10.69532371905999923 ) ) ;
#53255=AXIS2_PLACEMENT_3D ( 'NONE', #34560, #7423, #12993 ) ;
#53258=CARTESIAN_POINT ( 'NONE',  ( -12.09999999997999964, -92.79999999999999716, -2.688213410018000232E-10 ) ) ;
#53259=CARTESIAN_POINT ( 'NONE',  ( -5.945647593938746311, -80.17843449223505559, -8.956060015876818881 ) ) ;
#53260=CARTESIAN_POINT ( 'NONE',  ( -9.393203674808267678, -77.04166666666665719, -5.413904038987171319 ) ) ;
#53262=EDGE_CURVE ( 'NONE', #1042, #5144, #53558, .T. ) ;
#53268=CARTESIAN_POINT ( 'NONE',  ( 7.942219812765999087, -79.63612155000399184, 7.984679643171000762 ) ) ;
#53269=CARTESIAN_POINT ( 'NONE',  ( 10.75000000000000000, -77.35000000000000853, 0.000000000000000000 ) ) ;
#53278=CARTESIAN_POINT ( 'NONE',  ( 10.63911585229000067, -78.84139468996799849, 2.446340097336999975 ) ) ;
#53297=VECTOR ( 'NONE', #46688, 1000.000000000000114 ) ;
#53298=CARTESIAN_POINT ( 'NONE',  ( 7.570062472618999116, -76.71279439517699927, -7.820779103414999156 ) ) ;
#53302=DIRECTION ( 'NONE',  ( 0.000000000000000000, -1.000000000000000000, 0.000000000000000000 ) ) ;
#53306=CARTESIAN_POINT ( 'NONE',  ( -7.960542989054001595, -80.83912993679970782, 7.971132368775000643 ) ) ;
#53309=ORIENTED_EDGE ( 'NONE', *, *, #14386, .T. ) ;
#53321=CARTESIAN_POINT ( 'NONE',  ( -11.68767212001978706, -78.92083333333333428, -3.140974612311364655 ) ) ;
#53324=CARTESIAN_POINT ( 'NONE',  ( -1.215378159391584223, -79.98441448756166494, 10.68123553570516293 ) ) ;
#53326=ORIENTED_EDGE ( 'NONE', *, *, #54435, .F. ) ;
#53327=CARTESIAN_POINT ( 'NONE',  ( 5.810395355999260936, -77.27055076788118981, -9.061764198440011242 ) ) ;
#53350=DIRECTION ( 'NONE',  ( 0.000000000000000000, -1.000000000000000000, 0.000000000000000000 ) ) ;
#53352=CARTESIAN_POINT ( 'NONE',  ( -9.599999999999999645, -87.29999999999999716, 0.000000000000000000 ) ) ;
#53353=CARTESIAN_POINT ( 'NONE',  ( -1.708367912329182836, -80.96267845950610820, -11.07999331822880507 ) ) ;
#53360=CARTESIAN_POINT ( 'NONE',  ( -13.89999999994000035, -80.79999999994109317, -2.316526479204000061E-09 ) ) ;
#53364=CARTESIAN_POINT ( 'NONE',  ( -10.74970698200568897, -78.10629880980414441, -0.8321373431320605585 ) ) ;
#53370=CARTESIAN_POINT ( 'NONE',  ( -10.64055841416000092, -78.54452889900299795, -2.440058154124999934 ) ) ;
#53372=CARTESIAN_POINT ( 'NONE',  ( 8.042137835475001495, -77.25865908154399619, 9.127242153301999394 ) ) ;
#53376=CARTESIAN_POINT ( 'NONE',  ( -7.492394017799830941, -79.53652907763523672, 7.710241490960848765 ) ) ;
#53378=ORIENTED_EDGE ( 'NONE', *, *, #29617, .F. ) ;
#53381=CARTESIAN_POINT ( 'NONE',  ( 12.06518374142000027, -79.49911536532098921, -1.485411366123999821 ) ) ;
#53382=FACE_OUTER_BOUND ( 'NONE', #26188, .T. ) ;
#53399=DIRECTION ( 'NONE',  ( 0.000000000000000000, 1.000000000000000000, 0.000000000000000000 ) ) ;
#53406=CARTESIAN_POINT ( 'NONE',  ( 0.03269534938340999675, -76.06591632114400170, 11.81851555469000026 ) ) ;
#53407=CYLINDRICAL_SURFACE ( 'NONE', #23983, 12.00000000000000000 ) ;
#53422=CARTESIAN_POINT ( 'NONE',  ( 3.507155896972999898, -79.25137714550699286, 10.65448112794999957 ) ) ;
#53442=CARTESIAN_POINT ( 'NONE',  ( -6.206245474241998572, -79.67165790279912585, 9.343480492029000217 ) ) ;
#53443=CARTESIAN_POINT ( 'NONE',  ( 10.47020627418438643, -77.77083333333334281, 2.813789756862283387 ) ) ;
#53447=CYLINDRICAL_SURFACE ( 'NONE', #47439, 10.75000000000000000 ) ;
#53448=CARTESIAN_POINT ( 'NONE',  ( -5.261498566940000288, -77.58713293807399225, -10.76255997729999869 ) ) ;
#53451=CARTESIAN_POINT ( 'NONE',  ( 6.420671964385999964, -77.74679431087899673, -10.06034164291999922 ) ) ;
#53463=CARTESIAN_POINT ( 'NONE',  ( 10.34070037867000202, -78.05223280600100111, -4.346035695907999319 ) ) ;
#53466=CARTESIAN_POINT ( 'NONE',  ( -1.041600863181999959, -76.62709993674098996, -12.22549076760999931 ) ) ;
#53469=ORIENTED_EDGE ( 'NONE', *, *, #26612, .F. ) ;
#53472=CARTESIAN_POINT ( 'NONE',  ( -6.220196401501000061, -78.71846735336799838, -9.111031286755999048 ) ) ;
#53475=CONICAL_SURFACE ( 'NONE', #8204, 9.649999999844000698, 0.7853981633972997312 ) ;
#53481=CARTESIAN_POINT ( 'NONE',  ( -12.26242965668000018, -78.32234609596400787, 0.6546740380507000134 ) ) ;
#53484=CARTESIAN_POINT ( 'NONE',  ( 10.75000000000000000, -78.25000000000000000, 1.005550720961999908E-14 ) ) ;
#53497=CARTESIAN_POINT ( 'NONE',  ( -1.639962962630000076, -78.58499365464699338, 11.09633417262999977 ) ) ;
#53512=DIRECTION ( 'NONE',  ( 0.000000000000000000, -0.7071067811866525998, -0.7071067811864425456 ) ) ;
#53516=CARTESIAN_POINT ( 'NONE',  ( -0.4732869866705000095, -79.06307788497599631, -12.30780274174999889 ) ) ;
#53518=CARTESIAN_POINT ( 'NONE',  ( -4.118243260437115971, -78.00630453228950500, 9.929863582829632662 ) ) ;
#53519=CARTESIAN_POINT ( 'NONE',  ( 3.925078296951999501, -78.48233087649200002, 11.31856107452000160 ) ) ;
#53528=CARTESIAN_POINT ( 'NONE',  ( 11.24465069584000076, -78.06898427574600419, -0.6259355293341001270 ) ) ;
#53530=CARTESIAN_POINT ( 'NONE',  ( -9.248645349825999062, -80.77514956827684500, 6.415315719250000548 ) ) ;
#53542=EDGE_CURVE ( 'NONE', #22144, #23718, #4936, .T. ) ;
#53549=CARTESIAN_POINT ( 'NONE',  ( -5.883052656872999719, -77.69532935296300025, 9.603314844095001135 ) ) ;
#53555=CARTESIAN_POINT ( 'NONE',  ( 3.733146969192831843, -80.25324884369585732, -10.08725862556905994 ) ) ;
#53556=CARTESIAN_POINT ( 'NONE',  ( 10.47020627418439531, -77.22916666666667140, -2.813789756862242974 ) ) ;
#53558=B_SPLINE_CURVE_WITH_KNOTS ( 'NONE', 3,
 ( #46116, #18943, #31620, #32783, #41664, #32204, #36935, #1529, #19233, #18362, #37225, #55240, #54948, #19524, #50245, #37517, #54383, #22781, #49663, #10374, #13920, #27191, #41083, #23652, #31913, #49957, #14499, #45232, #9501, #383, #27487 ),
 .UNSPECIFIED., .F., .F.,
 ( 4, 1, 1, 1, 1, 1, 1, 1, 1, 1, 1, 1, 1, 1, 1, 1, 1, 1, 1, 1, 1, 1, 1, 1, 1, 1, 1, 1, 4 ),
 ( 0.000000000000000000, 0.01436125421998360463, 0.05169932518655311754, 0.08903739615315010847, 0.1263754671197221124, 0.1637135380862941303, 0.2010516090528911004, 0.2383896800194630905, 0.2757277509860102116, 0.3130658219525572772, 0.3504038929191043428, 0.3877419638859008200, 0.4250800348524479966, 0.4624181058189950622, 0.4997561767855421277, 0.5370942477520891378, 0.5744323187186362034, 0.6117703896851832690, 0.6491084606517303346, 0.6864465316185268673, 0.7237846025850739329, 0.7611226735516209985, 0.7984607445181682861, 0.8357988154847151296, 0.8731368864512621952, 0.9104749574178092608, 0.9478130283846057935, 0.9851510993511529701, 1.000000000000000000 ),
 .UNSPECIFIED. ) ;
#53561=CARTESIAN_POINT ( 'NONE',  ( 2.026540639977999714, -80.03068473043869346, -10.96119216345999803 ) ) ;
#53563=ORIENTED_EDGE ( 'NONE', *, *, #22640, .F. ) ;
#53569=VERTEX_POINT ( 'NONE', #50696 ) ;
#53571=CONICAL_SURFACE ( 'NONE', #26203, 9.649999999844000698, 0.7853981633972997312 ) ;
#53573=CARTESIAN_POINT ( 'NONE',  ( -10.53927088184999938, -79.61726667242798783, 3.259678459687000096 ) ) ;
#53590=CARTESIAN_POINT ( 'NONE',  ( 4.772733260105000319, -76.68771245318799856, -9.782200613967999558 ) ) ;
#53599=CARTESIAN_POINT ( 'NONE',  ( -9.578166812159000898, -80.35756696074160743, 5.930253639820000089 ) ) ;
#53603=CARTESIAN_POINT ( 'NONE',  ( -9.393203674808274783, -80.04166666666664298, -5.413904038987162437 ) ) ;
#53604=EDGE_CURVE ( 'NONE', #9803, #39177, #21862, .T. ) ;
#53624=CARTESIAN_POINT ( 'NONE',  ( 5.363150622483991548, -77.26670457031288208, -9.329320527232589200 ) ) ;
#53634=CARTESIAN_POINT ( 'NONE',  ( 7.897520336252998874, -77.37301250442499168, -9.100831677656000096 ) ) ;
#53635=EDGE_LOOP ( 'NONE', ( #57696, #51048, #34990, #47500 ) ) ;
#53639=CARTESIAN_POINT ( 'NONE',  ( 3.140974612311327796, -78.65416666666665435, 11.68767212001979594 ) ) ;
#53652=CARTESIAN_POINT ( 'NONE',  ( -7.167604382869162905, -77.57604025214112653, 9.599037027053000770 ) ) ;
#53663=DIRECTION ( 'NONE',  ( 0.000000000000000000, 1.000000000000000000, 0.000000000000000000 ) ) ;
#53671=CARTESIAN_POINT ( 'NONE',  ( 10.89235442234000040, -77.78191129495199618, 0.7293703643125000191 ) ) ;
#53672=CARTESIAN_POINT ( 'NONE',  ( -4.187998665200000303, -78.27610463408198882, 11.54367560014000205 ) ) ;
#53675=CARTESIAN_POINT ( 'NONE',  ( -10.75000000000000000, -79.00000000000000000, 0.000000000000000000 ) ) ;
#53683=CARTESIAN_POINT ( 'NONE',  ( -11.23721025937000029, -79.15059218971499888, -3.995116809576999994 ) ) ;
#53684=CARTESIAN_POINT ( 'NONE',  ( 6.760020157659999640, -80.81784931869341904, -8.895273066339001389 ) ) ;
#53687=CARTESIAN_POINT ( 'NONE',  ( -10.17713110909000029, -76.79936102791799613, 4.716330562529999604 ) ) ;
#53692=CARTESIAN_POINT ( 'NONE',  ( 3.630949683904999947, -79.79999999999999716, -11.17491406647000041 ) ) ;
#53699=CARTESIAN_POINT ( 'NONE',  ( -11.05000000000000071, -81.00000000000000000, 0.000000000000000000 ) ) ;
#53704=LINE ( 'NONE', #58121, #2895 ) ;
#53706=FACE_OUTER_BOUND ( 'NONE', #21213, .T. ) ;
#53715=CARTESIAN_POINT ( 'NONE',  ( -7.621235760192000441, -76.69489580791500316, -9.570988338631000403 ) ) ;
#53724=CARTESIAN_POINT ( 'NONE',  ( 9.869466656387999137, -76.96059422246487713, -5.330266269891000164 ) ) ;
#53727=CARTESIAN_POINT ( 'NONE',  ( 11.14115696400000033, -79.14243177349999314, -1.301050381412999890 ) ) ;
#53734=VECTOR ( 'NONE', #24221, 1000.000000000000000 ) ;
#53739=CARTESIAN_POINT ( 'NONE',  ( 11.13784153760999907, -76.48629006631499294, 5.174080857020999957 ) ) ;
#53745=DIRECTION ( 'NONE',  ( 1.776356839400000238E-14, -1.000000000000000000, 8.733754460384000171E-14 ) ) ;
#53751=CARTESIAN_POINT ( 'NONE',  ( 2.228685126279000173, -77.85842609231200129, 11.77068507108999995 ) ) ;
#53753=CARTESIAN_POINT ( 'NONE',  ( 8.241770352740999783, -78.26225130393000029, -8.631843597936001089 ) ) ;
#53757=CARTESIAN_POINT ( 'NONE',  ( 6.043427764450807871, -78.46666666666665435, -10.48543666025108934 ) ) ;
#53758=CARTESIAN_POINT ( 'NONE',  ( -10.90697944550000109, -80.02995714425549068, -0.4616983494901999996 ) ) ;
#53762=EDGE_CURVE ( 'NONE', #31986, #20195, #29320, .T. ) ;
#53769=CARTESIAN_POINT ( 'NONE',  ( 3.184503561814999717, -76.36297076860699917, 11.84932461738999976 ) ) ;
#53771=CARTESIAN_POINT ( 'NONE',  ( 0.6694192215519998435, -76.87011569981827108, 10.80149589243966446 ) ) ;
#53773=CARTESIAN_POINT ( 'NONE',  ( 10.53539001158999966, -79.99784788827008697, -3.979889026714000355 ) ) ;
#53782=CARTESIAN_POINT ( 'NONE',  ( -8.353021825866999706, -78.89206171986300831, -9.001266886329000627 ) ) ;
#53784=CARTESIAN_POINT ( 'NONE',  ( -13.89999999999999858, -80.79999999999999716, 0.000000000000000000 ) ) ;
#53787=CARTESIAN_POINT ( 'NONE',  ( 12.00000000000000000, -77.04999999999999716, 0.000000000000000000 ) ) ;
#53789=VERTEX_POINT ( 'NONE', #23079 ) ;
#53790=CARTESIAN_POINT ( 'NONE',  ( 10.24965171066401126, -78.82574021499290495, -3.245740100043394527 ) ) ;
#53796=CARTESIAN_POINT ( 'NONE',  ( -3.455491054688999863, -78.24078379918199744, -10.47670062235000010 ) ) ;
#53800=CARTESIAN_POINT ( 'NONE',  ( -0.4146318973827000098, -79.32037491569599297, -11.20920117498000046 ) ) ;
#53816=VERTEX_POINT ( 'NONE', #41386 ) ;
#53817=CARTESIAN_POINT ( 'NONE',  ( -5.635457317866999105, -79.02831925412799308, -10.95206051398000113 ) ) ;
#53819=CARTESIAN_POINT ( 'NONE',  ( -8.439750306821999004, -76.58265968624300513, 7.626226795102000189 ) ) ;
#53820=CARTESIAN_POINT ( 'NONE',  ( -5.334928932963716619, -78.01642494921711091, 9.332864396458077749 ) ) ;
#53821=CARTESIAN_POINT ( 'NONE',  ( 7.483561698776000526, -78.45520156106799448, 9.354804580292000793 ) ) ;
#53823=AXIS2_PLACEMENT_3D ( 'NONE', #14076, #53350, #35620 ) ;
#53828=CARTESIAN_POINT ( 'NONE',  ( 9.807952262865001103, -77.10173030608999056, -5.297043796141999827 ) ) ;
#53834=B_SPLINE_CURVE_WITH_KNOTS ( 'NONE', 3,
 ( #54624, #26557, #44587, #31868, #57871, #27733, #35716, #13281, #32158, #4143, #50197, #45777, #18318, #21848, #17424, #35411, #53442, #49315, #12984, #4438, #22438, #36013, #54038, #13577, #31568, #19771, #32446, #41912, #51663, #6181, #15625, #10626, #14738, #37182, #54900, #24193, #10044, #2067, #33619, #32737, #56079, #38056, #46654, #6473, #1776, #11211, #914, #1197, #19476, #29189, #28025, #5314, #42210, #51078, #28608, #37767, #55788, #33032, #15338, #14451, #24484, #46070, #5592, #37469, #10330 ),
 .UNSPECIFIED., .F., .F.,
 ( 4, 1, 1, 1, 1, 1, 1, 1, 1, 1, 1, 1, 1, 1, 1, 1, 1, 1, 1, 1, 1, 1, 1, 1, 1, 1, 1, 1, 1, 1, 1, 1, 1, 1, 1, 1, 1, 1, 1, 1, 1, 1, 1, 1, 1, 1, 1, 1, 1, 1, 1, 1, 1, 1, 1, 1, 1, 1, 1, 1, 1, 1, 4 ),
 ( 0.000000000000000000, 0.01249977652363855676, 0.02874978397245062101, 0.04499979142126268872, 0.06124979887007475643, 0.07749980631888682414, 0.09374981376769889185, 0.1099998212165109596, 0.1262498286653230273, 0.1424998361141350811, 0.1587498435629471627, 0.1749998510117592165, 0.1912498584605712981, 0.2074998659093833520, 0.2237498733581954335, 0.2399998808070074596, 0.2562498882558195135, 0.2724998957046316228, 0.2887499031534436766, 0.3049999106022557305, 0.3212499180510677843, 0.3374999254998798937, 0.3537499329486919475, 0.3699999403975040013, 0.3862499478463160552, 0.4024999552951281645, 0.4187499627439402183, 0.4349999701927522722, 0.4512499776415643260, 0.4674999850903764353, 0.4837499925391884892, 0.4999999999880005430, 0.5162500074368124858, 0.5325000148856245952, 0.5487500223344365935, 0.5650000297832487028, 0.5812500372320608122, 0.5975000446808729215, 0.6137500521296849199, 0.6300000595784970292, 0.6462500670273090275, 0.6625000744761211369, 0.6787500819249331352, 0.6950000893737452445, 0.7112500968225573539, 0.7275001042713694632, 0.7437501117201814615, 0.7600001191689935709, 0.7762501266178055692, 0.7925001340666176786, 0.8087501415154296769, 0.8250001489642417862, 0.8412501564130538956, 0.8575001638618660049, 0.8737501713106780032, 0.8900001787594901126, 0.9062501862083021109, 0.9225001936571142203, 0.9387502011059262186, 0.9550002085547383279, 0.9712502160035503262, 0.9875002234523625466, 1.000000000000000000 ),
 .UNSPECIFIED. ) ;
#53850=CARTESIAN_POINT ( 'NONE',  ( 10.94776161156000072, -76.97393005650599207, 2.097883759165000139 ) ) ;
#53856=CARTESIAN_POINT ( 'NONE',  ( -2.075652906230024630, -80.20975560462747467, -10.54757134404949781 ) ) ;
#53862=CARTESIAN_POINT ( 'NONE',  ( -1.769784341028000085, -80.00344838743689024, -11.00556513567000039 ) ) ;
#53875=CARTESIAN_POINT ( 'NONE',  ( 10.71899861749000138, -79.37213958541198622, -2.608601736514999825 ) ) ;
#53894=CARTESIAN_POINT ( 'NONE',  ( -9.673449916064999599, -76.98869575705799662, 4.989449158498000081 ) ) ;
#53903=CARTESIAN_POINT ( 'NONE',  ( 9.755626371838998168, -81.11000911083239373, -5.633583086437000453 ) ) ;
#53930=CARTESIAN_POINT ( 'NONE',  ( -5.191308461407881047, -77.18497258547503748, -9.414107671153617574 ) ) ;
#53931=CARTESIAN_POINT ( 'NONE',  ( 8.012523733906443013, -79.11708638852500997, 8.990154430766320814 ) ) ;
#53934=CARTESIAN_POINT ( 'NONE',  ( 7.520016693046000178, -79.88042186404709355, -9.389162645085001202 ) ) ;
#53939=CARTESIAN_POINT ( 'NONE',  ( 9.505630310840999186, -77.88846949747699000, -7.405319984134000499 ) ) ;
#53943=EDGE_CURVE ( 'NONE', #10829, #24242, #9576, .T. ) ;
#53965=CARTESIAN_POINT ( 'NONE',  ( 0.000000000000000000, -82.09999999999999432, 0.000000000000000000 ) ) ;
#53973=CARTESIAN_POINT ( 'NONE',  ( 10.01578477942999967, -77.80914763795398414, 4.342743515613999961 ) ) ;
#53974=CARTESIAN_POINT ( 'NONE',  ( -1.381217146163000065, -77.55708155120599656, -12.08613957309999876 ) ) ;
#53975=CARTESIAN_POINT ( 'NONE',  ( 0.000000000000000000, -80.89999999999999147, 0.000000000000000000 ) ) ;
#53982=CARTESIAN_POINT ( 'NONE',  ( -1.615886945735000024, -81.02768543471519536, 11.05491664572000232 ) ) ;
#53983=FACE_OUTER_BOUND ( 'NONE', #10386, .T. ) ;
#53985=CARTESIAN_POINT ( 'NONE',  ( 7.155101792066000499, -78.58303919030899465, -8.354909834651998324 ) ) ;
#54004=ORIENTED_EDGE ( 'NONE', *, *, #1941, .F. ) ;
#54010=EDGE_LOOP ( 'NONE', ( #17853, #17254, #27573, #2697 ) ) ;
#54011=CARTESIAN_POINT ( 'NONE',  ( -12.34758422210000184, -76.18886453605900044, 0.3526192563760000009 ) ) ;
#54012=CARTESIAN_POINT ( 'NONE',  ( -9.952579048958215324, -78.63104145445697668, -4.074197893549214911 ) ) ;
#54018=CARTESIAN_POINT ( 'NONE',  ( -8.729704736440837110, -77.69597548351386251, 7.043462628994999974 ) ) ;
#54033=CARTESIAN_POINT ( 'NONE',  ( 1.298131932841000147, -76.56825554292399261, 12.21218573294999921 ) ) ;
#54038=CARTESIAN_POINT ( 'NONE',  ( 11.15679540746000065, -79.50823984478810758, 1.159321710118000004 ) ) ;
#54040=B_SPLINE_SURFACE_WITH_KNOTS ( 'NONE', 3, 3, ( 
 ( #18314, #36305, #22730, #18607, #49906, #40448, #9740, #14446, #23021, #624, #18891, #27728, #45772, #32441, #26551, #54329, #31267, #4137, #22135, #58156, #17723, #54033, #35710, #53739, #49309, #49612, #44882, #22433, #39, #18015, #40741, #36007, #31864, #13573, #31564 ),
 ( #45182, #13870, #37464, #10622, #37763, #38339, #38053, #55191, #56076, #20065, #33324, #10326, #55784, #56363, #19766, #15334, #1772, #28603, #2064, #29186, #20344, #42785, #51361, #10037, #15033, #10917, #28306, #28897, #46357, #50486, #46944, #47234, #6469, #14732, #33616 ),
 ( #24480, #51074, #24187, #5881, #42495, #15621, #28020, #23889, #1481, #46065, #51660, #33028, #11208, #41908, #5587, #6762, #15913, #19471, #24772, #46650, #42205, #23600, #2349, #41612, #19183, #1193, #6177, #50781, #37178, #32732, #55485, #29470, #25054, #25627, #33898 ),
 ( #12062, #3485, #44222, #52504, #30042, #34184, #57792, #3771, #3209, #21199, #56650, #2637, #7626, #38916, #2915, #34473, #51941, #20913, #48374, #56934, #43650, #39200, #48095, #43936, #16783, #7339, #21491, #21774, #52790, #34764, #8202, #39497, #57501, #17063, #39778 ) ),
 .UNSPECIFIED., .F., .F., .F.,
 ( 4, 4 ),
 ( 4, 1, 1, 1, 1, 1, 1, 1, 1, 1, 1, 1, 1, 1, 1, 1, 1, 1, 1, 1, 1, 1, 1, 1, 1, 1, 1, 1, 1, 1, 1, 1, 4 ),
 ( -0.5168282991434000051, 1.516828299142999992 ),
 ( -0.01510644027126000107, 0.009441525169539000117, 0.03398949061033999797, 0.05853745605114000355, 0.08308542149195000115, 0.1076333869326999981, 0.1321813523735999862, 0.1567293178143999988, 0.1812772832552000113, 0.2058252486960000238, 0.2303732141367999808, 0.2549211795776000211, 0.2794691450183999781, 0.3040171104591999907, 0.3285650759000000032, 0.3531130413408000157, 0.3776610067816000282, 0.4022089722223999853, 0.4267569376631999978, 0.4513049031039999548, 0.4758528685447999673, 0.5004008339856000909, 0.5249487994264000479, 0.5494967648672000049, 0.5740447303079999619, 0.5985926957488000300, 0.6231406611895999870, 0.6476886266303999440, 0.6722365920712000120, 0.6967845575119999690, 0.7213325229527999261, 0.7458804883935999941, 0.7704284538343999511 ),
 .UNSPECIFIED. ) ;
#54053=CARTESIAN_POINT ( 'NONE',  ( 10.60715898610999908, -79.75759371423698951, -2.581384170113000032 ) ) ;
#54062=EDGE_CURVE ( 'NONE', #14498, #26643, #10980, .T. ) ;
#54063=CARTESIAN_POINT ( 'NONE',  ( 12.00000000000000000, -77.66041666666669130, 1.570796326794922093 ) ) ;
#54065=CARTESIAN_POINT ( 'NONE',  ( -4.249989987144469517, -76.90707437668547186, 9.952789594769198445 ) ) ;
#54067=CARTESIAN_POINT ( 'NONE',  ( -1.788059198778999770, -79.88890251626278882, -11.11920900327000084 ) ) ;
#54077=CARTESIAN_POINT ( 'NONE',  ( -6.606377239730371720, -78.42708333333332860, 8.596418555780411808 ) ) ;
#54080=ORIENTED_EDGE ( 'NONE', *, *, #8627, .F. ) ;
#54085=VERTEX_POINT ( 'NONE', #20406 ) ;
#54087=CARTESIAN_POINT ( 'NONE',  ( -8.507210620304000770, -77.69605693914598987, -7.023467935662000450 ) ) ;
#54093=CARTESIAN_POINT ( 'NONE',  ( 11.15679540746000065, -79.45655663070499486, 1.159321710118000004 ) ) ;
#54110=CARTESIAN_POINT ( 'NONE',  ( -2.550058755020000234, -79.48197165242800111, -12.16911022628999994 ) ) ;
#54111=CARTESIAN_POINT ( 'NONE',  ( 6.067686772785999771, -75.97136531054800912, 9.621429083000000659 ) ) ;
#54112=CARTESIAN_POINT ( 'NONE',  ( -7.708860374575333907, -78.03865554921938497, 7.492616441312939912 ) ) ;
#54113=CARTESIAN_POINT ( 'NONE',  ( -6.777984382448000389, -78.21103772225399098, -9.878005474088999094 ) ) ;
#54117=CARTESIAN_POINT ( 'NONE',  ( 2.661146832675047147, -80.95524119419135900, 10.42413934193408309 ) ) ;
#54120=CARTESIAN_POINT ( 'NONE',  ( -8.675294248904002359, -77.83711156713900436, 6.999562148147999707 ) ) ;
#54122=CARTESIAN_POINT ( 'NONE',  ( -3.046770093036999860, -80.56158377905549628, -10.59643116276000008 ) ) ;
#54127=CARTESIAN_POINT ( 'NONE',  ( 10.79417609527999922, -77.42640152541599718, -3.050225076229999832 ) ) ;
#54138=CARTESIAN_POINT ( 'NONE',  ( 10.80251317621999974, -78.04940181198600158, 3.184285419974999698 ) ) ;
#54146=CARTESIAN_POINT ( 'NONE',  ( 8.596418555780450887, -77.19791666666668561, -6.606377239730321982 ) ) ;
#54148=ORIENTED_EDGE ( 'NONE', *, *, #16607, .T. ) ;
#54151=CARTESIAN_POINT ( 'NONE',  ( 9.395013887366999938, -79.18635809738199782, 5.999026139886999509 ) ) ;
#54158=CIRCLE ( 'NONE', #26773, 1.499999999999999556 ) ;
#54175=CARTESIAN_POINT ( 'NONE',  ( -7.223234266881706667, -76.97379502737749135, -9.635782272404652460 ) ) ;
#54180=CARTESIAN_POINT ( 'NONE',  ( 11.09875712452000052, -76.16149361465799927, 1.375294608629999971 ) ) ;
#54183=CARTESIAN_POINT ( 'NONE',  ( -10.70541732380000077, -76.51213885926499358, 1.965825919828999790 ) ) ;
#54185=DIRECTION ( 'NONE',  ( 1.000000000000000000, 0.000000000000000000, 0.000000000000000000 ) ) ;
#54187=CARTESIAN_POINT ( 'NONE',  ( -7.960542989054001595, -80.77134138352347748, 7.971132368775000643 ) ) ;
#54188=CARTESIAN_POINT ( 'NONE',  ( 10.48543666025108401, -76.59166666666665435, 6.043427764450814976 ) ) ;
#54193=CARTESIAN_POINT ( 'NONE',  ( 8.828526701892000617, -80.59834844877070736, -6.997593314318000246 ) ) ;
#54219=CARTESIAN_POINT ( 'NONE',  ( 7.162480479084130991, -77.28307999974209963, -8.040150979671629727 ) ) ;
#54227=CARTESIAN_POINT ( 'NONE',  ( -12.03258451680999919, -78.18689196713800982, 0.6424029262030001020 ) ) ;
#54230=ORIENTED_EDGE ( 'NONE', *, *, #57145, .T. ) ;
#54247=CARTESIAN_POINT ( 'NONE',  ( -5.261498566940001176, -77.73881614468353973, -10.76255997729999869 ) ) ;
#54250=CARTESIAN_POINT ( 'NONE',  ( 4.275783788279646558, -77.00602939643633249, -10.37011484984485676 ) ) ;
#54257=CARTESIAN_POINT ( 'NONE',  ( 2.801992291048324812, -76.27265625000197247, 11.67810493544244999 ) ) ;
#54267=DIRECTION ( 'NONE',  ( 0.000000000000000000, -0.1961161351384349827, -0.9805806756908699295 ) ) ;
#54269=CARTESIAN_POINT ( 'NONE',  ( -10.66734455299000039, -77.50954786493399240, 2.320156498608999751 ) ) ;
#54271=CARTESIAN_POINT ( 'NONE',  ( -10.75000000000000000, -76.50000000000000000, 0.000000000000000000 ) ) ;
#54278=CARTESIAN_POINT ( 'NONE',  ( 0.2367807722781999913, -79.49682939073299792, 11.92391661984999907 ) ) ;
#54279=VECTOR ( 'NONE', #41869, 1000.000000000000114 ) ;
#54280=CARTESIAN_POINT ( 'NONE',  ( 11.04613657998999976, -80.82006762628775220, -0.4641449021664000307 ) ) ;
#54305=PRESENTATION_STYLE_ASSIGNMENT (( #48700 ) ) ;
#54308=CARTESIAN_POINT ( 'NONE',  ( -12.01364710452999951, -77.17245025537799563, 2.874040219260999951 ) ) ;
#54315=CARTESIAN_POINT ( 'NONE',  ( 7.374560639698993114, -78.97708333333332575, -9.596002108778149520 ) ) ;
#54329=CARTESIAN_POINT ( 'NONE',  ( -1.925872869407999843, -76.81415197275400430, -12.12904120624999926 ) ) ;
#54340=CARTESIAN_POINT ( 'NONE',  ( -1.835125225091999823, -77.88555540773499786, 11.83842809849000055 ) ) ;
#54342=CARTESIAN_POINT ( 'NONE',  ( 7.455335830631999450, -78.39789788104899060, 9.319520915745998835 ) ) ;
#54347=CARTESIAN_POINT ( 'NONE',  ( -7.210617325615999995, -79.59417565622599966, -8.196484842528999337 ) ) ;
#54351=ADVANCED_FACE ( 'NONE', ( #2906 ), #15906, .F. ) ;
#54355=CARTESIAN_POINT ( 'NONE',  ( 6.043427764450763462, -77.73333333333330586, 10.48543666025111065 ) ) ;
#54359=CARTESIAN_POINT ( 'NONE',  ( -6.231249681807000229, -79.69824811525000996, 9.381124237602000093 ) ) ;
#54361=CARTESIAN_POINT ( 'NONE',  ( -5.413904038987206846, -79.91666666666665719, 9.393203674808249914 ) ) ;
#54367=CARTESIAN_POINT ( 'NONE',  ( 2.251292830498444086, -76.35833333333332007, 10.57172952794451959 ) ) ;
#54378=ORIENTED_EDGE ( 'NONE', *, *, #35821, .F. ) ;
#54379=CARTESIAN_POINT ( 'NONE',  ( 10.75000000000000000, -78.85000000000000853, 0.000000000000000000 ) ) ;
#54380=CARTESIAN_POINT ( 'NONE',  ( -2.787231282280638656, -77.70418860435997033, -10.40622658089639607 ) ) ;
#54381=CONICAL_SURFACE ( 'NONE', #57190, 9.649999999909001147, 0.7853981633972997312 ) ;
#54383=CARTESIAN_POINT ( 'NONE',  ( -1.963210506780999953, -76.36095766513311389, -11.00998129987999974 ) ) ;
#54388=CARTESIAN_POINT ( 'NONE',  ( 11.21665020278000036, -78.51660049291498922, 0.06973997782872000395 ) ) ;
#54390=VERTEX_POINT ( 'NONE', #34757 ) ;
#54395=CYLINDRICAL_SURFACE ( 'NONE', #17793, 11.05000000000000071 ) ;
#54398=CARTESIAN_POINT ( 'NONE',  ( -12.00000000000000000, -78.39999999999999147, 0.000000000000000000 ) ) ;
#54405=EDGE_LOOP ( 'NONE', ( #17744, #45746, #41751, #33578 ) ) ;
#54406=CARTESIAN_POINT ( 'NONE',  ( -5.660024744116999962, -78.92225316430300097, 10.80800494192000016 ) ) ;
#54407=CARTESIAN_POINT ( 'NONE',  ( -4.602886058546999948, -76.30107567883000286, -10.53195524498000069 ) ) ;
#54408=CARTESIAN_POINT ( 'NONE',  ( -6.498065648774645986, -78.02678715505997786, 8.565420681610083520 ) ) ;
#54409=CARTESIAN_POINT ( 'NONE',  ( 11.70594025892000012, -78.40094293021999761, 2.546964289010999583 ) ) ;
#54411=AXIS2_PLACEMENT_3D ( 'NONE', #21131, #21426, #16426 ) ;
#54412=LINE ( 'NONE', #9241, #9915 ) ;
#54415=CARTESIAN_POINT ( 'NONE',  ( 7.367079209569801002, -80.91505000046390705, 7.831813084430341299 ) ) ;
#54418=CARTESIAN_POINT ( 'NONE',  ( 0.5439554104848000060, -77.02002127708399826, -11.13367472273999859 ) ) ;
#54419=CARTESIAN_POINT ( 'NONE',  ( -9.596002108778193929, -78.24791666666664014, 7.374560639698935383 ) ) ;
#54420=CARTESIAN_POINT ( 'NONE',  ( -5.285748055207999840, -80.37364997703009806, 9.676158635172999567 ) ) ;
#54427=CARTESIAN_POINT ( 'NONE',  ( 9.668944085725000193, -76.99062003738698934, 5.685915129398999568 ) ) ;
#54431=CARTESIAN_POINT ( 'NONE',  ( -10.75000000000000000, -78.50000000000000000, 0.000000000000000000 ) ) ;
#54435=EDGE_CURVE ( 'NONE', #19148, #4693, #8195, .T. ) ;
#54438=CARTESIAN_POINT ( 'NONE',  ( 7.461283454533999659, -76.89222102750099452, -8.281536679888001018 ) ) ;
#54445=CARTESIAN_POINT ( 'NONE',  ( 10.75000000000000000, -77.25000000000000000, 0.000000000000000000 ) ) ;
#54446=CARTESIAN_POINT ( 'NONE',  ( 8.645788266876911266, -78.65487569970177617, 7.146464437358057253 ) ) ;
#54448=PLANE ( 'NONE',  #41619 ) ;
#54450=CARTESIAN_POINT ( 'NONE',  ( -2.830810333559000025, -78.99570369636998635, -10.78151721355999904 ) ) ;
#54452=ORIENTED_EDGE ( 'NONE', *, *, #25141, .T. ) ;
#54457=ORIENTED_EDGE ( 'NONE', *, *, #52837, .F. ) ;
#54463=CARTESIAN_POINT ( 'NONE',  ( -10.75000000000000000, -78.01041666666665719, -1.407171709420429018 ) ) ;
#54469=CIRCLE ( 'NONE', #28864, 14.00000000000000000 ) ;
#54481=CARTESIAN_POINT ( 'NONE',  ( -10.34138800174999950, -80.80143906952710608, 4.468208825537999473 ) ) ;
#54487=CARTESIAN_POINT ( 'NONE',  ( 5.620590082324000036, -80.56825076276699349, -9.763102121971000358 ) ) ;
#54490=ORIENTED_EDGE ( 'NONE', *, *, #19452, .F. ) ;
#54497=CARTESIAN_POINT ( 'NONE',  ( -2.598793908247287732, -79.49442965258924687, 10.43132793576024220 ) ) ;
#54505=B_SPLINE_CURVE_WITH_KNOTS ( 'NONE', 3,
 ( #17884, #21999, #5176, #36749, #32303, #22295, #40006, #8426, #58022, #58321 ),
 .UNSPECIFIED., .F., .F.,
 ( 4, 2, 2, 2, 4 ),
 ( 0.000000000000000000, 0.2499999999999998335, 0.4999999999999998890, 0.7499999999999998890, 1.000000000000000000 ),
 .UNSPECIFIED. ) ;
#54513=ORIENTED_EDGE ( 'NONE', *, *, #1839, .F. ) ;
#54514=CARTESIAN_POINT ( 'NONE',  ( -4.625569715417624295, -77.18961895380674321, -9.703952514631545512 ) ) ;
#54515=CARTESIAN_POINT ( 'NONE',  ( 11.87139580924463012, -79.06341727770498551, 2.023209039049198577 ) ) ;
#54524=CARTESIAN_POINT ( 'NONE',  ( 10.48586718643000104, -77.40014181984899722, -5.936521791247999502 ) ) ;
#54528=CARTESIAN_POINT ( 'NONE',  ( 1.570796326794857478, -78.66458333333331154, 12.00000000000000533 ) ) ;
#54537=CARTESIAN_POINT ( 'NONE',  ( -10.85772169724999969, -76.75329282578898926, 1.763485056683000041 ) ) ;
#54564=CARTESIAN_POINT ( 'NONE',  ( -12.22643784615999962, -77.38083722509800566, -1.144550905343000080 ) ) ;
#54571=CARTESIAN_POINT ( 'NONE',  ( 6.273262642061999905, -80.40039539424418535, 9.103776903494001260 ) ) ;
#54575=CARTESIAN_POINT ( 'NONE',  ( 9.869466656387999137, -77.04448811493399774, -5.330266269891000164 ) ) ;
#54580=CARTESIAN_POINT ( 'NONE',  ( 5.522795323340943696, -76.07083333333035569, 9.558450660443439162 ) ) ;
#54582=DIRECTION ( 'NONE',  ( -1.000000000000000000, 0.000000000000000000, 0.000000000000000000 ) ) ;
#54592=ORIENTED_EDGE ( 'NONE', *, *, #47173, .T. ) ;
#54601=ORIENTED_EDGE ( 'NONE', *, *, #42905, .T. ) ;
#54615=AXIS2_PLACEMENT_3D ( 'NONE', #3411, #30256, #43566 ) ;
#54624=CARTESIAN_POINT ( 'NONE',  ( 6.586108526242999694, -80.07391735373440156, 8.810401493720998900 ) ) ;
#54629=CARTESIAN_POINT ( 'NONE',  ( 7.919842512018000491, -77.31583978383599742, 8.988445846368000147 ) ) ;
#54633=CARTESIAN_POINT ( 'NONE',  ( -4.109499447189000065, -78.41155876290798687, 11.32730267836999971 ) ) ;
#54636=CARTESIAN_POINT ( 'NONE',  ( 10.35105862822000056, -80.30232057427369341, 3.468557695829999954 ) ) ;
#54643=CARTESIAN_POINT ( 'NONE',  ( -7.845158543477998236, -76.94443866757499961, -9.736889158655001708 ) ) ;
#54648=CARTESIAN_POINT ( 'NONE',  ( 10.52346617262000095, -78.43212195875699422, -3.675769182893000142 ) ) ;
#54650=CARTESIAN_POINT ( 'NONE',  ( 6.724037440004856592, -79.72330751359039880, -9.661915242757062927 ) ) ;
#54662=CARTESIAN_POINT ( 'NONE',  ( 9.800312463269442276, -78.81625363457253286, -4.431906745122180524 ) ) ;
#54666=CIRCLE ( 'NONE', #24492, 11.05000000000000071 ) ;
#54670=CARTESIAN_POINT ( 'NONE',  ( 6.233047529871999615, -78.88050366622999832, 9.960502923565000444 ) ) ;
#54671=CARTESIAN_POINT ( 'NONE',  ( -0.2721098858049000313, -79.14303638195599433, 11.21356619464000026 ) ) ;
#54672=CARTESIAN_POINT ( 'NONE',  ( -2.527424140845015543, -80.99999999999998579, 10.49288982607049192 ) ) ;
#54675=ORIENTED_EDGE ( 'NONE', *, *, #6993, .F. ) ;
#54681=CARTESIAN_POINT ( 'NONE',  ( 9.596002108778174389, -78.59791666666667709, -7.374560639698961140 ) ) ;
#54690=CARTESIAN_POINT ( 'NONE',  ( -12.03384906095000062, -78.92404336158600131, 2.625351077966999735 ) ) ;
#54691=CARTESIAN_POINT ( 'NONE',  ( 6.130995657900000673, -76.03909237496100104, 9.721816919625998921 ) ) ;
#54692=CARTESIAN_POINT ( 'NONE',  ( 8.547764506834246490, -77.90230234131951192, 6.557723838816148287 ) ) ;
#54699=CARTESIAN_POINT ( 'NONE',  ( -3.455491054688999863, -78.55851086359500357, -10.47670062235000010 ) ) ;
#54700=CARTESIAN_POINT ( 'NONE',  ( 5.137083998358000336, -77.31100733245999379, -10.56753840748999984 ) ) ;
#54701=CARTESIAN_POINT ( 'NONE',  ( -10.62901853172999900, -80.93745138310640641, 2.931062299181000252 ) ) ;
#54705=CARTESIAN_POINT ( 'NONE',  ( -8.649885944100999424, -77.75323764143800531, -7.141259254888000285 ) ) ;
#54717=CARTESIAN_POINT ( 'NONE',  ( 3.911191660715999774, -77.12336614992500472, 10.56108632439999973 ) ) ;
#54720=CARTESIAN_POINT ( 'NONE',  ( 12.00000000000000000, -77.54999999999999716, 0.000000000000000000 ) ) ;
#54723=CARTESIAN_POINT ( 'NONE',  ( -7.443611313279832054, -80.16459463203885605, -7.755757990568101334 ) ) ;
#54727=DIRECTION ( 'NONE',  ( 0.000000000000000000, -1.000000000000000000, 0.000000000000000000 ) ) ;
#54728=CARTESIAN_POINT ( 'NONE',  ( 11.14495853502000067, -80.13963010244600582, -0.2109943715695999922 ) ) ;
#54761=CARTESIAN_POINT ( 'NONE',  ( 7.496935112050000072, -80.65095063950900567, 8.408636027568000770 ) ) ;
#54766=PLANE ( 'NONE',  #15815 ) ;
#54778=CARTESIAN_POINT ( 'NONE',  ( -8.941925947373027483, -79.55322172220051868, 5.966891831842909610 ) ) ;
#54800=CARTESIAN_POINT ( 'NONE',  ( 11.90415444617999974, -79.94018912574220792, -1.731350929957999885 ) ) ;
#54803=EDGE_LOOP ( 'NONE', ( #33448, #42804 ) ) ;
#54804=CARTESIAN_POINT ( 'NONE',  ( -11.80948866808000020, -78.67521964476598839, 2.394107155543000243 ) ) ;
#54809=CARTESIAN_POINT ( 'NONE',  ( -5.318190277593210169, -76.48798860270505884, -10.78586198116576256 ) ) ;
#54813=CIRCLE ( 'NONE', #15237, 11.70000000000000107 ) ;
#54815=CARTESIAN_POINT ( 'NONE',  ( -10.47020627418439354, -80.52083333333331439, -2.813789756862263847 ) ) ;
#54819=CARTESIAN_POINT ( 'NONE',  ( -10.99972769911000015, -76.18386543273099676, 2.019869862886000345 ) ) ;
#54833=FACE_OUTER_BOUND ( 'NONE', #21890, .T. ) ;
#54834=CARTESIAN_POINT ( 'NONE',  ( -10.75000000000000000, -79.51041666666668561, -1.407171709420429018 ) ) ;
#54849=CARTESIAN_POINT ( 'NONE',  ( -4.459146134027999864, -80.11617729102648866, 10.37101146982000088 ) ) ;
#54851=FACE_OUTER_BOUND ( 'NONE', #41800, .T. ) ;
#54852=CARTESIAN_POINT ( 'NONE',  ( 9.144378690012999300, -77.53474228896699572, -6.496033325431000094 ) ) ;
#54857=CARTESIAN_POINT ( 'NONE',  ( -9.490437400528026757, -76.14895833332546715, 5.483493355980267658 ) ) ;
#54858=EDGE_CURVE ( 'NONE', #16988, #21964, #4591, .T. ) ;
#54867=CARTESIAN_POINT ( 'NONE',  ( 1.675539995062999887, -79.19048418952499446, 11.92720225554999836 ) ) ;
#54871=EDGE_CURVE ( 'NONE', #31838, #10296, #50971, .T. ) ;
#54875=ORIENTED_EDGE ( 'NONE', *, *, #38273, .F. ) ;
#54900=CARTESIAN_POINT ( 'NONE',  ( -7.301194973305000779, -79.18140372876651156, 8.515319286630999684 ) ) ;
#54903=FACE_OUTER_BOUND ( 'NONE', #40032, .T. ) ;
#54910=CARTESIAN_POINT ( 'NONE',  ( 4.441925970415999458, -77.42124252579399979, 11.07721969470000190 ) ) ;
#54913=CARTESIAN_POINT ( 'NONE',  ( 2.343379474233999726, -80.38402960327920255, 10.44606179296999926 ) ) ;
#54919=CARTESIAN_POINT ( 'NONE',  ( -10.86848958346127247, -76.18151041669857193, -1.423534178637803960 ) ) ;
#54921=CARTESIAN_POINT ( 'NONE',  ( -5.327124403004999564, -75.96338747164598715, -11.31261546482999947 ) ) ;
#54926=CARTESIAN_POINT ( 'NONE',  ( -2.830810333559000025, -78.81343076078299248, -10.78151721355999904 ) ) ;
#54929=CARTESIAN_POINT ( 'NONE',  ( -10.75000000000000000, -80.00000000000000000, 0.000000000000000000 ) ) ;
#54933=DIRECTION ( 'NONE',  ( 1.000000000000000000, 0.000000000000000000, 0.000000000000000000 ) ) ;
#54945=CARTESIAN_POINT ( 'NONE',  ( 6.822280249786099482, -78.77980337427507607, -8.307691429770278191 ) ) ;
#54948=CARTESIAN_POINT ( 'NONE',  ( 9.886069181790999139, -76.46128543308955727, -5.228720670581999741 ) ) ;
#54951=CARTESIAN_POINT ( 'NONE',  ( 3.166308453645628074, -76.40348697233208952, 11.78162183767860682 ) ) ;
#54952=CARTESIAN_POINT ( 'NONE',  ( 11.20814727018469981, -77.82862452491039562, 4.230534968287241959 ) ) ;
#54953=CARTESIAN_POINT ( 'NONE',  ( -4.152600241220000044, -79.36092712597098853, -10.41988588363999924 ) ) ;
#54955=VERTEX_POINT ( 'NONE', #3321 ) ;
#54975=CARTESIAN_POINT ( 'NONE',  ( 6.043427764450807871, -79.56666666666666288, -10.48543666025108756 ) ) ;
#54976=CARTESIAN_POINT ( 'NONE',  ( -3.290092089285999499, -76.67444993108999540, 11.13683286123999849 ) ) ;
#54979=CARTESIAN_POINT ( 'NONE',  ( -11.96278216175999987, -78.06186122270700878, 0.6386762756999999624 ) ) ;
#54984=CARTESIAN_POINT ( 'NONE',  ( 4.081313924463877640, -80.94422573434229662, 9.944984660275112631 ) ) ;
#54987=CARTESIAN_POINT ( 'NONE',  ( -11.05562587724999979, -77.40133007910999652, -1.423986317748999975 ) ) ;
#54989=CARTESIAN_POINT ( 'NONE',  ( -8.190711764258001182, -80.40049766303370404, 7.381016022845000357 ) ) ;
#54993=CARTESIAN_POINT ( 'NONE',  ( 0.5473670387515998659, -76.82720197937599949, -11.20350390113000039 ) ) ;
#55009=CARTESIAN_POINT ( 'NONE',  ( -1.570796326794885012, -79.41458333333333997, -12.00000000000000178 ) ) ;
#55012=CARTESIAN_POINT ( 'NONE',  ( -10.31421052434999908, -76.72175206120299151, 3.823226550887000030 ) ) ;
#55017=ADVANCED_FACE ( 'NONE', ( #52909 ), #3037, .F. ) ;
#55020=CARTESIAN_POINT ( 'NONE',  ( -10.22609403765000025, -79.98946642284438724, -4.138687607718999573 ) ) ;
#55022=ORIENTED_EDGE ( 'NONE', *, *, #44348, .T. ) ;
#55030=CARTESIAN_POINT ( 'NONE',  ( -10.25000000000000000, -87.20000000000000284, 0.000000000000000000 ) ) ;
#55037=CARTESIAN_POINT ( 'NONE',  ( 0.000000000000000000, -79.79999999999999716, 0.000000000000000000 ) ) ;
#55049=CARTESIAN_POINT ( 'NONE',  ( -5.059370734576000395, -80.85404126026540439, -10.06538451635999998 ) ) ;
#55050=CARTESIAN_POINT ( 'NONE',  ( -7.374560639699022424, -76.72708333333333997, 9.596002108778135309 ) ) ;
#55066=CARTESIAN_POINT ( 'NONE',  ( -0.9930572065396647830, -79.48254699571987203, 10.70474299318766853 ) ) ;
#55070=EDGE_CURVE ( 'NONE', #55197, #40109, #37968, .T. ) ;
#55087=CARTESIAN_POINT ( 'NONE',  ( 7.652056849482000267, -79.52181829387700418, 9.281873293285000770 ) ) ;
#55093=ORIENTED_EDGE ( 'NONE', *, *, #43595, .F. ) ;
#55106=CARTESIAN_POINT ( 'NONE',  ( -5.051502324002999760E-14, -80.79999999999999716, 0.000000000000000000 ) ) ;
#55108=CARTESIAN_POINT ( 'NONE',  ( -9.831705185582000794, -76.15878349074199605, 5.330239850318999828 ) ) ;
#55110=AXIS2_PLACEMENT_3D ( 'NONE', #10628, #46364, #19478 ) ;
#55131=CARTESIAN_POINT ( 'NONE',  ( 9.687205842286999768, -77.57074243306399808, -7.546775612817000045 ) ) ;
#55136=ORIENTED_EDGE ( 'NONE', *, *, #19452, .T. ) ;
#55138=CARTESIAN_POINT ( 'NONE',  ( 8.646305450917001423, -80.01125923301559340, 6.688629566474999955 ) ) ;
#55141=CARTESIAN_POINT ( 'NONE',  ( 9.869466656387999137, -77.11227666821000071, -5.330266269891000164 ) ) ;
#55146=CARTESIAN_POINT ( 'NONE',  ( 10.93439773960121641, -81.00000000000000000, -1.422938603756783049 ) ) ;
#55147=VERTEX_POINT ( 'NONE', #36925 ) ;
#55150=CARTESIAN_POINT ( 'NONE',  ( -10.34138800174999950, -80.66586196297468803, 4.468208825537999473 ) ) ;
#55151=FACE_OUTER_BOUND ( 'NONE', #48900, .T. ) ;
#55159=CARTESIAN_POINT ( 'NONE',  ( -1.381217146163000065, -77.87480861561799372, -12.08613957309999876 ) ) ;
#55163=B_SPLINE_CURVE_WITH_KNOTS ( 'NONE', 3,
 ( #27208, #10102, #23380, #41390, #973, #18957 ),
 .UNSPECIFIED., .F., .F.,
 ( 4, 2, 4 ),
 ( 0.000000000000000000, 0.5000000000000001110, 1.000000000000000000 ),
 .UNSPECIFIED. ) ;
#55175=CARTESIAN_POINT ( 'NONE',  ( 10.46888361534042566, -80.82922105002511159, -2.813437968995440741 ) ) ;
#55186=CARTESIAN_POINT ( 'NONE',  ( -5.413904038987160661, -77.58333333333332860, -9.393203674808278336 ) ) ;
#55191=CARTESIAN_POINT ( 'NONE',  ( -8.987350104473000201, -77.07422532591699849, 8.369597699504998545 ) ) ;
#55197=VERTEX_POINT ( 'NONE', #45518 ) ;
#55203=CARTESIAN_POINT ( 'NONE',  ( -8.524893907337000698, -77.63827704918399775, -8.352346156331998728 ) ) ;
#55213=CARTESIAN_POINT ( 'NONE',  ( -6.713100897100000353, -76.79350771435500178, 10.54932473490999989 ) ) ;
#55218=CARTESIAN_POINT ( 'NONE',  ( 7.840078887343000069, -78.96286685420099616, -8.084993976410000727 ) ) ;
#55229=CARTESIAN_POINT ( 'NONE',  ( 1.407171709420391936, -79.36458333333331439, 10.75000000000000178 ) ) ;
#55238=CARTESIAN_POINT ( 'NONE',  ( 6.023077783880060210, -78.77250036845040881, -8.904115691191277548 ) ) ;
#55240=CARTESIAN_POINT ( 'NONE',  ( 11.01994305158000209, -76.48636737507854377, -1.906499110313000234 ) ) ;
#55247=CARTESIAN_POINT ( 'NONE',  ( -6.778077112046531738, -78.12704699457141544, -9.878140615074055830 ) ) ;
#55248=CARTESIAN_POINT ( 'NONE',  ( 4.782478426736999744, -79.60605421298700435, 10.14623135401999932 ) ) ;
#55264=ORIENTED_EDGE ( 'NONE', *, *, #1014, .F. ) ;
#55265=CARTESIAN_POINT ( 'NONE',  ( 3.140974612311376646, -79.54583333333333428, -11.68767212001978706 ) ) ;
#55267=CARTESIAN_POINT ( 'NONE',  ( 5.679944191426311129, -77.93085335426356153, 9.133896504759128732 ) ) ;
#55268=CARTESIAN_POINT ( 'NONE',  ( 6.917788961650999546, -78.74009410830100819, -9.780606322222999083 ) ) ;
#55274=CARTESIAN_POINT ( 'NONE',  ( 10.44390837562477969, -80.86943310474272550, 2.545984649820042023 ) ) ;
#55275=CARTESIAN_POINT ( 'NONE',  ( 0.000000000000000000, -92.13603921945998820, 0.000000000000000000 ) ) ;
#55277=CARTESIAN_POINT ( 'NONE',  ( -10.98551332331999930, -76.95156662648800250, 1.010146990136999934 ) ) ;
#55278=CARTESIAN_POINT ( 'NONE',  ( -9.801255020792000394, -76.59853460670321113, 7.399866681860999940 ) ) ;
#55279=CARTESIAN_POINT ( 'NONE',  ( 5.459723135333999444, -80.22537985460630239, 9.711247138783999588 ) ) ;
#55284=CARTESIAN_POINT ( 'NONE',  ( -11.12496554189999998, -77.27629933467800072, -1.432917402686000097 ) ) ;
#55286=CARTESIAN_POINT ( 'NONE',  ( 6.536160117426359051, -80.22377045582020116, 8.743586084475110098 ) ) ;
#55288=CARTESIAN_POINT ( 'NONE',  ( -9.238576773750232007, -78.54311845634511258, -5.559101997765075964 ) ) ;
#55300=CARTESIAN_POINT ( 'NONE',  ( 0.000000000000000000, -76.29999999999999716, 0.000000000000000000 ) ) ;
#55304=CARTESIAN_POINT ( 'NONE',  ( -10.72781790777320765, -80.10681046886573142, -0.8882985175872072370 ) ) ;
#55309=CARTESIAN_POINT ( 'NONE',  ( 3.315825420378000210, -79.60815762081898583, -10.52174111842000137 ) ) ;
#55312=ADVANCED_FACE ( 'NONE', ( #38670 ), #19871, .T. ) ;
#55313=ORIENTED_EDGE ( 'NONE', *, *, #48488, .T. ) ;
#55328=CARTESIAN_POINT ( 'NONE',  ( -9.404538367151713985, -76.95366911081998751, -7.521839627126676753 ) ) ;
#55333=EDGE_CURVE ( 'NONE', #3745, #30361, #34226, .T. ) ;
#55337=CARTESIAN_POINT ( 'NONE',  ( -5.508096857961803927, -77.38721230508248539, -10.70907476296403793 ) ) ;
#55343=CARTESIAN_POINT ( 'NONE',  ( 8.828526701892000617, -80.46277134221820404, -6.997593314318000246 ) ) ;
#55345=CARTESIAN_POINT ( 'NONE',  ( -5.413682991573638859, -76.68346113739394809, -9.392790915597688084 ) ) ;
#55347=EDGE_CURVE ( 'NONE', #31098, #353, #26656, .T. ) ;
#55361=CARTESIAN_POINT ( 'NONE',  ( 9.898445906460613841, -79.38214623308790863, 4.225145221008577145 ) ) ;
#55376=ORIENTED_EDGE ( 'NONE', *, *, #18928, .F. ) ;
#55377=CARTESIAN_POINT ( 'NONE',  ( -6.309004353333000026, -79.21496069382000371, -10.24224633278999796 ) ) ;
#55382=CARTESIAN_POINT ( 'NONE',  ( 11.83900414546000057, -78.36332874153899297, -1.507807444711000144 ) ) ;
#55386=VERTEX_POINT ( 'NONE', #28647 ) ;
#55394=CARTESIAN_POINT ( 'NONE',  ( 10.75000000000000355, -80.73958333333332860, -1.407171709420407035 ) ) ;
#55396=CARTESIAN_POINT ( 'NONE',  ( -7.679961486493839473, -79.79999999999998295, -9.071626512970588863 ) ) ;
#55401=CARTESIAN_POINT ( 'NONE',  ( -1.963210506780999953, -76.30927514267598610, -11.00998129987999974 ) ) ;
#55413=CARTESIAN_POINT ( 'NONE',  ( -10.24862125074130859, -78.07571521542081427, 3.248992843890492033 ) ) ;
#55418=CARTESIAN_POINT ( 'NONE',  ( -10.07979664880000037, -76.97175206120299151, 3.736335038366999761 ) ) ;
#55429=CARTESIAN_POINT ( 'NONE',  ( 8.118221194901000359, -77.19093201713099006, 9.213591238522999660 ) ) ;
#55437=CARTESIAN_POINT ( 'NONE',  ( 7.587302191891999392, -79.95518973060389101, 7.873108652756999781 ) ) ;
#55441=CARTESIAN_POINT ( 'NONE',  ( -11.12496554189999998, -77.41187644123000666, -1.432917402686000097 ) ) ;
#55449=CARTESIAN_POINT ( 'NONE',  ( -4.454457568640999732, -80.60566659096738817, 10.34731867136000005 ) ) ;
#55455=CARTESIAN_POINT ( 'NONE',  ( 8.048377923311001325, -77.50846663325098973, -9.274674788995000085 ) ) ;
#55462=CARTESIAN_POINT ( 'NONE',  ( -7.374560639699022424, -79.72708333333335418, 9.596002108778135309 ) ) ;
#55468=CARTESIAN_POINT ( 'NONE',  ( 10.75068688215930379, -80.83963933037178151, -1.406941906430807521 ) ) ;
#55470=DIRECTION ( 'NONE',  ( 0.000000000000000000, -0.7071067811866525998, -0.7071067811864425456 ) ) ;
#55475=CARTESIAN_POINT ( 'NONE',  ( -12.00000000000000178, -78.81041666666666856, -1.570796326794897890 ) ) ;
#55485=CARTESIAN_POINT ( 'NONE',  ( -12.27595451887999900, -76.06383379162799940, 0.3505736730271999391 ) ) ;
#55490=CYLINDRICAL_SURFACE ( 'NONE', #24791, 10.75000000000000000 ) ;
#55497=CARTESIAN_POINT ( 'NONE',  ( -0.7974440169908999509, -78.62859328629799904, -12.02330465019000094 ) ) ;
#55503=CARTESIAN_POINT ( 'NONE',  ( 7.599690325503999588, -79.21286685420099616, -7.837095951096998192 ) ) ;
#55516=CARTESIAN_POINT ( 'NONE',  ( -8.075863243196769403, -76.41068158389745690, -7.736832730023080806 ) ) ;
#55517=CARTESIAN_POINT ( 'NONE',  ( 7.833999859145873934, -79.73288990288156697, -8.785953829483144517 ) ) ;
#55521=CARTESIAN_POINT ( 'NONE',  ( -5.269052519453173211, -78.76382107170879010, 9.902459013403186461 ) ) ;
#55532=CARTESIAN_POINT ( 'NONE',  ( 8.747355858532181117, -78.80079676788167831, -6.250980141072946417 ) ) ;
#55538=CARTESIAN_POINT ( 'NONE',  ( -9.663535141866287148, -76.10162506589206544, -7.446444224017321645 ) ) ;
#55539=CARTESIAN_POINT ( 'NONE',  ( 3.249543687795219959, -78.69676261847072851, -11.53084807003014056 ) ) ;
#55540=CARTESIAN_POINT ( 'NONE',  ( 6.766402264611000028, -79.44263615497600028, -8.946167390840999545 ) ) ;
#55543=ORIENTED_EDGE ( 'NONE', *, *, #42332, .F. ) ;
#55550=CARTESIAN_POINT ( 'NONE',  ( 3.140974612311376646, -78.54583333333332007, -11.68767212001978706 ) ) ;
#55562=CARTESIAN_POINT ( 'NONE',  ( 10.45296947248102803, -77.86878944864642449, 2.509422360510712213 ) ) ;
#55563=CARTESIAN_POINT ( 'NONE',  ( 11.70594025892000012, -78.33315437694399463, 2.546964289010999583 ) ) ;
#55571=CARTESIAN_POINT ( 'NONE',  ( -9.833855776131001036, -77.49629348652399585, -4.999701486664000605 ) ) ;
#55580=CARTESIAN_POINT ( 'NONE',  ( 2.854969924326999919, -78.12062596773400003, 10.84745395576000071 ) ) ;
#55582=CARTESIAN_POINT ( 'NONE',  ( 6.436424241555000592, -80.32391735373440156, 8.610165096135999008 ) ) ;
#55590=CARTESIAN_POINT ( 'NONE',  ( 10.33259770149999923, -77.55914763795398414, 4.480110411294999651 ) ) ;
#55594=CARTESIAN_POINT ( 'NONE',  ( -12.00000000000000355, -77.78958333333331154, 1.570796326794848596 ) ) ;
#55598=ORIENTED_EDGE ( 'NONE', *, *, #11996, .F. ) ;
#55605=CARTESIAN_POINT ( 'NONE',  ( -9.575027280576000166, -79.41750321980599381, 5.479104576271000226 ) ) ;
#55624=CARTESIAN_POINT ( 'NONE',  ( 11.00000000000000000, -76.04999999999999716, -1.235097113410999977E-09 ) ) ;
#55638=CARTESIAN_POINT ( 'NONE',  ( 1.548297770046941357, -76.13463541594487083, -11.83463544049746652 ) ) ;
#55639=CIRCLE ( 'NONE', #21661, 11.70000000000000107 ) ;
#55655=CARTESIAN_POINT ( 'NONE',  ( 10.34395135506634311, -79.37222233871651156, 2.957440531220869140 ) ) ;
#55667=CARTESIAN_POINT ( 'NONE',  ( 7.601957635810941305, -80.28750185634191894, -7.600825067425311055 ) ) ;
#55670=PRODUCT_DEFINITION ( 'UNKNOWN', '', #24436, #25680 ) ;
#55673=CARTESIAN_POINT ( 'NONE',  ( -11.22206352833000054, -79.66321515653298491, -4.332716936452000844 ) ) ;
#55677=CARTESIAN_POINT ( 'NONE',  ( -1.828203654226000063, -78.01064764102999050, 11.79377691179999843 ) ) ;
#55678=ORIENTED_EDGE ( 'NONE', *, *, #31687, .T. ) ;
#55682=CARTESIAN_POINT ( 'NONE',  ( 10.47020627418438643, -78.77083333333334281, 2.813789756862283387 ) ) ;
#55697=CARTESIAN_POINT ( 'NONE',  ( 3.089703999423501379, -78.54774383309995756, -10.47025070535708835 ) ) ;
#55698=CARTESIAN_POINT ( 'NONE',  ( 7.486068761172999686, -75.88288212886199346, -8.059700645992000645 ) ) ;
#55702=CARTESIAN_POINT ( 'NONE',  ( 11.06434106074000034, -76.55977708591699127, -1.914180163160999815 ) ) ;
#55705=AXIS2_PLACEMENT_3D ( 'NONE', #11605, #4097, #48207 ) ;
#55707=B_SPLINE_CURVE_WITH_KNOTS ( 'NONE', 3,
 ( #49409, #26942, #4531, #17219 ),
 .UNSPECIFIED., .F., .F.,
 ( 4, 4 ),
 ( 0.000000000000000000, 1.000000000000000000 ),
 .UNSPECIFIED. ) ;
#55713=CARTESIAN_POINT ( 'NONE',  ( -10.76103485090999889, -79.54790851955898745, -5.748848539142999314 ) ) ;
#55714=CARTESIAN_POINT ( 'NONE',  ( -9.129079589776326387, -78.05585660196875608, 5.676768158082784232 ) ) ;
#55735=CARTESIAN_POINT ( 'NONE',  ( 10.40890440584000132, -80.99049444111729201, 4.369998498427999145 ) ) ;
#55738=CARTESIAN_POINT ( 'NONE',  ( 9.668944085725000193, -77.19398569721599301, 5.685915129398999568 ) ) ;
#55744=ORIENTED_EDGE ( 'NONE', *, *, #7707, .F. ) ;
#55746=CARTESIAN_POINT ( 'NONE',  ( -5.059370734576000395, -80.78625270698918825, -10.06538451635999998 ) ) ;
#55753=CARTESIAN_POINT ( 'NONE',  ( 6.321312781113044288, -78.78005093995929542, 10.10155803323563894 ) ) ;
#55756=CARTESIAN_POINT ( 'NONE',  ( -10.77989530031999976, -78.79720534002599663, -5.637054895855999170 ) ) ;
#55758=CARTESIAN_POINT ( 'NONE',  ( 9.298780387958270666, -78.70743112811207709, -5.515246406192360062 ) ) ;
#55763=CARTESIAN_POINT ( 'NONE',  ( -10.75007815099182551, -77.61041948879531560, -1.407065427747188568 ) ) ;
#55767=CARTESIAN_POINT ( 'NONE',  ( -8.824204240651999598, -78.62350394595299008, -6.427191105727000142 ) ) ;
#55769=CARTESIAN_POINT ( 'NONE',  ( 7.103614071024587417, -80.78233878846501170, -8.098765007180103837 ) ) ;
#55784=CARTESIAN_POINT ( 'NONE',  ( 12.07535958108000074, -76.86931163439298587, -2.237927141218000404 ) ) ;
#55788=CARTESIAN_POINT ( 'NONE',  ( 5.745747329289001115, -78.58220418272651386, 9.633509135241000720 ) ) ;
#55789=AXIS2_PLACEMENT_3D ( 'NONE', #44406, #54727, #26675 ) ;
#55796=CARTESIAN_POINT ( 'NONE',  ( 9.846943056836000352, -78.70998123256900669, -6.945033154232000072 ) ) ;
#55797=CARTESIAN_POINT ( 'NONE',  ( 0.000000000000000000, -87.70000000000000284, 0.000000000000000000 ) ) ;
#55801=CARTESIAN_POINT ( 'NONE',  ( -10.54473782110994584, -79.58454813932776517, 2.090270118525876075 ) ) ;
#55812=CARTESIAN_POINT ( 'NONE',  ( 2.325232682335999890, -78.41813999416500280, -11.01938817673000059 ) ) ;
#55813=CARTESIAN_POINT ( 'NONE',  ( 10.02302243881105248, -76.06467930920804577, -4.754755962258590429 ) ) ;
#55814=CARTESIAN_POINT ( 'NONE',  ( -7.104039980509410768, -78.97588114887535937, 9.465219502475884283 ) ) ;
#55819=B_SPLINE_CURVE_WITH_KNOTS ( 'NONE', 3,
 ( #38404, #31190, #44801, #4353 ),
 .UNSPECIFIED., .F., .F.,
 ( 4, 4 ),
 ( 0.000000000000000000, 1.000000000000000000 ),
 .UNSPECIFIED. ) ;
#55831=CARTESIAN_POINT ( 'NONE',  ( 8.956105305515906778, -78.80351547480260876, -5.945488880285457967 ) ) ;
#55839=CARTESIAN_POINT ( 'NONE',  ( 10.99434377831019560, -78.83240919558934934, 4.758605572679748263 ) ) ;
#55840=CARTESIAN_POINT ( 'NONE',  ( 8.554126827399000987, -80.09570377856319112, -7.255689219360999864 ) ) ;
#55847=CARTESIAN_POINT ( 'NONE',  ( 5.263204982374492857, -78.01377408750333586, -9.905568246058097159 ) ) ;
#55860=CARTESIAN_POINT ( 'NONE',  ( -9.517692138466999907, -76.32513885926499597, -6.653162853725000048 ) ) ;
#55861=CARTESIAN_POINT ( 'NONE',  ( -0.2771659042208530210, -77.97711776262842420, 10.74664504278661781 ) ) ;
#55862=CARTESIAN_POINT ( 'NONE',  ( 4.374544387491000386, -77.28864099784598807, -11.15253550093999912 ) ) ;
#55868=CARTESIAN_POINT ( 'NONE',  ( 10.45021209859945799, -80.86923990539705187, 2.519930479213339680 ) ) ;
#55870=CARTESIAN_POINT ( 'NONE',  ( -10.07979664880000037, -76.57175206120300004, 3.736335038366999761 ) ) ;
#55871=CARTESIAN_POINT ( 'NONE',  ( 8.993546968190999635, -77.65971154453498571, -6.388884668894999841 ) ) ;
#55872=CARTESIAN_POINT ( 'NONE',  ( 9.406806676749999596, -76.84443103653305229, -7.895227358184000899 ) ) ;
#55873=CARTESIAN_POINT ( 'NONE',  ( 0.6259563484655999988, -80.65615852947209419, -10.89273910470000040 ) ) ;
#55879=CARTESIAN_POINT ( 'NONE',  ( -3.513443458492000016, -78.43354160802699937, -10.65240647004999985 ) ) ;
#55883=CARTESIAN_POINT ( 'NONE',  ( -1.123220714122999953, -76.95895616928899585, 12.10057525372000065 ) ) ;
#55892=CARTESIAN_POINT ( 'NONE',  ( 10.48543666025108401, -77.59166666666668277, 6.043427764450814976 ) ) ;
#55894=VECTOR ( 'NONE', #12908, 1000.000000000000114 ) ;
#55902=CARTESIAN_POINT ( 'NONE',  ( -1.629741404508999958, -78.77781295235500636, 11.02717296151999982 ) ) ;
#55905=EDGE_LOOP ( 'NONE', ( #32856, #5211, #18482, #3258 ) ) ;
#55952=CARTESIAN_POINT ( 'NONE',  ( -2.002768801220407013, -79.48993535946543432, 10.56433384562239475 ) ) ;
#55963=CARTESIAN_POINT ( 'NONE',  ( 4.585445119925699586, -80.26028109100353447, -9.723566880156193193 ) ) ;
#55964=CARTESIAN_POINT ( 'NONE',  ( -7.100359491673154722, -77.16761677373057182, -8.072272176001158428 ) ) ;
#55965=CARTESIAN_POINT ( 'NONE',  ( 14.00000000000000000, -91.29999999999999716, -8.151435677387999117E-14 ) ) ;
#55968=CARTESIAN_POINT ( 'NONE',  ( 0.4713521909880000194, -79.00577527788799159, 12.02020425643999957 ) ) ;
#55974=CARTESIAN_POINT ( 'NONE',  ( -7.140570215937000143, -77.54944927882600325, 9.562832187120999805 ) ) ;
#55977=CARTESIAN_POINT ( 'NONE',  ( 2.813789756862229652, -78.85416666666665719, 10.47020627418440064 ) ) ;
#55978=ORIENTED_EDGE ( 'NONE', *, *, #50580, .F. ) ;
#55989=CARTESIAN_POINT ( 'NONE',  ( -5.413904038987160661, -80.58333333333332860, -9.393203674808278336 ) ) ;
#55992=AXIS2_PLACEMENT_3D ( 'NONE', #51371, #2075, #50203 ) ;
#55995=CARTESIAN_POINT ( 'NONE',  ( -1.963210506780999953, -76.51264080250500399, -11.00998129987999974 ) ) ;
#55996=CARTESIAN_POINT ( 'NONE',  ( 10.14846770183394931, -76.32381270956288688, -3.633859120905852613 ) ) ;
#55998=CARTESIAN_POINT ( 'NONE',  ( 1.857189518626999991, -76.68518679586200903, 11.07404950498000140 ) ) ;
#56005=CARTESIAN_POINT ( 'NONE',  ( 10.14252871893000041, -79.37232516803899784, 6.568753285854999291 ) ) ;
#56006=CARTESIAN_POINT ( 'NONE',  ( -10.10146701087682963, -78.07232890951112836, 3.678169913406422520 ) ) ;
#56025=CARTESIAN_POINT ( 'NONE',  ( -6.032763990770999563, -81.13038518513180009, 9.116036532382999269 ) ) ;
#56028=CARTESIAN_POINT ( 'NONE',  ( 4.275724345439000373, -77.05780398220699112, -10.36997068233999997 ) ) ;
#56045=CARTESIAN_POINT ( 'NONE',  ( 12.10970598371999962, -77.58985457952199738, 2.037349774713999917 ) ) ;
#56049=EDGE_LOOP ( 'NONE', ( #22637, #49392, #3365, #9360, #37673, #12746, #53211, #14639, #4279, #34603, #11555 ) ) ;
#56054=AXIS2_PLACEMENT_3D ( 'NONE', #19403, #37394, #14959 ) ;
#56058=CARTESIAN_POINT ( 'NONE',  ( 0.9322037676993999433, -78.70521297495899660, -10.87687281004000006 ) ) ;
#56063=DIRECTION ( 'NONE',  ( 0.000000000000000000, 0.000000000000000000, -1.000000000000000000 ) ) ;
#56076=CARTESIAN_POINT ( 'NONE',  ( -3.699256142337000064, -77.03324258761200838, 11.71059914860999918 ) ) ;
#56079=CARTESIAN_POINT ( 'NONE',  ( 10.93160348586000019, -79.01798567075552171, 2.513594203403000105 ) ) ;
#56087=CARTESIAN_POINT ( 'NONE',  ( 7.599120132820000428, -78.26244375222299254, 9.499258065358000991 ) ) ;
#56091=CARTESIAN_POINT ( 'NONE',  ( 3.413317904202999742, -79.37628491221198601, 10.36940822202999790 ) ) ;
#56102=CARTESIAN_POINT ( 'NONE',  ( -10.48543666025109289, -77.94166666666666288, -6.043427764450796325 ) ) ;
#56105=CARTESIAN_POINT ( 'NONE',  ( 11.09894631581144786, -76.10969828002846782, 1.375318052133717828 ) ) ;
#56106=CARTESIAN_POINT ( 'NONE',  ( 10.61587740312611494, -79.26335282761201029, -5.228565026272720573 ) ) ;
#56120=CARTESIAN_POINT ( 'NONE',  ( -12.24313050396999891, -77.30790438420399369, 2.928939827507999638 ) ) ;
#56121=CARTESIAN_POINT ( 'NONE',  ( -3.172678955510176202, -78.70149065425773927, -10.30724250848049017 ) ) ;
#56129=CARTESIAN_POINT ( 'NONE',  ( -5.394429334091999984, -79.98675840655589298, -9.834543342166998769 ) ) ;
#56137=CARTESIAN_POINT ( 'NONE',  ( 0.1392768204836610790, -77.22392014045128406, 11.21615847476518901 ) ) ;
#56138=UNCERTAINTY_MEASURE_WITH_UNIT (LENGTH_MEASURE( 1.000000000000000082E-05 ), #16650, 'distance_accuracy_value', 'NONE');
#56142=CARTESIAN_POINT ( 'NONE',  ( 10.75000000000000000, -80.75000000000000000, 3.489821576044999869E-14 ) ) ;
#56146=CARTESIAN_POINT ( 'NONE',  ( 9.785129497364000173, -79.35060081380299835, -6.997026981537000090 ) ) ;
#56150=CARTESIAN_POINT ( 'NONE',  ( -11.68767212001978706, -79.42083333333333428, -3.140974612311364655 ) ) ;
#56152=CARTESIAN_POINT ( 'NONE',  ( 10.20085796994174743, -79.32408745329188093, -3.463766342026746159 ) ) ;
#56153=CARTESIAN_POINT ( 'NONE',  ( 5.537129384246000541, -78.90287000084299507, 10.62336504503000079 ) ) ;
#56157=CARTESIAN_POINT ( 'NONE',  ( 8.169132698983039731, -80.90664037331559655, 6.987377867537430731 ) ) ;
#56160=CARTESIAN_POINT ( 'NONE',  ( -10.68734765800000019, -76.97880296949000467, -2.735374635455000369 ) ) ;
#56162=CARTESIAN_POINT ( 'NONE',  ( 2.000571476059000098, -81.16626456354109109, -10.72571703250999953 ) ) ;
#56164=ORIENTED_EDGE ( 'NONE', *, *, #6365, .F. ) ;
#56169=CARTESIAN_POINT ( 'NONE',  ( 11.19952915612999966, -78.01168059572700031, -0.6234238306063999424 ) ) ;
#56173=CARTESIAN_POINT ( 'NONE',  ( -12.25072062129000017, -77.00442731979100586, 0.6836512919489999840 ) ) ;
#56180=( GEOMETRIC_REPRESENTATION_CONTEXT ( 3 ) GLOBAL_UNCERTAINTY_ASSIGNED_CONTEXT ( ( #56138 ) ) GLOBAL_UNIT_ASSIGNED_CONTEXT ( ( #16650, #7787, #2498 ) ) REPRESENTATION_CONTEXT ( 'NONE', 'WORKASPACE' ) );
#56182=CARTESIAN_POINT ( 'NONE',  ( -11.68767212001979061, -76.82083333333335418, -3.140974612311365988 ) ) ;
#56183=CARTESIAN_POINT ( 'NONE',  ( 10.48543666025110710, -79.50833333333332575, -6.043427764450776785 ) ) ;
#56189=ORIENTED_EDGE ( 'NONE', *, *, #10602, .T. ) ;
#56196=EDGE_CURVE ( 'NONE', #7434, #2543, #50418, .T. ) ;
#56223=CARTESIAN_POINT ( 'NONE',  ( 9.596002108778145967, -77.20208333333333428, 7.374560639699002884 ) ) ;
#56244=CARTESIAN_POINT ( 'NONE',  ( -2.531359639385017068, -79.49391352960579127, 10.44770980819917838 ) ) ;
#56249=CARTESIAN_POINT ( 'NONE',  ( -9.367668485852000515, -77.09685739310599217, 5.826535979523000286 ) ) ;
#56255=CARTESIAN_POINT ( 'NONE',  ( 5.984702975412354853, -80.27245023178548422, -8.929714566242253682 ) ) ;
#56258=CARTESIAN_POINT ( 'NONE',  ( -11.60111135005000094, -79.22298198540099179, -3.181408645392000523 ) ) ;
#56262=CARTESIAN_POINT ( 'NONE',  ( 0.9591162783412999771, -78.25481147984399399, -11.89603288543000126 ) ) ;
#56264=ORIENTED_EDGE ( 'NONE', *, *, #563, .T. ) ;
#56272=ORIENTED_EDGE ( 'NONE', *, *, #30956, .F. ) ;
#56281=CARTESIAN_POINT ( 'NONE',  ( 0.2112907341303528197, -79.79999999999999716, -11.79160395029623487 ) ) ;
#56282=CARTESIAN_POINT ( 'NONE',  ( -7.115719518657461329, -80.03287302791015634, 8.059270059204177272 ) ) ;
#56285=CARTESIAN_POINT ( 'NONE',  ( -7.860507001410999450, -76.83870604836299378, 7.955276143908999842 ) ) ;
#56288=CARTESIAN_POINT ( 'NONE',  ( 9.824451308078000267, -76.60242220834099669, -5.196131110057000235 ) ) ;
#56290=CARTESIAN_POINT ( 'NONE',  ( 0.000000000000000000, -92.13603921945998820, 0.000000000000000000 ) ) ;
#56293=CARTESIAN_POINT ( 'NONE',  ( 8.621786563366999445, -78.88570433617398692, 7.917562470644999628 ) ) ;
#56294=CARTESIAN_POINT ( 'NONE',  ( 11.05131777856872688, -76.22578125001119531, 4.579357959789169819 ) ) ;
#56314=CARTESIAN_POINT ( 'NONE',  ( 5.194930721789999595, -80.11395898343219812, 10.15375755480999942 ) ) ;
#56319=DIRECTION ( 'NONE',  ( 0.000000000000000000, 1.000000000000000000, 0.000000000000000000 ) ) ;
#56323=CARTESIAN_POINT ( 'NONE',  ( -12.00000000000000000, -78.89999999999999147, -1.868256502752000067E-14 ) ) ;
#56326=CARTESIAN_POINT ( 'NONE',  ( 0.000000000000000000, -80.89999999999999147, 0.000000000000000000 ) ) ;
#56334=CARTESIAN_POINT ( 'NONE',  ( 8.118221194901000359, -77.64411321036999425, 9.213591238522999660 ) ) ;
#56338=CARTESIAN_POINT ( 'NONE',  ( 1.570796326794857478, -79.66458333333332575, 12.00000000000000533 ) ) ;
#56342=CARTESIAN_POINT ( 'NONE',  ( -0.2648292726109000017, -78.95034006197499821, 10.91353432424999959 ) ) ;
#56344=CARTESIAN_POINT ( 'NONE',  ( -10.75000000000000000, -80.59999999999999432, 0.000000000000000000 ) ) ;
#56354=CARTESIAN_POINT ( 'NONE',  ( -0.08519377839585000334, -78.52556629197296445, 11.97951611939999950 ) ) ;
#56363=CARTESIAN_POINT ( 'NONE',  ( 9.406806676749999596, -76.82832889608799576, -7.895227358184000899 ) ) ;
#56367=ORIENTED_EDGE ( 'NONE', *, *, #49245, .T. ) ;
#56370=CARTESIAN_POINT ( 'NONE',  ( 0.000000000000000000, -75.15999999999999659, 0.000000000000000000 ) ) ;
#56374=CARTESIAN_POINT ( 'NONE',  ( -10.77989530031999976, -78.47947827561399947, -5.637054895855999170 ) ) ;
#56378=CARTESIAN_POINT ( 'NONE',  ( 9.789168614380999500, -79.24010319720299833, -4.831929617604999727 ) ) ;
#56388=CARTESIAN_POINT ( 'NONE',  ( 7.374560639698994002, -78.07708333333332007, -9.596002108778151296 ) ) ;
#56391=CARTESIAN_POINT ( 'NONE',  ( -11.24501830132000002, -78.77221245318798992, 0.6192963436278000611 ) ) ;
#56392=CARTESIAN_POINT ( 'NONE',  ( 11.06827260339915497, -76.61133711981047156, 1.603586413861646021 ) ) ;
#56393=CARTESIAN_POINT ( 'NONE',  ( -10.28470975277595123, -79.09086982037037217, -5.853606176233665082 ) ) ;
#56407=CARTESIAN_POINT ( 'NONE',  ( -10.04675991039999872, -76.77512878623900860, 7.585220848138000349 ) ) ;
#56408=CARTESIAN_POINT ( 'NONE',  ( -0.4971289415107331133, -78.72148840043671214, -10.74989891806322539 ) ) ;
#56411=EDGE_CURVE ( 'NONE', #2822, #15756, #13911, .T. ) ;
#56416=CARTESIAN_POINT ( 'NONE',  ( -5.414008284903408352, -79.68335750799590755, -9.393288886975321716 ) ) ;
#56419=CARTESIAN_POINT ( 'NONE',  ( 6.766402264611000028, -79.51042470825198905, -8.946167390840999545 ) ) ;
#56434=CARTESIAN_POINT ( 'NONE',  ( -9.625846388754000671, -79.20118265956556058, -7.214584339064000318 ) ) ;
#56437=VERTEX_POINT ( 'NONE', #28102 ) ;
#56440=CARTESIAN_POINT ( 'NONE',  ( -6.606781056858329393, -79.17307604219098494, -8.596831229953354025 ) ) ;
#56441=CARTESIAN_POINT ( 'NONE',  ( 8.272973658470998970, -78.18397787739699822, -8.664523719228998999 ) ) ;
#56445=CARTESIAN_POINT ( 'NONE',  ( 8.386770501422327939, -80.90424990314578224, 6.732465268853045970 ) ) ;
#56448=CARTESIAN_POINT ( 'NONE',  ( -4.570437647871999687, -78.36785646258199733, 10.04055945087000090 ) ) ;
#56449=CARTESIAN_POINT ( 'NONE',  ( 1.897323258163000181, -80.38768166943580695, 10.74448230087999967 ) ) ;
#56457=CARTESIAN_POINT ( 'NONE',  ( 10.34070037867000202, -77.98444425272499814, -4.346035695907999319 ) ) ;
#56469=CARTESIAN_POINT ( 'NONE',  ( 12.00000000000000000, -77.04999999999999716, 0.000000000000000000 ) ) ;
#56482=B_SPLINE_CURVE_WITH_KNOTS ( 'NONE', 3,
 ( #50743, #1732, #55146, #32985, #19725, #45435, #24144, #10284, #36558, #51031, #9998, #41574, #50157, #14692, #27978, #46027, #23849, #40995, #36845 ),
 .UNSPECIFIED., .F., .F.,
 ( 4, 1, 1, 1, 2, 2, 1, 1, 2, 2, 2, 4 ),
 ( 0.000000000000000000, 0.1250000000000000278, 0.1875000000000000000, 0.2187500000000001110, 0.2343750000000001388, 0.2500000000000001665, 0.3750000000000008327, 0.4375000000000009437, 0.4687500000000009992, 0.5000000000000011102, 0.7500000000000006661, 1.000000000000000000 ),
 .UNSPECIFIED. ) ;
#56486=CARTESIAN_POINT ( 'NONE',  ( -9.659853700179651170, -81.00000000000000000, -4.855990401126174305 ) ) ;
#56487=CARTESIAN_POINT ( 'NONE',  ( 1.468061006981000061, -77.43767547371999171, 10.81758581523999929 ) ) ;
#56494=B_SPLINE_CURVE_WITH_KNOTS ( 'NONE', 3,
 ( #27951, #45411, #41547, #36819, #14668, #51007, #10258, #28240, #10557, #28540, #24121, #46587, #42139, #37699, #34417, #38279, #11151, #39147 ),
 .UNSPECIFIED., .F., .F.,
 ( 4, 2, 2, 2, 2, 2, 2, 2, 4 ),
 ( 0.000000000000000000, 0.1250000000000000278, 0.2500000000000000555, 0.3750000000000000000, 0.5000000000000000000, 0.6250000000000000000, 0.7500000000000000000, 0.8750000000000001110, 1.000000000000000000 ),
 .UNSPECIFIED. ) ;
#56503=CARTESIAN_POINT ( 'NONE',  ( 9.393203674808285442, -76.70833333333330017, -5.413904038987152667 ) ) ;
#56504=CARTESIAN_POINT ( 'NONE',  ( 12.00000000000000000, -76.66041666666667709, 1.570796326794922093 ) ) ;
#56511=CARTESIAN_POINT ( 'NONE',  ( -11.96278216175999987, -78.19743832925900051, 0.6386762756999999624 ) ) ;
#56519=LINE ( 'NONE', #15493, #44877 ) ;
#56520=ORIENTED_EDGE ( 'NONE', *, *, #26680, .T. ) ;
#56526=CIRCLE ( 'NONE', #15081, 9.599999999999999645 ) ;
#56527=CARTESIAN_POINT ( 'NONE',  ( -2.813980853284178352, -76.99599360018594041, 10.47075201474027928 ) ) ;
#56531=DIRECTION ( 'NONE',  ( 0.000000000000000000, -1.000000000000000000, 0.000000000000000000 ) ) ;
#56535=CARTESIAN_POINT ( 'NONE',  ( 7.081068198472000752, -76.96067567809700449, 8.459326660559002065 ) ) ;
#56541=CARTESIAN_POINT ( 'NONE',  ( 6.477052170204919967, -80.27679150412248532, -8.581165962541923875 ) ) ;
#56545=CARTESIAN_POINT ( 'NONE',  ( 3.714552462503000196, -79.41612481817199409, 11.44155784250999908 ) ) ;
#56547=CARTESIAN_POINT ( 'NONE',  ( 11.26004178396000199, -80.07190303803308495, -0.2131731071575000136 ) ) ;
#56550=VERTEX_POINT ( 'NONE', #52451 ) ;
#56565=CARTESIAN_POINT ( 'NONE',  ( -7.233059401658657350, -80.03400354919075710, 7.953958400202933987 ) ) ;
#56569=CARTESIAN_POINT ( 'NONE',  ( 11.06808393496999976, -76.59534390116400004, 1.603559079323000125 ) ) ;
#56573=EDGE_CURVE ( 'NONE', #20674, #7434, #21722, .T. ) ;
#56574=CARTESIAN_POINT ( 'NONE',  ( -9.775444717333000355, -76.92096869264500469, 5.042056850663000134 ) ) ;
#56580=CARTESIAN_POINT ( 'NONE',  ( -10.48016323062205402, -78.08210605472315535, 2.414871192752478191 ) ) ;
#56590=B_SPLINE_CURVE_WITH_KNOTS ( 'NONE', 3,
 ( #13282, #26281, #8279, #18021, #21278, #40454, #7991, #25988, #35412, #21569, #46, #58163, #36014, #39285, #34840, #53443, #43733, #8569 ),
 .UNSPECIFIED., .F., .F.,
 ( 4, 2, 2, 2, 2, 2, 2, 2, 4 ),
 ( 0.000000000000000000, 0.1250000000000000000, 0.2500000000000000000, 0.3750000000000000000, 0.5000000000000000000, 0.6250000000000000000, 0.7500000000000000000, 0.8750000000000000000, 1.000000000000000000 ),
 .UNSPECIFIED. ) ;
#56599=CARTESIAN_POINT ( 'NONE',  ( -8.418594644163000851, -80.80783708579305369, -7.485750452785000064 ) ) ;
#56606=CARTESIAN_POINT ( 'NONE',  ( 0.4236292209062061387, -79.97211130723771078, 10.75836326857063696 ) ) ;
#56618=CARTESIAN_POINT ( 'NONE',  ( 5.569438312554999548, -79.02790074527499087, 10.68535195481999978 ) ) ;
#56624=ADVANCED_FACE ( 'NONE', ( #28835 ), #3808, .F. ) ;
#56629=CARTESIAN_POINT ( 'NONE',  ( -5.128001663057999870, -78.48732223094400240, 9.637373342098999984 ) ) ;
#56639=CARTESIAN_POINT ( 'NONE',  ( 0.5355496356945241843, -80.72104928547346958, 11.19811601257680600 ) ) ;
#56641=CARTESIAN_POINT ( 'NONE',  ( 8.272973658470998970, -78.33566108400613359, -8.664523719228998999 ) ) ;
#56650=CARTESIAN_POINT ( 'NONE',  ( 8.135116633385999663, -76.81570000444999380, 9.200136113044999675 ) ) ;
#56651=DIRECTION ( 'NONE',  ( 1.000000000000000000, 0.000000000000000000, 0.000000000000000000 ) ) ;
#56653=CARTESIAN_POINT ( 'NONE',  ( 7.374560639698993114, -77.97708333333332575, -9.596002108778149520 ) ) ;
#56661=CARTESIAN_POINT ( 'NONE',  ( -5.775534476593000122, -77.85550402086698796, 10.70634074252000012 ) ) ;
#56665=CARTESIAN_POINT ( 'NONE',  ( -9.692003024890606611, -79.56447609509856989, 4.663514834557163091 ) ) ;
#56668=CARTESIAN_POINT ( 'NONE',  ( 5.024405752997999741, -79.03188383819500018, 10.94290901707999986 ) ) ;
#56670=AXIS2_PLACEMENT_3D ( 'NONE', #1965, #20247, #5782 ) ;
#56680=CARTESIAN_POINT ( 'NONE',  ( 1.784652037779075551, -79.18669371328248019, -11.69830041377290542 ) ) ;
#56694=ORIENTED_EDGE ( 'NONE', *, *, #42819, .T. ) ;
#56695=CARTESIAN_POINT ( 'NONE',  ( 12.37782695028000113, -77.06200795437399620, -2.293983437537999936 ) ) ;
#56696=CARTESIAN_POINT ( 'NONE',  ( -5.679944600031325841, -78.68085203632810476, -9.133896387890597879 ) ) ;
#56697=ADVANCED_FACE ( 'NONE', ( #30791 ), #47441, .F. ) ;
#56700=CARTESIAN_POINT ( 'NONE',  ( 10.61613183210000066, -77.36922082312399596, -2.999913216257000137 ) ) ;
#56704=CARTESIAN_POINT ( 'NONE',  ( -2.787192588043336805, -79.70418878019351894, -10.40599190913065719 ) ) ;
#56707=CARTESIAN_POINT ( 'NONE',  ( -1.472820794058999905, -78.44820733118199030, -10.90095403661999995 ) ) ;
#56712=ORIENTED_EDGE ( 'NONE', *, *, #14771, .T. ) ;
#56716=CARTESIAN_POINT ( 'NONE',  ( -4.531967804315558013, -77.44181088446534034, -10.26074445566288063 ) ) ;
#56733=CARTESIAN_POINT ( 'NONE',  ( 2.956870837876000468, -78.85316765784999404, 11.44999256673999888 ) ) ;
#56741=CARTESIAN_POINT ( 'NONE',  ( 8.060704535212000366, -78.21769278298098982, -7.362092663522000535 ) ) ;
#56742=CARTESIAN_POINT ( 'NONE',  ( 7.293551704196000962, -80.70985390147936300, -8.114658963368000855 ) ) ;
#56751=CARTESIAN_POINT ( 'NONE',  ( 8.164775677042001689, -76.39296509471499519, 9.001221300116000634 ) ) ;
#56754=ORIENTED_EDGE ( 'NONE', *, *, #2708, .F. ) ;
#56756=CARTESIAN_POINT ( 'NONE',  ( 9.892383529026000488, -78.85464906837700028, -4.882876457188000785 ) ) ;
#56770=EDGE_LOOP ( 'NONE', ( #47205, #5277, #15149, #16616, #24133, #10369, #39420 ) ) ;
#56777=CARTESIAN_POINT ( 'NONE',  ( -7.595061814885000651, -78.00963867675800145, 7.841581601742999119 ) ) ;
#56792=CARTESIAN_POINT ( 'NONE',  ( 5.413904038987179312, -76.66666666666664298, -9.393203674808262349 ) ) ;
#56799=CARTESIAN_POINT ( 'NONE',  ( -0.08519377839585000334, -78.57724874519199432, 11.97951611939999950 ) ) ;
#56800=CARTESIAN_POINT ( 'NONE',  ( -8.359900899578630415E-07, -76.12787248224110215, -11.82848710057588626 ) ) ;
#56807=CARTESIAN_POINT ( 'NONE',  ( 10.83766451684999943, -77.55149375871098982, -3.062514061775999608 ) ) ;
#56827=CARTESIAN_POINT ( 'NONE',  ( 9.509459933319000413, -76.93343933509500232, 5.592128946851999238 ) ) ;
#56832=CARTESIAN_POINT ( 'NONE',  ( 6.197920565227482470, -80.27432104992929851, -8.783392821118267690 ) ) ;
#56833=CARTESIAN_POINT ( 'NONE',  ( 9.983882708737807476, -79.88084066504498537, 4.071020308803501742 ) ) ;
#56837=CARTESIAN_POINT ( 'NONE',  ( 2.377756013412999803, -79.13915084896299845, -11.79209151100000064 ) ) ;
#56855=DIRECTION ( 'NONE',  ( 0.000000000000000000, -1.000000000000000000, 0.000000000000000000 ) ) ;
#56857=CARTESIAN_POINT ( 'NONE',  ( -4.459282313423081234, -80.00899937169181442, 9.789565273130554246 ) ) ;
#56859=CARTESIAN_POINT ( 'NONE',  ( -1.432420283025999996, -76.21911477132699986, 11.09153081809999897 ) ) ;
#56862=AXIS2_PLACEMENT_3D ( 'NONE', #25122, #43145, #16276 ) ;
#56863=CARTESIAN_POINT ( 'NONE',  ( 2.063533415121999948, -76.25127502049299721, 10.92068915710999910 ) ) ;
#56870=VECTOR ( 'NONE', #25149, 1000.000000000000000 ) ;
#56871=CARTESIAN_POINT ( 'NONE',  ( -4.368592420383399677, -78.00830336871821657, 9.822916132917713483 ) ) ;
#56884=DIRECTION ( 'NONE',  ( 0.000000000000000000, -1.000000000000000000, 0.000000000000000000 ) ) ;
#56890=CARTESIAN_POINT ( 'NONE',  ( -2.612980907336999614, -80.35637179573859612, -10.95817168551000087 ) ) ;
#56897=CARTESIAN_POINT ( 'NONE',  ( 4.236362259395971996, -79.94289841385737816, 9.879967597326936968 ) ) ;
#56900=CARTESIAN_POINT ( 'NONE',  ( 9.172146100395819346, -77.30629003610285110, -5.638845386412532967 ) ) ;
#56910=CARTESIAN_POINT ( 'NONE',  ( -11.79389253715000052, -77.73916203849999818, 2.981045019388999684 ) ) ;
#56917=ORIENTED_EDGE ( 'NONE', *, *, #22640, .T. ) ;
#56934=CARTESIAN_POINT ( 'NONE',  ( -9.801255020792000394, -76.44685535970599233, 7.399866681860999940 ) ) ;
#56937=CARTESIAN_POINT ( 'NONE',  ( 9.596002108778172612, -77.99791666666665435, -7.374560639698962028 ) ) ;
#56943=CARTESIAN_POINT ( 'NONE',  ( 8.400721904471998513, -78.12679717510499700, -8.798318138657000631 ) ) ;
#56945=CARTESIAN_POINT ( 'NONE',  ( 6.586108526242999694, -80.07391735373440156, 8.810401493720998900 ) ) ;
#56948=CARTESIAN_POINT ( 'NONE',  ( -10.74994525727461259, -79.59655355021966727, 0.4779014380844182064 ) ) ;
#56951=CARTESIAN_POINT ( 'NONE',  ( -3.882040082920265700, -78.80112713863415763, 11.40455788431460249 ) ) ;
#56952=CARTESIAN_POINT ( 'NONE',  ( -7.282623421190000279, -79.61782371684098791, 9.589350811714000500 ) ) ;
#56955=CARTESIAN_POINT ( 'NONE',  ( -1.413307538656764395, -76.24661458376434098, -10.80338542964358517 ) ) ;
#56962=CARTESIAN_POINT ( 'NONE',  ( 3.686727602956580530, -78.89922203454568717, 11.17960410108377367 ) ) ;
#56976=CARTESIAN_POINT ( 'NONE',  ( 12.54822461858999993, -76.57021509471499598, -1.007481608483999924 ) ) ;
#56977=CARTESIAN_POINT ( 'NONE',  ( 4.122725566465639702, -78.75634067257766446, -9.928003433801906752 ) ) ;
#56987=CARTESIAN_POINT ( 'NONE',  ( 11.14115696400000033, -79.07464322022299541, -1.301050381412999890 ) ) ;
#56996=CARTESIAN_POINT ( 'NONE',  ( 10.75931538509122021, -78.12271945951098928, 3.171551892671853334 ) ) ;
#57005=DIRECTION ( 'NONE',  ( 1.000000000000000000, 0.000000000000000000, 0.000000000000000000 ) ) ;
#57012=CARTESIAN_POINT ( 'NONE',  ( -9.964549960864999889, -77.51927491423099070, 6.650098383618000319 ) ) ;
#57018=CARTESIAN_POINT ( 'NONE',  ( -10.67318205552422761, -76.59044953065486538, 1.292397307245511717 ) ) ;
#57028=CARTESIAN_POINT ( 'NONE',  ( -11.61792497750000130, -79.30050612125899079, 3.950725441919999970 ) ) ;
#57031=CARTESIAN_POINT ( 'NONE',  ( 5.263131812197999970, -77.99776011999799152, -9.905430536777000583 ) ) ;
#57035=CARTESIAN_POINT ( 'NONE',  ( 4.613038445363000228, -76.78576930215800189, 11.49595188101000076 ) ) ;
#57039=CARTESIAN_POINT ( 'NONE',  ( 5.650974246042000715, -78.47334026635199677, 9.474609463724998903 ) ) ;
#57044=DIRECTION ( 'NONE',  ( 4.275554269583999736E-12, 1.000000000000000000, -1.682668868129999999E-10 ) ) ;
#57061=CARTESIAN_POINT ( 'NONE',  ( 9.605397716210999803, -76.78400324167699864, -5.187648860687999353 ) ) ;
#57065=CARTESIAN_POINT ( 'NONE',  ( -8.382198119002001846, -79.75615640372498660, -7.453647783897999979 ) ) ;
#57074=CARTESIAN_POINT ( 'NONE',  ( 10.47020627418439531, -76.72916666666667140, -2.813789756862242974 ) ) ;
#57079=CARTESIAN_POINT ( 'NONE',  ( -8.351691841945999784, -76.51493262182999899, 7.546656452382999980 ) ) ;
#57083=DIRECTION ( 'NONE',  ( 1.000000000000000000, 0.000000000000000000, 0.000000000000000000 ) ) ;
#57086=CARTESIAN_POINT ( 'NONE',  ( -5.883052656872999719, -77.74214815972399606, 9.603314844095001135 ) ) ;
#57088=CARTESIAN_POINT ( 'NONE',  ( 4.382699061554999886, -81.04870889205099616, -10.08957852304999925 ) ) ;
#57091=CARTESIAN_POINT ( 'NONE',  ( 0.000000000000000000, -87.70000000000000284, 0.000000000000000000 ) ) ;
#57104=B_SPLINE_CURVE_WITH_KNOTS ( 'NONE', 3,
 ( #56945, #12356, #30920, #11790 ),
 .UNSPECIFIED., .F., .F.,
 ( 4, 4 ),
 ( 0.000000000000000000, 1.000000000000000000 ),
 .UNSPECIFIED. ) ;
#57107=CARTESIAN_POINT ( 'NONE',  ( -0.8117802668354000550, -77.26027545111699624, -11.00194288205000070 ) ) ;
#57113=CARTESIAN_POINT ( 'NONE',  ( -4.051423106035414001, -80.19464027527671135, -9.957102339836081839 ) ) ;
#57116=CARTESIAN_POINT ( 'NONE',  ( 7.520016693046000178, -79.67705620421800461, -9.389162645085001202 ) ) ;
#57118=CARTESIAN_POINT ( 'NONE',  ( -5.416162833245999231, -79.90848498002219458, -9.874165520190000933 ) ) ;
#57119=CARTESIAN_POINT ( 'NONE',  ( 10.47007982758580447, -77.37089620502051446, 2.813809139533428372 ) ) ;
#57124=DIRECTION ( 'NONE',  ( 0.000000000000000000, -1.000000000000000000, 0.000000000000000000 ) ) ;
#57139=EDGE_CURVE ( 'NONE', #353, #54955, #49077, .T. ) ;
#57140=CARTESIAN_POINT ( 'NONE',  ( -10.24633426275284265, -80.07555679980247021, 3.252597035816566784 ) ) ;
#57143=CARTESIAN_POINT ( 'NONE',  ( 10.12567350656000009, -76.11878700336998804, 4.748118780173999909 ) ) ;
#57145=EDGE_CURVE ( 'NONE', #28272, #40983, #22265, .T. ) ;
#57147=CARTESIAN_POINT ( 'NONE',  ( 10.88552170588999957, -76.72031315673200424, 1.577109214857000064 ) ) ;
#57163=LINE ( 'NONE', #25003, #40459 ) ;
#57166=CARTESIAN_POINT ( 'NONE',  ( 10.86112223246497344, -80.98224957254201684, -2.453532618892452444 ) ) ;
#57167=CARTESIAN_POINT ( 'NONE',  ( 7.745630616141999880, -80.09064385942969011, 8.037401158237999610 ) ) ;
#57168=EDGE_CURVE ( 'NONE', #12394, #5899, #17011, .T. ) ;
#57190=AXIS2_PLACEMENT_3D ( 'NONE', #31771, #42110, #27924 ) ;
#57193=EDGE_CURVE ( 'NONE', #38464, #24242, #53704, .T. ) ;
#57204=PLANE ( 'NONE',  #27706 ) ;
#57207=CARTESIAN_POINT ( 'NONE',  ( -0.7928179559538000021, -78.76973013078654162, -11.95355612867000339 ) ) ;
#57219=CARTESIAN_POINT ( 'NONE',  ( -6.043427764450786555, -77.88333333333332575, -10.48543666025110177 ) ) ;
#57225=CIRCLE ( 'NONE', #50684, 11.70000000000000107 ) ;
#57226=CARTESIAN_POINT ( 'NONE',  ( 3.113304451009999863, -78.49783470746899638, -10.55022916317000181 ) ) ;
#57228=CARTESIAN_POINT ( 'NONE',  ( 3.002529760384999857, -78.79598695555699805, 11.62679918156999825 ) ) ;
#57233=CARTESIAN_POINT ( 'NONE',  ( -5.896991955202756763, -79.52120778372643883, 8.992014754021855794 ) ) ;
#57235=CARTESIAN_POINT ( 'NONE',  ( -9.797890753601748770, -78.85056356931703192, 7.009672782845664862 ) ) ;
#57237=CARTESIAN_POINT ( 'NONE',  ( 4.220196950471000186, -79.60564988871099956, 11.40022119696999958 ) ) ;
#57243=CARTESIAN_POINT ( 'NONE',  ( 11.68767212001979239, -78.12916666666666288, -3.140974612311342451 ) ) ;
#57245=ORIENTED_EDGE ( 'NONE', *, *, #44633, .T. ) ;
#57247=CARTESIAN_POINT ( 'NONE',  ( 11.00000000000000000, -81.00000000000000000, -2.369510767747999942E-13 ) ) ;
#57258=CARTESIAN_POINT ( 'NONE',  ( 8.596576764504078483, -78.40209458680075727, 6.606494579572424364 ) ) ;
#57263=CARTESIAN_POINT ( 'NONE',  ( 3.138727503548000008, -77.40410827300999586, -12.06897532934999973 ) ) ;
#57264=CARTESIAN_POINT ( 'NONE',  ( 5.072952311206533338, -78.76416732819434685, -9.477694199498785110 ) ) ;
#57273=CARTESIAN_POINT ( 'NONE',  ( -5.859445663532000026, -77.66873914051188876, 9.564779511708000115 ) ) ;
#57294=CARTESIAN_POINT ( 'NONE',  ( -9.393203674808267678, -79.54166666666665719, -5.413904038987171319 ) ) ;
#57301=CARTESIAN_POINT ( 'NONE',  ( 10.68063106575048593, -79.33970932340548643, -1.407236774638731980 ) ) ;
#57302=CARTESIAN_POINT ( 'NONE',  ( -8.148905501844000199, -78.56378829332899727, -8.781309899900000104 ) ) ;
#57314=CARTESIAN_POINT ( 'NONE',  ( 7.803849947780999052, -79.64674332227700404, 9.470181462888000112 ) ) ;
#57317=CARTESIAN_POINT ( 'NONE',  ( -11.21668965365999959, -77.83434206198700167, -0.06311738993059998193 ) ) ;
#57320=CARTESIAN_POINT ( 'NONE',  ( -10.68812519998999910, -76.89896751707298961, 6.261071428515000648 ) ) ;
#57324=CARTESIAN_POINT ( 'NONE',  ( 10.36875976864000037, -78.41886758034799243, 3.767035497191999927 ) ) ;
#57330=CARTESIAN_POINT ( 'NONE',  ( 10.25000000000000000, -82.09999999999999432, 0.000000000000000000 ) ) ;
#57344=CARTESIAN_POINT ( 'NONE',  ( -3.834123575518456395, -81.00000000000002842, -10.21712803629676536 ) ) ;
#57345=CARTESIAN_POINT ( 'NONE',  ( 2.897215155706000189, -77.21978472970600649, -10.52527958449999979 ) ) ;
#57351=CARTESIAN_POINT ( 'NONE',  ( 6.879576957522999692, -79.02077514267600122, 8.859431780707000215 ) ) ;
#57370=CARTESIAN_POINT ( 'NONE',  ( -12.06632373222999988, -79.58087695312399035, -0.6505690833180000077 ) ) ;
#57372=CARTESIAN_POINT ( 'NONE',  ( 10.99419336675999936, -78.98418847654799890, 4.758540471090999979 ) ) ;
#57377=SURFACE_SIDE_STYLE ('',( #25787 ) ) ;
#57379=CARTESIAN_POINT ( 'NONE',  ( 4.292950718366999929, -76.97953055567299430, -10.41175003194000048 ) ) ;
#57381=CARTESIAN_POINT ( 'NONE',  ( 4.228967157898000373, -80.66775882426230737, 10.43118177971000016 ) ) ;
#57399=CARTESIAN_POINT ( 'NONE',  ( -11.07095105964000048, -78.19956549158798964, 1.299477954992000139 ) ) ;
#57405=CARTESIAN_POINT ( 'NONE',  ( 1.469922439804874026, -80.23638809882929479, -10.65449918043788635 ) ) ;
#57408=CARTESIAN_POINT ( 'NONE',  ( 10.12072861152395298, -79.63538404776677737, 4.836575372680795404 ) ) ;
#57410=CARTESIAN_POINT ( 'NONE',  ( -5.092641036025000290, -79.47589207986699478, 10.89826376711000044 ) ) ;
#57412=CARTESIAN_POINT ( 'NONE',  ( 4.801746450173999925, -79.66335789300599401, 10.18710928510000002 ) ) ;
#57422=CARTESIAN_POINT ( 'NONE',  ( 7.921848887473175616, -78.29045646104971468, -7.357746221004406451 ) ) ;
#57429=CARTESIAN_POINT ( 'NONE',  ( 2.774709120699121456, -79.79999999999999716, 11.60977811668827364 ) ) ;
#57430=CARTESIAN_POINT ( 'NONE',  ( -6.857072527857152267, -80.03044501592233928, 8.278933358856727764 ) ) ;
#57437=CARTESIAN_POINT ( 'NONE',  ( -5.138289791457000710, -76.61246662722099643, -9.595228483104000006 ) ) ;
#57441=CYLINDRICAL_SURFACE ( 'NONE', #54411, 12.00000000000000000 ) ;
#57444=AXIS2_PLACEMENT_3D ( 'NONE', #6315, #37022, #42044 ) ;
#57453=CYLINDRICAL_SURFACE ( 'NONE', #20607, 12.00000000000000000 ) ;
#57458=CARTESIAN_POINT ( 'NONE',  ( 11.00000000000000000, -81.00000000000000000, -2.369510767747999942E-13 ) ) ;
#57464=CARTESIAN_POINT ( 'NONE',  ( -1.738099071051254940, -79.98838542116494921, 10.60879108008627902 ) ) ;
#57483=ORIENTED_EDGE ( 'NONE', *, *, #5230, .F. ) ;
#57501=CARTESIAN_POINT ( 'NONE',  ( -6.018890980713000438, -75.91407976174099304, 10.70471907396000155 ) ) ;
#57502=DIRECTION ( 'NONE',  ( -1.000000000000000000, 0.000000000000000000, 0.000000000000000000 ) ) ;
#57510=AXIS2_PLACEMENT_3D ( 'NONE', #22385, #40396, #13819 ) ;
#57511=CARTESIAN_POINT ( 'NONE',  ( -3.162453476786999840, -77.97768216442000266, -11.86569286591000072 ) ) ;
#57517=CARTESIAN_POINT ( 'NONE',  ( -6.422077643389767942, -79.52599266752667972, 8.620883091140045806 ) ) ;
#57520=CARTESIAN_POINT ( 'NONE',  ( 1.162094749123000037, -79.12624453345600273, 12.10061229221000012 ) ) ;
#57547=CARTESIAN_POINT ( 'NONE',  ( -0.6708319208533000122, -76.31181275097399919, -12.33441669056000123 ) ) ;
#57548=CARTESIAN_POINT ( 'NONE',  ( -10.45176477158148742, -78.61882830641657449, -2.514439583694316305 ) ) ;
#57555=CARTESIAN_POINT ( 'NONE',  ( -4.647088938219000376, -78.15899331454487253, 10.20895072913000057 ) ) ;
#57558=CARTESIAN_POINT ( 'NONE',  ( 5.865103843792000227, -78.57046857046199761, -9.561319920857000554 ) ) ;
#57574=CARTESIAN_POINT ( 'NONE',  ( 5.753255980621002408, -78.98433428202568507, 10.26026234797696723 ) ) ;
#57578=VERTEX_POINT ( 'NONE', #48344 ) ;
#57581=CARTESIAN_POINT ( 'NONE',  ( -10.40626589979188488, -79.12100314181128624, -2.787243473566140661 ) ) ;
#57582=CARTESIAN_POINT ( 'NONE',  ( 11.88382656225999945, -78.23823650824398612, -1.513515996960000054 ) ) ;
#57596=CARTESIAN_POINT ( 'NONE',  ( 0.2436306363661999985, -79.70001058397200211, 12.26886527195999932 ) ) ;
#57600=CARTESIAN_POINT ( 'NONE',  ( -11.31839317768999997, -76.97443299368299563, -5.033003383563999122 ) ) ;
#57605=CARTESIAN_POINT ( 'NONE',  ( -4.084105282113999813, -79.23595787040198957, -10.24801534084000032 ) ) ;
#57613=CARTESIAN_POINT ( 'NONE',  ( -9.933360547807000174, -78.37660472681200474, -7.219704108085999827 ) ) ;
#57615=CARTESIAN_POINT ( 'NONE',  ( -2.813789756862300262, -79.39583333333331439, 10.47020627418438465 ) ) ;
#57623=CARTESIAN_POINT ( 'NONE',  ( 10.54436264862384043, -78.83449620097776744, -2.092280515037520772 ) ) ;
#57626=ORIENTED_EDGE ( 'NONE', *, *, #26342, .F. ) ;
#57629=CARTESIAN_POINT ( 'NONE',  ( -10.51004847261784114, -80.99999999999998579, -2.396571149024055547 ) ) ;
#57630=CARTESIAN_POINT ( 'NONE',  ( 10.72166763895999964, -76.83847592767999402, 2.054558110510000368 ) ) ;
#57633=CARTESIAN_POINT ( 'NONE',  ( -5.394429334091999984, -79.85118130000350334, -9.834543342166998769 ) ) ;
#57650=CARTESIAN_POINT ( 'NONE',  ( -9.555168389065999079, -79.12901475210699687, -7.397172803072000313 ) ) ;
#57652=CARTESIAN_POINT ( 'NONE',  ( 2.697636866285999968, -77.84475722874999803, -11.67213861177999945 ) ) ;
#57659=CARTESIAN_POINT ( 'NONE',  ( -8.763613300111000370, -76.77071859265899434, 6.838397221053000408 ) ) ;
#57661=CARTESIAN_POINT ( 'NONE',  ( -11.22958316615000207, -80.82884494028411382, -0.7682314979056000803 ) ) ;
#57668=CARTESIAN_POINT ( 'NONE',  ( 7.155101792066000499, -78.37967353048000518, -8.354909834651998324 ) ) ;
#57677=CARTESIAN_POINT ( 'NONE',  ( 7.154950478465999630, -77.02840274250999641, 8.547589380727000474 ) ) ;
#57684=CARTESIAN_POINT ( 'NONE',  ( -5.040219434754469319, -80.18634211511320586, -9.501857774222978392 ) ) ;
#57685=CARTESIAN_POINT ( 'NONE',  ( -10.75000000000000000, -77.01041666666665719, -1.407171709420429018 ) ) ;
#57689=CARTESIAN_POINT ( 'NONE',  ( 4.847151869481000297, -78.84031454048799503, 11.00961342987999991 ) ) ;
#57691=EDGE_CURVE ( 'NONE', #38899, #14050, #17346, .T. ) ;
#57692=CARTESIAN_POINT ( 'NONE',  ( 10.53539001158999966, -80.04466669503129594, -3.979889026714000355 ) ) ;
#57696=ORIENTED_EDGE ( 'NONE', *, *, #39537, .T. ) ;
#57701=DIRECTION ( 'NONE',  ( 0.000000000000000000, 1.000000000000000000, 0.000000000000000000 ) ) ;
#57702=CARTESIAN_POINT ( 'NONE',  ( 1.070392484793000198, -79.44059423600799619, 10.86414404906000009 ) ) ;
#57718=CARTESIAN_POINT ( 'NONE',  ( 0.000000000000000000, -76.08749999999699298, 0.000000000000000000 ) ) ;
#57727=CARTESIAN_POINT ( 'NONE',  ( -0.9004183036393477169, -80.98178841101156422, 10.71218087055294532 ) ) ;
#57728=CARTESIAN_POINT ( 'NONE',  ( 11.22355342542000045, -80.65854382077790774, 0.9700744431168999427 ) ) ;
#57732=CARTESIAN_POINT ( 'NONE',  ( -8.596418555780440229, -80.05208333333332860, -6.606377239730328199 ) ) ;
#57751=CARTESIAN_POINT ( 'NONE',  ( -1.347939806071310143, -79.98541859949588684, 10.66559394157654950 ) ) ;
#57754=CARTESIAN_POINT ( 'NONE',  ( -4.478752552746194660, -77.19081009185403275, -9.773648971711729416 ) ) ;
#57761=ADVANCED_FACE ( 'NONE', ( #14057 ), #8570, .T. ) ;
#57764=CARTESIAN_POINT ( 'NONE',  ( -12.11185258877999971, -77.76629135392300896, -1.133824260204999934 ) ) ;
#57769=CARTESIAN_POINT ( 'NONE',  ( 9.799999999999998934, -92.13603921945998820, -1.131976457013999809E-12 ) ) ;
#57781=AXIS2_PLACEMENT_3D ( 'NONE', #5839, #23272, #13821 ) ;
#57782=CARTESIAN_POINT ( 'NONE',  ( 11.06070397063424693, -80.58681085545528333, -1.829055307137330111 ) ) ;
#57790=LINE ( 'NONE', #53360, #55894 ) ;
#57792=CARTESIAN_POINT ( 'NONE',  ( -11.94395460750000204, -76.97963095766999686, 2.857367593729999822 ) ) ;
#57793=CARTESIAN_POINT ( 'NONE',  ( 11.59999999999999964, -90.29999999999999716, 0.000000000000000000 ) ) ;
#57800=CARTESIAN_POINT ( 'NONE',  ( -10.57583826563999985, -77.04653003390299659, -2.706834349011999930 ) ) ;
#57801=CARTESIAN_POINT ( 'NONE',  ( -12.03507225495000199, -78.35749258035299647, 2.439839133843999974 ) ) ;
#57806=CARTESIAN_POINT ( 'NONE',  ( -3.736121491853147791, -79.50337531813939052, 10.07978767405712617 ) ) ;
#57810=CARTESIAN_POINT ( 'NONE',  ( -5.602477186682999211, -79.77762550192599633, -10.65853832389000111 ) ) ;
#57811=CARTESIAN_POINT ( 'NONE',  ( -11.16943811108000162, -80.64298588867529816, -0.2596301638153999947 ) ) ;
#57813=CARTESIAN_POINT ( 'NONE',  ( 0.000000000000000000, -76.00000000000000000, 0.000000000000000000 ) ) ;
#57839=CARTESIAN_POINT ( 'NONE',  ( 8.104433285180000723, -76.94079223774500065, 9.165435814006000825 ) ) ;
#57844=EDGE_CURVE ( 'NONE', #8174, #23335, #32125, .T. ) ;
#57847=CARTESIAN_POINT ( 'NONE',  ( -10.58728162385000005, -77.72321182651586469, 3.705074683290000337 ) ) ;
#57852=CARTESIAN_POINT ( 'NONE',  ( 3.371435477143000181, -79.55097691852699882, -10.69820234502000034 ) ) ;
#57871=CARTESIAN_POINT ( 'NONE',  ( 11.21485848424000054, -79.99849401882083555, -0.2123177049684000228 ) ) ;
#57876=CARTESIAN_POINT ( 'NONE',  ( 0.4844284812283000119, -77.37009841468399429, 11.97002061314999999 ) ) ;
#57877=CARTESIAN_POINT ( 'NONE',  ( -10.75000000000000000, -78.10000000000000853, 0.000000000000000000 ) ) ;
#57879=CARTESIAN_POINT ( 'NONE',  ( 2.945718361321999712, -78.93144108438299611, 11.40680644849000025 ) ) ;
#57894=CARTESIAN_POINT ( 'NONE',  ( 6.027877668513000664, -76.10658001266899930, -10.82135396111999981 ) ) ;
#57898=CARTESIAN_POINT ( 'NONE',  ( -9.575027280576000166, -79.09977615539300189, 5.479104576271000226 ) ) ;
#57903=B_SPLINE_SURFACE_WITH_KNOTS ( 'NONE', 3, 3, ( 
 ( #30770, #15846, #48803, #6984, #28824, #6697, #46873, #48518, #15260, #2283, #12774, #39642, #19694, #57370, #15555, #6400, #29119, #8349, #20279, #56005, #24415, #8063, #38272, #33548, #26347, #12492, #57650, #24705, #37981, #26058, #44084, #47165, #2000, #44364, #56293 ),
 ( #3635, #33834, #51587, #37694, #30490, #17206, #42717, #11145, #21638, #35194, #51872, #19994, #55713, #11426, #51294, #29406, #10851, #42431, #47459, #24988, #16929, #43008, #2565, #20566, #38564, #34910, #52942, #27804, #4807, #45260, #54406, #22808, #13651, #36380, #39928 ),
 ( #36093, #40226, #13944, #31940, #3917, #35787, #13354, #57944, #40819, #26929, #49984, #58238, #17498, #700, #49092, #18682, #14231, #27513, #49393, #36674, #35486, #23099, #17801, #27221, #53516, #53817, #5100, #411, #54690, #13057, #31352, #18097, #32230, #26629, #8942 ),
 ( #41109, #44960, #4515, #45554, #18389, #31056, #50272, #9527, #9820, #49689, #54110, #21920, #119, #8644, #31646, #44664, #22516, #4218, #22215, #40526, #9235, #18970, #28386, #10115, #11282, #28095, #23678, #23391, #20140, #46144, #19846, #46434, #42283, #24558, #33693 ) ),
 .UNSPECIFIED., .F., .F., .F.,
 ( 4, 4 ),
 ( 4, 1, 1, 1, 1, 1, 1, 1, 1, 1, 1, 1, 1, 1, 1, 1, 1, 1, 1, 1, 1, 1, 1, 1, 1, 1, 1, 1, 1, 1, 1, 1, 4 ),
 ( -0.1772706441294000235, 1.177270644128999955 ),
 ( 0.3465776244131999473, 0.3673974550078999979, 0.3882172856025000174, 0.4090371161971999570, 0.4298569467919000076, 0.4506767773865999471, 0.4714966079812999977, 0.4923164385759000172, 0.5131362691705999568, 0.5339560997653000074, 0.5547759303600000580, 0.5755957609545999665, 0.5964155915493000171, 0.6172354221440000677, 0.6380552527387000072, 0.6588750833333999468, 0.6796949139279999663, 0.7005147445227000169, 0.7213345751173999565, 0.7421544057121000071, 0.7629742363067000266, 0.7837940669013999662, 0.8046138974961000168, 0.8254337280908000674, 0.8462535586855000069, 0.8670733892801000264, 0.8878932198747999660, 0.9087130504695000166, 0.9295328810641999562, 0.9503527116587999757, 0.9711725422535000263, 0.9919923728481999659, 1.012812203443000048 ),
 .UNSPECIFIED. ) ;
#57905=LINE ( 'NONE', #21882, #3419 ) ;
#57907=CARTESIAN_POINT ( 'NONE',  ( 7.091067894987999942, -79.00057898155800729, -10.02559399679999963 ) ) ;
#57910=DIRECTION ( 'NONE',  ( -1.000000000000000000, 0.000000000000000000, 0.000000000000000000 ) ) ;
#57920=CARTESIAN_POINT ( 'NONE',  ( 5.066356038949999530, -77.47816619513099567, 9.799682181994000985 ) ) ;
#57925=CARTESIAN_POINT ( 'NONE',  ( 9.453938376997999882, -78.99353879967499381, 6.036651369377000087 ) ) ;
#57930=B_SPLINE_CURVE_WITH_KNOTS ( 'NONE', 3,
 ( #43347, #43067, #3762, #53353, #25330, #35035, #30033, #52495, #39768, #25044, #8193, #16198, #56639, #3200, #47796, #48649, #43928, #57782, #2625, #38623, #39192, #43641, #26196, #34176, #12900, #25618, #2904, #7617, #20904, #47518, #17336, #52781, #12335, #29744, #52212 ),
 .UNSPECIFIED., .F., .F.,
 ( 4, 1, 1, 1, 1, 1, 1, 1, 1, 1, 1, 1, 1, 1, 1, 1, 1, 1, 1, 1, 1, 1, 1, 1, 1, 1, 1, 1, 1, 1, 1, 1, 4 ),
 ( 0.000000000000000000, 0.01250051965580525719, 0.04500048563628020193, 0.07750045161695787166, 0.1100004175974328147, 0.1425003835781102624, 0.1750003495585852054, 0.2075003155390599263, 0.2400002815197375960, 0.2725002475002122893, 0.3050002134806872323, 0.3375001794613649020, 0.3700001454418396230, 0.4025001114225172927, 0.4350000774029922357, 0.4675000433834667346, 0.5000000093641446819, 0.5324999753446193473, 0.5649999413252972946, 0.5974999073057719601, 0.6299998732862467365, 0.6624998392669243508, 0.6949998052473993493, 0.7274997712280767415, 0.7599997372085517400, 0.7924997031890266275, 0.8249996691697041307, 0.8574996351501790182, 0.8899996011308567434, 0.9224995671113316309, 0.9549995330918061853, 0.9874994990724837995, 1.000000000000000000 ),
 .UNSPECIFIED. ) ;
#57938=EDGE_CURVE ( 'NONE', #23344, #50686, #26465, .T. ) ;
#57944=CARTESIAN_POINT ( 'NONE',  ( 10.99809925207999939, -79.65397460938399377, -5.545072090542999987 ) ) ;
#57946=CARTESIAN_POINT ( 'NONE',  ( -7.077166588276162962, -78.03223210419182010, 8.091922746255471921 ) ) ;
#57947=CARTESIAN_POINT ( 'NONE',  ( -10.26943924278000075, -78.59084813818699899, 6.168847710360999770 ) ) ;
#57954=CARTESIAN_POINT ( 'NONE',  ( -2.318770996637999904, -77.71491181672199389, 11.02076520135999971 ) ) ;
#57955=CARTESIAN_POINT ( 'NONE',  ( -12.00000000000000000, -78.29999999999999716, 0.000000000000000000 ) ) ;
#57956=CARTESIAN_POINT ( 'NONE',  ( -10.82155256717999947, -80.34558659221879395, -3.096403820615999614 ) ) ;
#57973=CARTESIAN_POINT ( 'NONE',  ( -4.665811493888000427, -78.18558352699498926, 10.25008134894000023 ) ) ;
#57977=CARTESIAN_POINT ( 'NONE',  ( -3.321932689530000093, -81.00000000000000000, 10.22385755016999909 ) ) ;
#57980=CARTESIAN_POINT ( 'NONE',  ( 0.01100736988436660027, -80.22531903115304885, -10.74985747427674632 ) ) ;
#57982=CARTESIAN_POINT ( 'NONE',  ( 8.733980040321597471, -78.54593032769474803, -7.038404617877435321 ) ) ;
#57986=CARTESIAN_POINT ( 'NONE',  ( 3.350422000336999773, -79.54043055640599391, -10.63152260923000014 ) ) ;
#57997=CARTESIAN_POINT ( 'NONE',  ( 11.02987528609000023, -79.88963010244600582, -0.2088156359816000229 ) ) ;
#58014=AXIS2_PLACEMENT_3D ( 'NONE', #25870, #2586, #53034 ) ;
#58015=CARTESIAN_POINT ( 'NONE',  ( -9.568646597019998978, -76.48705691727600708, 5.187623148002000306 ) ) ;
#58022=CARTESIAN_POINT ( 'NONE',  ( 12.00000000000000533, -77.54258394437167112, -1.118314842272786214 ) ) ;
#58023=CARTESIAN_POINT ( 'NONE',  ( -0.8464931918749931672, -80.98139962866328290, 10.71653294235299292 ) ) ;
#58024=CARTESIAN_POINT ( 'NONE',  ( 1.328862289696999932, -80.19948534945449126, 11.18676134159000135 ) ) ;
#58029=EDGE_CURVE ( 'NONE', #18786, #4693, #43483, .T. ) ;
#58040=CARTESIAN_POINT ( 'NONE',  ( -10.48543666025109289, -78.94166666666666288, -6.043427764450796325 ) ) ;
#58048=CARTESIAN_POINT ( 'NONE',  ( -2.489408411739813420, -77.20657166405426608, -10.45779613294925348 ) ) ;
#58058=EDGE_LOOP ( 'NONE', ( #40769, #41305, #11194, #54452 ) ) ;
#58059=CARTESIAN_POINT ( 'NONE',  ( -11.99726733138999890, -77.69856428951000282, -1.123097615067000010 ) ) ;
#58060=ORIENTED_EDGE ( 'NONE', *, *, #36471, .F. ) ;
#58064=CARTESIAN_POINT ( 'NONE',  ( -11.68767212001979594, -78.77916666666666856, 3.140974612311315806 ) ) ;
#58076=CARTESIAN_POINT ( 'NONE',  ( 8.049666437455634593, -77.33396340929790824, -8.806025772650324157 ) ) ;
#58095=CARTESIAN_POINT ( 'NONE',  ( 5.122310662682999727, -78.19045643997900186, -9.640399341584998893 ) ) ;
#58096=CARTESIAN_POINT ( 'NONE',  ( 1.675539995062999887, -78.73730299628599028, 11.92720225554999836 ) ) ;
#58104=CARTESIAN_POINT ( 'NONE',  ( -4.600316697258000076, -80.98327349430469724, 9.793279191701000030 ) ) ;
#58108=CARTESIAN_POINT ( 'NONE',  ( -3.244487197725999916, -76.93554274292699802, -10.73738397614000029 ) ) ;
#58121=CARTESIAN_POINT ( 'NONE',  ( -14.00000000000000000, -91.29999999999999716, 8.108919984112999312E-14 ) ) ;
#58127=ORIENTED_EDGE ( 'NONE', *, *, #14386, .F. ) ;
#58133=CARTESIAN_POINT ( 'NONE',  ( -10.57243353979999867, -76.14788179775399612, 6.388556512783999608 ) ) ;
#58134=CARTESIAN_POINT ( 'NONE',  ( -10.45298374846471567, -78.61878984457777619, -2.509360686428254272 ) ) ;
#58143=CARTESIAN_POINT ( 'NONE',  ( -0.02522423216716376468, -78.37478882719507567, -11.17055116352559452 ) ) ;
#58146=CARTESIAN_POINT ( 'NONE',  ( -9.805641529082999241, -79.44203154651999910, -5.446788484474000214 ) ) ;
#58156=CARTESIAN_POINT ( 'NONE',  ( -9.801255020792000394, -76.65022101953400124, 7.399866681860999940 ) ) ;
#58161=CARTESIAN_POINT ( 'NONE',  ( -6.606377239730330864, -79.57291666666665719, -8.596418555780440229 ) ) ;
#58163=CARTESIAN_POINT ( 'NONE',  ( 5.413904038987143785, -77.83333333333332860, 9.393203674808290771 ) ) ;
#58169=CARTESIAN_POINT ( 'NONE',  ( 4.458743082292000004, -77.34296909926000296, 11.11915799896999957 ) ) ;
#58170=CYLINDRICAL_SURFACE ( 'NONE', #33450, 10.75000000000000000 ) ;
#58172=CARTESIAN_POINT ( 'NONE',  ( 1.628430890020000188, -78.94048418952499446, 11.59185972383999896 ) ) ;
#58177=CARTESIAN_POINT ( 'NONE',  ( -1.733234625524999961, -80.13890251626278882, -10.77827740047999860 ) ) ;
#58187=CARTESIAN_POINT ( 'NONE',  ( -1.134051983850000056, -76.89122910487600393, 12.21726166519999879 ) ) ;
#58189=CARTESIAN_POINT ( 'NONE',  ( 4.316049272395066083, -76.84239669216790958, 9.924321351449295392 ) ) ;
#58192=CARTESIAN_POINT ( 'NONE',  ( 6.010232441408999371, -80.10679326027729985, 9.524218016016000377 ) ) ;
#58195=DIRECTION ( 'NONE',  ( 0.000000000000000000, -1.000000000000000000, 0.000000000000000000 ) ) ;
#58201=CARTESIAN_POINT ( 'NONE',  ( -8.771511755855000203, -77.88827704918399775, -8.593972346821999508 ) ) ;
#58210=CARTESIAN_POINT ( 'NONE',  ( 10.55352543338477389, -78.83484157365509759, -2.045682359817731832 ) ) ;
#58215=CARTESIAN_POINT ( 'NONE',  ( 1.606468910658999993, -77.77776596815100163, -10.91425636589999826 ) ) ;
#58219=CARTESIAN_POINT ( 'NONE',  ( -2.710423231297999891, -79.66052689899100869, 10.88447134676999895 ) ) ;
#58223=ADVANCED_FACE ( 'NONE', ( #45598, #36422 ), #54448, .T. ) ;
#58238=CARTESIAN_POINT ( 'NONE',  ( -7.388677236831999728, -79.51494008599399876, -9.854616049676000245 ) ) ;
#58239=CARTESIAN_POINT ( 'NONE',  ( 2.909452169864999771, -76.42760485387299241, 10.87394468084000110 ) ) ;
#58240=CARTESIAN_POINT ( 'NONE',  ( -5.260139927115998759, -78.01577672530346774, 9.375410799120500016 ) ) ;
#58241=EDGE_CURVE ( 'NONE', #616, #6742, #25718, .T. ) ;
#58242=CARTESIAN_POINT ( 'NONE',  ( -0.08519377839585000334, -78.50946019191600556, 11.97951611939999950 ) ) ;
#58248=CARTESIAN_POINT ( 'NONE',  ( 5.439600774063181099, -80.93322674150709872, 9.274161813587999958 ) ) ;
#58252=CARTESIAN_POINT ( 'NONE',  ( -10.79885705035999877, -76.91107590507699854, -2.763914921897999921 ) ) ;
#58253=CARTESIAN_POINT ( 'NONE',  ( 10.48543666025108401, -78.09166666666666856, 6.043427764450814976 ) ) ;
#58254=CARTESIAN_POINT ( 'NONE',  ( -5.246654900278999278, -80.97711506270789528, -9.828008984874001541 ) ) ;
#58266=DIRECTION ( 'NONE',  ( 1.000000000000000000, 0.000000000000000000, 0.000000000000000000 ) ) ;
#58270=CARTESIAN_POINT ( 'NONE',  ( -9.495603837127998048, -78.32176524200400536, -6.055366803880999349 ) ) ;
#58275=DIRECTION ( 'NONE',  ( 0.000000000000000000, -1.000000000000000000, 0.000000000000000000 ) ) ;
#58276=CARTESIAN_POINT ( 'NONE',  ( 2.126420427321150441, -80.24120890908154990, -10.53736461004005953 ) ) ;
#58278=CARTESIAN_POINT ( 'NONE',  ( 3.371482348195443457, -79.49920233275777548, -10.69835107572759902 ) ) ;
#58280=ADVANCED_FACE ( 'NONE', ( #31982 ), #39971, .T. ) ;
#58283=CARTESIAN_POINT ( 'NONE',  ( 2.392795665116000059, -80.24857547445330397, 10.66634390655999987 ) ) ;
#58295=CARTESIAN_POINT ( 'NONE',  ( 6.654794014482000364, -79.31766689940799608, -8.798605060253001042 ) ) ;
#58317=CARTESIAN_POINT ( 'NONE',  ( 12.00000000000000000, -76.54999999999999716, 0.000000000000000000 ) ) ;
#58318=FACE_OUTER_BOUND ( 'NONE', #55905, .T. ) ;
#58321=CARTESIAN_POINT ( 'NONE',  ( 12.00000000000000000, -77.54999999999999716, 0.000000000000000000 ) ) ;
#58322=CARTESIAN_POINT ( 'NONE',  ( 10.07210119001000059, -80.68864150678149372, 5.045985883512999592 ) ) ;
#58327=CYLINDRICAL_SURFACE ( 'NONE', #24188, 12.00000000000000000 ) ;
#58331=VECTOR ( 'NONE', #33968, 1000.000000000000114 ) ;
#58346=CARTESIAN_POINT ( 'NONE',  ( -2.015531751727218435, -77.21013824102965373, -10.56028365160725535 ) ) ;
#58353=CARTESIAN_POINT ( 'NONE',  ( -5.944540622819851627, -76.10208333280840520, -10.31217357874345630 ) ) ;
#58356=CARTESIAN_POINT ( 'NONE',  ( 0.3886576371541999864, -77.31875387357798957, -11.81216847760999933 ) ) ;
#58362=CARTESIAN_POINT ( 'NONE',  ( -12.00019890019965096, -76.39977373798492977, -1.177339121803222359E-06 ) ) ;
#58364=EDGE_CURVE ( 'NONE', #28435, #27557, #54813, .T. ) ;
#58366=ORIENTED_EDGE ( 'NONE', *, *, #30225, .T. ) ;
#58369=AXIS2_PLACEMENT_3D ( 'NONE', #17563, #51346, #56063 ) ;
#58392=CARTESIAN_POINT ( 'NONE',  ( 7.977342298186999692, -77.83638398095499156, 7.452340293345999456 ) ) ;
#58393=CARTESIAN_POINT ( 'NONE',  ( 1.747513281931999840, -77.07779697871899316, -11.88039736288000014 ) ) ;
#58394=CARTESIAN_POINT ( 'NONE',  ( -9.700000000000001066, -90.29999999999999716, 0.000000000000000000 ) ) ;
#58396=CARTESIAN_POINT ( 'NONE',  ( -8.596418555780431348, -79.05208333333331439, -6.606377239730338857 ) ) ;
#58402=CARTESIAN_POINT ( 'NONE',  ( 1.140106547902999923, -78.99079040463000467, 11.87165445709000089 ) ) ;
#58403=CARTESIAN_POINT ( 'NONE',  ( 11.16260469787999909, -80.88779469070068728, -0.4690387474302000204 ) ) ;
#58406=CARTESIAN_POINT ( 'NONE',  ( 7.199825537761999961, -77.15343348694199221, 8.601198917431998936 ) ) ;
#58407=DIRECTION ( 'NONE',  ( -3.552713678800000476E-14, -1.000000000000000000, -1.110223024625000030E-13 ) ) ;
ENDSEC;
END-ISO-10303-21;
